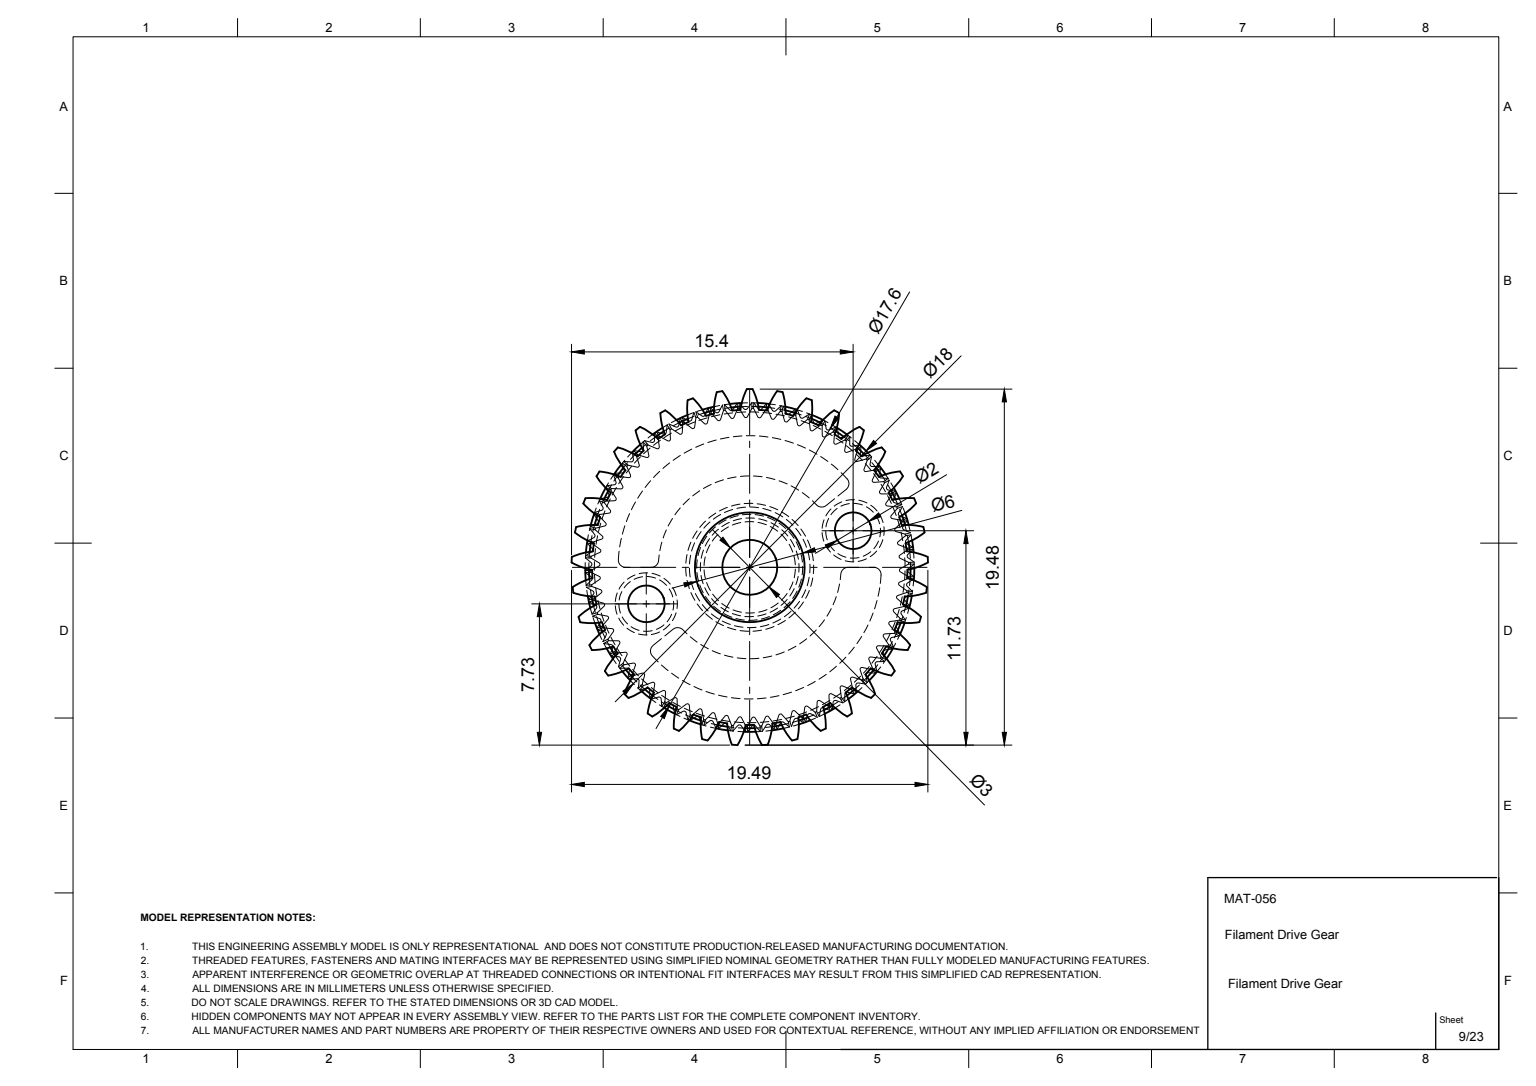
ISO-10303-21;
HEADER;
/* Generated by software containing ST-Developer
 * from STEP Tools, Inc. (www.steptools.com) 
 */

FILE_DESCRIPTION(
/* description */ (''),
/* implementation_level */ '2;1');

FILE_NAME(
/* name */ 'Filament Drive Gear.step',
/* time_stamp */ '2026-10-28T16:47:13+01:00',
/* author */ (''),
/* organization */ (''),
/* preprocessor_version */ 'ST-DEVELOPER v20.2',
/* originating_system */ 'Autodesk Translation Framework v15.17.0.0',
/* authorisation */ '');

FILE_SCHEMA (('AUTOMOTIVE_DESIGN { 1 0 10303 214 3 1 1 }'));
ENDSEC;

DATA;
#10=MECHANICAL_DESIGN_GEOMETRIC_PRESENTATION_REPRESENTATION('',(#4574,#4575),#459242);
#1698=TOROIDAL_SURFACE('',#97244,10.516666667,1.816666667);
#1699=TOROIDAL_SURFACE('',#97247,10.516666667,1.816666667);
#1700=TOROIDAL_SURFACE('',#97250,10.516666667,1.816666667);
#1701=TOROIDAL_SURFACE('',#97253,10.516666667,1.816666667);
#1702=TOROIDAL_SURFACE('',#97256,10.516666667,1.816666667);
#1703=TOROIDAL_SURFACE('',#97259,10.516666667,1.816666667);
#1704=TOROIDAL_SURFACE('',#97262,10.516666667,1.816666667);
#1705=TOROIDAL_SURFACE('',#97265,10.516666667,1.816666667);
#1706=TOROIDAL_SURFACE('',#97268,10.516666667,1.816666667);
#1707=TOROIDAL_SURFACE('',#97271,10.516666667,1.816666667);
#1708=TOROIDAL_SURFACE('',#97274,10.516666667,1.816666667);
#1709=TOROIDAL_SURFACE('',#97277,10.516666667,1.816666667);
#1710=TOROIDAL_SURFACE('',#97280,10.516666667,1.816666667);
#1711=TOROIDAL_SURFACE('',#97283,10.516666667,1.816666667);
#1712=TOROIDAL_SURFACE('',#97286,10.516666667,1.816666667);
#1713=TOROIDAL_SURFACE('',#97289,10.516666667,1.816666667);
#1714=TOROIDAL_SURFACE('',#97292,10.516666667,1.816666667);
#1715=TOROIDAL_SURFACE('',#97295,10.516666667,1.816666667);
#1716=TOROIDAL_SURFACE('',#97298,10.516666667,1.816666667);
#1717=TOROIDAL_SURFACE('',#97301,10.516666667,1.816666667);
#1718=TOROIDAL_SURFACE('',#97304,10.516666667,1.816666667);
#1719=TOROIDAL_SURFACE('',#97307,10.516666667,1.816666667);
#1720=TOROIDAL_SURFACE('',#97310,10.516666667,1.816666667);
#1721=TOROIDAL_SURFACE('',#97313,10.516666667,1.816666667);
#1722=TOROIDAL_SURFACE('',#97316,10.516666667,1.816666667);
#1723=TOROIDAL_SURFACE('',#97319,10.516666667,1.816666667);
#1724=TOROIDAL_SURFACE('',#97322,10.516666667,1.816666667);
#1725=TOROIDAL_SURFACE('',#97325,10.516666667,1.816666667);
#1726=TOROIDAL_SURFACE('',#97328,10.516666667,1.816666667);
#1727=TOROIDAL_SURFACE('',#97331,10.516666667,1.816666667);
#1728=TOROIDAL_SURFACE('',#97334,10.516666667,1.816666667);
#1729=TOROIDAL_SURFACE('',#97337,10.516666667,1.816666667);
#1730=TOROIDAL_SURFACE('',#97340,10.516666667,1.816666667);
#1731=TOROIDAL_SURFACE('',#97343,10.516666667,1.816666667);
#1732=TOROIDAL_SURFACE('',#97346,10.516666667,1.816666667);
#1733=TOROIDAL_SURFACE('',#97349,10.516666667,1.816666667);
#1734=TOROIDAL_SURFACE('',#97352,10.516666667,1.816666667);
#1735=TOROIDAL_SURFACE('',#97355,10.516666667,1.816666667);
#1736=TOROIDAL_SURFACE('',#97358,10.516666667,1.816666667);
#1737=TOROIDAL_SURFACE('',#97361,10.516666667,1.816666667);
#1738=TOROIDAL_SURFACE('',#97364,10.516666667,1.816666667);
#1739=TOROIDAL_SURFACE('',#97367,10.516666667,1.816666667);
#1740=TOROIDAL_SURFACE('',#97370,10.516666667,1.816666667);
#1741=TOROIDAL_SURFACE('',#97373,10.516666667,1.816666667);
#1742=TOROIDAL_SURFACE('',#97376,10.516666667,1.816666667);
#1743=TOROIDAL_SURFACE('',#97379,10.516666667,1.816666667);
#1744=TOROIDAL_SURFACE('',#97382,10.516666667,1.816666667);
#1745=TOROIDAL_SURFACE('',#97385,10.516666667,1.816666667);
#1746=TOROIDAL_SURFACE('',#97388,10.516666667,1.816666667);
#1747=TOROIDAL_SURFACE('',#97391,10.516666667,1.816666667);
#1748=TOROIDAL_SURFACE('',#97394,10.516666667,1.816666667);
#1749=TOROIDAL_SURFACE('',#97397,10.516666667,1.816666667);
#1750=TOROIDAL_SURFACE('',#97400,10.516666667,1.816666667);
#1751=TOROIDAL_SURFACE('',#97403,10.516666667,1.816666667);
#1752=TOROIDAL_SURFACE('',#97406,10.516666667,1.816666667);
#1753=TOROIDAL_SURFACE('',#97409,10.516666667,1.816666667);
#1754=TOROIDAL_SURFACE('',#97412,10.516666667,1.816666667);
#1755=TOROIDAL_SURFACE('',#97415,10.516666667,1.816666667);
#1756=TOROIDAL_SURFACE('',#97418,10.516666667,1.816666667);
#1757=TOROIDAL_SURFACE('',#97421,10.516666667,1.816666667);
#1758=TOROIDAL_SURFACE('',#97424,10.516666667,1.816666667);
#1759=TOROIDAL_SURFACE('',#97427,10.516666667,1.816666667);
#1760=TOROIDAL_SURFACE('',#97430,10.516666667,1.816666667);
#1761=TOROIDAL_SURFACE('',#97433,10.516666667,1.816666667);
#1762=TOROIDAL_SURFACE('',#97436,10.516666667,1.816666667);
#1763=TOROIDAL_SURFACE('',#97439,10.516666667,1.816666667);
#1764=TOROIDAL_SURFACE('',#97442,10.516666667,1.816666667);
#1765=TOROIDAL_SURFACE('',#97445,10.516666667,1.816666667);
#1766=TOROIDAL_SURFACE('',#97448,10.516666667,1.816666667);
#1767=TOROIDAL_SURFACE('',#97451,10.516666667,1.816666667);
#1768=TOROIDAL_SURFACE('',#97496,2.222884449,0.1);
#1769=TOROIDAL_SURFACE('',#97501,2.222884449,0.1);
#1770=TOROIDAL_SURFACE('',#97506,2.222884449,0.1);
#1771=TOROIDAL_SURFACE('',#97511,2.222884449,0.1);
#1772=TOROIDAL_SURFACE('',#97516,2.222884449,0.1);
#1773=TOROIDAL_SURFACE('',#97521,2.222884449,0.1);
#1774=TOROIDAL_SURFACE('',#97526,2.222884449,0.1);
#1775=TOROIDAL_SURFACE('',#97531,2.222884449,0.1);
#1776=TOROIDAL_SURFACE('',#97536,2.222884449,0.1);
#1777=TOROIDAL_SURFACE('',#97541,2.222884449,0.1);
#1778=TOROIDAL_SURFACE('',#97546,2.222884449,0.1);
#1779=TOROIDAL_SURFACE('',#97551,2.222884449,0.1);
#1780=TOROIDAL_SURFACE('',#97556,2.222884449,0.1);
#1781=TOROIDAL_SURFACE('',#97561,2.222884449,0.1);
#1782=TOROIDAL_SURFACE('',#97566,2.222884449,0.1);
#1783=TOROIDAL_SURFACE('',#97571,2.222884449,0.1);
#1784=TOROIDAL_SURFACE('',#97576,2.222884449,0.1);
#1785=TOROIDAL_SURFACE('',#97581,2.222884449,0.1);
#1786=TOROIDAL_SURFACE('',#97586,2.222884449,0.1);
#1787=TOROIDAL_SURFACE('',#97591,2.222884449,0.1);
#1788=TOROIDAL_SURFACE('',#97596,2.222884449,0.1);
#1789=TOROIDAL_SURFACE('',#97601,2.222884449,0.1);
#1790=TOROIDAL_SURFACE('',#97606,2.222884449,0.1);
#1791=TOROIDAL_SURFACE('',#97611,2.222884449,0.1);
#1792=TOROIDAL_SURFACE('',#97616,2.222884449,0.1);
#1793=TOROIDAL_SURFACE('',#97621,2.222884449,0.1);
#1794=TOROIDAL_SURFACE('',#97626,2.222884449,0.1);
#1795=TOROIDAL_SURFACE('',#97631,2.222884449,0.1);
#1796=TOROIDAL_SURFACE('',#97636,2.222884449,0.1);
#1797=TOROIDAL_SURFACE('',#97641,2.222884449,0.1);
#1798=TOROIDAL_SURFACE('',#97646,2.222884449,0.1);
#1799=TOROIDAL_SURFACE('',#97651,2.222884449,0.1);
#1800=TOROIDAL_SURFACE('',#97656,2.222884449,0.1);
#1801=TOROIDAL_SURFACE('',#97661,2.222884449,0.1);
#1802=TOROIDAL_SURFACE('',#97666,2.222884449,0.1);
#1803=TOROIDAL_SURFACE('',#97671,2.222884449,0.1);
#1804=TOROIDAL_SURFACE('',#97676,2.222884449,0.1);
#1805=TOROIDAL_SURFACE('',#97681,2.222884449,0.1);
#1806=TOROIDAL_SURFACE('',#97686,2.222884449,0.1);
#1807=TOROIDAL_SURFACE('',#97691,2.222884449,0.1);
#1808=TOROIDAL_SURFACE('',#97696,2.222884449,0.1);
#1809=TOROIDAL_SURFACE('',#97701,2.222884449,0.1);
#1810=TOROIDAL_SURFACE('',#97706,2.222884449,0.1);
#1811=TOROIDAL_SURFACE('',#97711,2.222884449,0.1);
#1812=TOROIDAL_SURFACE('',#97716,2.222884449,0.1);
#1813=TOROIDAL_SURFACE('',#97721,2.222884449,0.1);
#1814=TOROIDAL_SURFACE('',#97726,2.222884449,0.1);
#1815=TOROIDAL_SURFACE('',#97731,2.222884449,0.1);
#1816=TOROIDAL_SURFACE('',#97736,2.222884449,0.1);
#1817=TOROIDAL_SURFACE('',#97741,2.222884449,0.1);
#1818=TOROIDAL_SURFACE('',#97746,2.222884449,0.1);
#1819=TOROIDAL_SURFACE('',#97751,2.222884449,0.1);
#1820=TOROIDAL_SURFACE('',#97756,2.222884449,0.1);
#1821=TOROIDAL_SURFACE('',#97761,2.222884449,0.1);
#1822=TOROIDAL_SURFACE('',#97766,2.222884449,0.1);
#1823=TOROIDAL_SURFACE('',#97771,2.222884449,0.1);
#1824=TOROIDAL_SURFACE('',#97776,2.222884449,0.1);
#1825=TOROIDAL_SURFACE('',#97781,2.222884449,0.1);
#1826=TOROIDAL_SURFACE('',#97786,2.222884449,0.1);
#1827=TOROIDAL_SURFACE('',#97791,2.222884449,0.1);
#1828=TOROIDAL_SURFACE('',#97796,2.222884449,0.1);
#1829=TOROIDAL_SURFACE('',#97801,2.222884449,0.1);
#1830=TOROIDAL_SURFACE('',#97806,2.222884449,0.1);
#1831=TOROIDAL_SURFACE('',#97811,2.222884449,0.1);
#1832=TOROIDAL_SURFACE('',#97816,2.222884449,0.1);
#1833=TOROIDAL_SURFACE('',#97821,2.222884449,0.1);
#1834=TOROIDAL_SURFACE('',#97826,2.222884449,0.1);
#1835=TOROIDAL_SURFACE('',#97831,2.222884449,0.1);
#1836=TOROIDAL_SURFACE('',#97836,2.222884449,0.1);
#1837=TOROIDAL_SURFACE('',#97841,2.222884449,0.1);
#1838=TOROIDAL_SURFACE('',#97850,1.6,0.1);
#1839=TOROIDAL_SURFACE('',#97854,1.6,0.1);
#1840=TOROIDAL_SURFACE('',#97858,1.7,0.2);
#1841=TOROIDAL_SURFACE('',#97863,1.7,0.2);
#1842=TOROIDAL_SURFACE('',#97867,2.8,0.2);
#1843=TOROIDAL_SURFACE('',#97872,0.6,0.2);
#1844=TOROIDAL_SURFACE('',#97877,0.6,0.2);
#1845=TOROIDAL_SURFACE('',#97882,3.9,0.4);
#1846=TOROIDAL_SURFACE('',#97887,1.1,0.4);
#1847=TOROIDAL_SURFACE('',#97892,1.1,0.4);
#1848=TOROIDAL_SURFACE('',#98404,0.6,0.2);
#1849=TOROIDAL_SURFACE('',#98409,7.4,0.2);
#1850=TOROIDAL_SURFACE('',#98410,0.6,0.2);
#1851=TOROIDAL_SURFACE('',#98412,4.8,0.2);
#1852=TOROIDAL_SURFACE('',#98416,0.6,0.2);
#1853=TOROIDAL_SURFACE('',#98417,0.6,0.2);
#1854=TOROIDAL_SURFACE('',#98420,4.8,0.2);
#1855=TOROIDAL_SURFACE('',#98423,0.6,0.2);
#1856=TOROIDAL_SURFACE('',#98427,7.4,0.2);
#1857=TOROIDAL_SURFACE('',#98429,0.6,0.2);
#4411=SHAPE_REPRESENTATION_RELATIONSHIP('SRR','None',#459336,#4432);
#4432=ADVANCED_BREP_SHAPE_REPRESENTATION('',(#4454,#4455),#459225);
#4454=MANIFOLD_SOLID_BREP('Feed gear',#94632);
#4455=MANIFOLD_SOLID_BREP('Drive gear',#94633);
#4574=STYLED_ITEM('',(#459512),#4454);
#4575=STYLED_ITEM('',(#459512),#4455);
#4712=CONICAL_SURFACE('',#97454,2.9,0.78539816250733);
#4713=CONICAL_SURFACE('',#97458,1.5,0.78539816250733);
#4714=CONICAL_SURFACE('',#97462,1.5,0.78539816250733);
#4715=CONICAL_SURFACE('',#97466,8.8,0.78539816250733);
#4716=CONICAL_SURFACE('',#97470,1.7,0.78539816250733);
#4717=CONICAL_SURFACE('',#97473,1.7,0.78539816250733);
#4718=CONICAL_SURFACE('',#97476,3.3,0.78539816250733);
#4719=CONICAL_SURFACE('',#97480,2.5,0.78539816250733);
#4720=CONICAL_SURFACE('',#97485,9.,0.78539816250733);
#4721=CONICAL_SURFACE('',#97494,2.272884449,1.04719754999232);
#4722=CONICAL_SURFACE('',#97498,1.816666667,1.04719754999232);
#4723=CONICAL_SURFACE('',#97499,2.272884449,1.04719754999232);
#4724=CONICAL_SURFACE('',#97503,1.816666667,1.04719754999232);
#4725=CONICAL_SURFACE('',#97504,2.272884449,1.04719754999232);
#4726=CONICAL_SURFACE('',#97508,1.816666667,1.04719754999232);
#4727=CONICAL_SURFACE('',#97509,2.272884449,1.04719754999232);
#4728=CONICAL_SURFACE('',#97513,1.816666667,1.04719754999232);
#4729=CONICAL_SURFACE('',#97514,2.272884449,1.04719754999232);
#4730=CONICAL_SURFACE('',#97518,1.816666667,1.04719754999232);
#4731=CONICAL_SURFACE('',#97519,2.272884449,1.04719754999232);
#4732=CONICAL_SURFACE('',#97523,1.816666667,1.04719754999232);
#4733=CONICAL_SURFACE('',#97524,2.272884449,1.04719754999232);
#4734=CONICAL_SURFACE('',#97528,1.816666667,1.04719754999232);
#4735=CONICAL_SURFACE('',#97529,2.272884449,1.04719754999232);
#4736=CONICAL_SURFACE('',#97533,1.816666667,1.04719754999232);
#4737=CONICAL_SURFACE('',#97534,2.272884449,1.04719754999232);
#4738=CONICAL_SURFACE('',#97538,1.816666667,1.04719754999232);
#4739=CONICAL_SURFACE('',#97539,2.272884449,1.04719754999232);
#4740=CONICAL_SURFACE('',#97543,1.816666667,1.04719754999232);
#4741=CONICAL_SURFACE('',#97544,2.272884449,1.04719754999232);
#4742=CONICAL_SURFACE('',#97548,1.816666667,1.04719754999232);
#4743=CONICAL_SURFACE('',#97549,2.272884449,1.04719754999232);
#4744=CONICAL_SURFACE('',#97553,1.816666667,1.04719754999232);
#4745=CONICAL_SURFACE('',#97554,2.272884449,1.04719754999232);
#4746=CONICAL_SURFACE('',#97558,1.816666667,1.04719754999232);
#4747=CONICAL_SURFACE('',#97559,2.272884449,1.04719754999232);
#4748=CONICAL_SURFACE('',#97563,1.816666667,1.04719754999232);
#4749=CONICAL_SURFACE('',#97564,2.272884449,1.04719754999232);
#4750=CONICAL_SURFACE('',#97568,1.816666667,1.04719754999232);
#4751=CONICAL_SURFACE('',#97569,2.272884449,1.04719754999232);
#4752=CONICAL_SURFACE('',#97573,1.816666667,1.04719754999232);
#4753=CONICAL_SURFACE('',#97574,2.272884449,1.04719754999232);
#4754=CONICAL_SURFACE('',#97578,1.816666667,1.04719754999232);
#4755=CONICAL_SURFACE('',#97579,2.272884449,1.04719754999232);
#4756=CONICAL_SURFACE('',#97583,1.816666667,1.04719754999232);
#4757=CONICAL_SURFACE('',#97584,2.272884449,1.04719754999232);
#4758=CONICAL_SURFACE('',#97588,1.816666667,1.04719754999232);
#4759=CONICAL_SURFACE('',#97589,2.272884449,1.04719754999232);
#4760=CONICAL_SURFACE('',#97593,1.816666667,1.04719754999232);
#4761=CONICAL_SURFACE('',#97594,2.272884449,1.04719754999232);
#4762=CONICAL_SURFACE('',#97598,1.816666667,1.04719754999232);
#4763=CONICAL_SURFACE('',#97599,2.272884449,1.04719754999232);
#4764=CONICAL_SURFACE('',#97603,1.816666667,1.04719754999232);
#4765=CONICAL_SURFACE('',#97604,2.272884449,1.04719754999232);
#4766=CONICAL_SURFACE('',#97608,1.816666667,1.04719754999232);
#4767=CONICAL_SURFACE('',#97609,2.272884449,1.04719754999232);
#4768=CONICAL_SURFACE('',#97613,1.816666667,1.04719754999232);
#4769=CONICAL_SURFACE('',#97614,2.272884449,1.04719754999232);
#4770=CONICAL_SURFACE('',#97618,1.816666667,1.04719754999232);
#4771=CONICAL_SURFACE('',#97619,2.272884449,1.04719754999232);
#4772=CONICAL_SURFACE('',#97623,1.816666667,1.04719754999232);
#4773=CONICAL_SURFACE('',#97624,2.272884449,1.04719754999232);
#4774=CONICAL_SURFACE('',#97628,1.816666667,1.04719754999232);
#4775=CONICAL_SURFACE('',#97629,2.272884449,1.04719754999232);
#4776=CONICAL_SURFACE('',#97633,1.816666667,1.04719754999232);
#4777=CONICAL_SURFACE('',#97634,2.272884449,1.04719754999232);
#4778=CONICAL_SURFACE('',#97638,1.816666667,1.04719754999232);
#4779=CONICAL_SURFACE('',#97639,2.272884449,1.04719754999232);
#4780=CONICAL_SURFACE('',#97643,1.816666667,1.04719754999232);
#4781=CONICAL_SURFACE('',#97644,2.272884449,1.04719754999232);
#4782=CONICAL_SURFACE('',#97648,1.816666667,1.04719754999232);
#4783=CONICAL_SURFACE('',#97649,2.272884449,1.04719754999232);
#4784=CONICAL_SURFACE('',#97653,1.816666667,1.04719754999232);
#4785=CONICAL_SURFACE('',#97654,2.272884449,1.04719754999232);
#4786=CONICAL_SURFACE('',#97658,1.816666667,1.04719754999232);
#4787=CONICAL_SURFACE('',#97659,2.272884449,1.04719754999232);
#4788=CONICAL_SURFACE('',#97663,1.816666667,1.04719754999232);
#4789=CONICAL_SURFACE('',#97664,2.272884449,1.04719754999232);
#4790=CONICAL_SURFACE('',#97668,1.816666667,1.04719754999232);
#4791=CONICAL_SURFACE('',#97669,2.272884449,1.04719754999232);
#4792=CONICAL_SURFACE('',#97673,1.816666667,1.04719754999232);
#4793=CONICAL_SURFACE('',#97674,2.272884449,1.04719754999232);
#4794=CONICAL_SURFACE('',#97678,1.816666667,1.04719754999232);
#4795=CONICAL_SURFACE('',#97679,2.272884449,1.04719754999232);
#4796=CONICAL_SURFACE('',#97683,1.816666667,1.04719754999232);
#4797=CONICAL_SURFACE('',#97684,2.272884449,1.04719754999232);
#4798=CONICAL_SURFACE('',#97688,1.816666667,1.04719754999232);
#4799=CONICAL_SURFACE('',#97689,2.272884449,1.04719754999232);
#4800=CONICAL_SURFACE('',#97693,1.816666667,1.04719754999232);
#4801=CONICAL_SURFACE('',#97694,2.272884449,1.04719754999232);
#4802=CONICAL_SURFACE('',#97698,1.816666667,1.04719754999232);
#4803=CONICAL_SURFACE('',#97699,2.272884449,1.04719754999232);
#4804=CONICAL_SURFACE('',#97703,1.816666667,1.04719754999232);
#4805=CONICAL_SURFACE('',#97704,2.272884449,1.04719754999232);
#4806=CONICAL_SURFACE('',#97708,1.816666667,1.04719754999232);
#4807=CONICAL_SURFACE('',#97709,2.272884449,1.04719754999232);
#4808=CONICAL_SURFACE('',#97713,1.816666667,1.04719754999232);
#4809=CONICAL_SURFACE('',#97714,2.272884449,1.04719754999232);
#4810=CONICAL_SURFACE('',#97718,1.816666667,1.04719754999232);
#4811=CONICAL_SURFACE('',#97719,2.272884449,1.04719754999232);
#4812=CONICAL_SURFACE('',#97723,1.816666667,1.04719754999232);
#4813=CONICAL_SURFACE('',#97724,2.272884449,1.04719754999232);
#4814=CONICAL_SURFACE('',#97728,1.816666667,1.04719754999232);
#4815=CONICAL_SURFACE('',#97729,2.272884449,1.04719754999232);
#4816=CONICAL_SURFACE('',#97733,1.816666667,1.04719754999232);
#4817=CONICAL_SURFACE('',#97734,2.272884449,1.04719754999232);
#4818=CONICAL_SURFACE('',#97738,1.816666667,1.04719754999232);
#4819=CONICAL_SURFACE('',#97739,2.272884449,1.04719754999232);
#4820=CONICAL_SURFACE('',#97743,1.816666667,1.04719754999232);
#4821=CONICAL_SURFACE('',#97744,2.272884449,1.04719754999232);
#4822=CONICAL_SURFACE('',#97748,1.816666667,1.04719754999232);
#4823=CONICAL_SURFACE('',#97749,2.272884449,1.04719754999232);
#4824=CONICAL_SURFACE('',#97753,1.816666667,1.04719754999232);
#4825=CONICAL_SURFACE('',#97754,2.272884449,1.04719754999232);
#4826=CONICAL_SURFACE('',#97758,1.816666667,1.04719754999232);
#4827=CONICAL_SURFACE('',#97759,2.272884449,1.04719754999232);
#4828=CONICAL_SURFACE('',#97763,1.816666667,1.04719754999232);
#4829=CONICAL_SURFACE('',#97764,2.272884449,1.04719754999232);
#4830=CONICAL_SURFACE('',#97768,1.816666667,1.04719754999232);
#4831=CONICAL_SURFACE('',#97769,2.272884449,1.04719754999232);
#4832=CONICAL_SURFACE('',#97773,1.816666667,1.04719754999232);
#4833=CONICAL_SURFACE('',#97774,2.272884449,1.04719754999232);
#4834=CONICAL_SURFACE('',#97778,1.816666667,1.04719754999232);
#4835=CONICAL_SURFACE('',#97779,2.272884449,1.04719754999232);
#4836=CONICAL_SURFACE('',#97783,1.816666667,1.04719754999232);
#4837=CONICAL_SURFACE('',#97784,2.272884449,1.04719754999232);
#4838=CONICAL_SURFACE('',#97788,1.816666667,1.04719754999232);
#4839=CONICAL_SURFACE('',#97789,2.272884449,1.04719754999232);
#4840=CONICAL_SURFACE('',#97793,1.816666667,1.04719754999232);
#4841=CONICAL_SURFACE('',#97794,2.272884449,1.04719754999232);
#4842=CONICAL_SURFACE('',#97798,1.816666667,1.04719754999232);
#4843=CONICAL_SURFACE('',#97799,2.272884449,1.04719754999232);
#4844=CONICAL_SURFACE('',#97803,1.816666667,1.04719754999232);
#4845=CONICAL_SURFACE('',#97804,2.272884449,1.04719754999232);
#4846=CONICAL_SURFACE('',#97808,1.816666667,1.04719754999232);
#4847=CONICAL_SURFACE('',#97809,2.272884449,1.04719754999232);
#4848=CONICAL_SURFACE('',#97813,1.816666667,1.04719754999232);
#4849=CONICAL_SURFACE('',#97814,2.272884449,1.04719754999232);
#4850=CONICAL_SURFACE('',#97818,1.816666667,1.04719754999232);
#4851=CONICAL_SURFACE('',#97819,2.272884449,1.04719754999232);
#4852=CONICAL_SURFACE('',#97823,1.816666667,1.04719754999232);
#4853=CONICAL_SURFACE('',#97824,2.272884449,1.04719754999232);
#4854=CONICAL_SURFACE('',#97828,1.816666667,1.04719754999232);
#4855=CONICAL_SURFACE('',#97829,2.272884449,1.04719754999232);
#4856=CONICAL_SURFACE('',#97833,1.816666667,1.04719754999232);
#4857=CONICAL_SURFACE('',#97834,2.272884449,1.04719754999232);
#4858=CONICAL_SURFACE('',#97838,1.816666667,1.04719754999232);
#4859=CONICAL_SURFACE('',#97839,2.272884449,1.04719754999232);
#4860=CONICAL_SURFACE('',#97843,1.816666667,1.04719754999232);
#5170=FACE_BOUND('',#13390,.T.);
#5171=FACE_BOUND('',#13392,.T.);
#5172=FACE_BOUND('',#13393,.T.);
#5173=FACE_BOUND('',#13394,.T.);
#5174=FACE_BOUND('',#13396,.T.);
#5175=FACE_BOUND('',#13397,.T.);
#5176=FACE_BOUND('',#13398,.T.);
#5177=FACE_BOUND('',#13633,.T.);
#5178=FACE_BOUND('',#13634,.T.);
#5179=FACE_BOUND('',#13635,.T.);
#5180=FACE_BOUND('',#13636,.T.);
#5181=FACE_BOUND('',#13637,.T.);
#5182=FACE_BOUND('',#13675,.T.);
#5183=FACE_BOUND('',#13676,.T.);
#5184=FACE_BOUND('',#13677,.T.);
#5185=FACE_BOUND('',#13787,.T.);
#5186=FACE_BOUND('',#13791,.T.);
#5591=PLANE('',#97491);
#5592=PLANE('',#97492);
#5593=PLANE('',#97493);
#5594=PLANE('',#97922);
#5595=PLANE('',#98149);
#5596=PLANE('',#98366);
#5597=PLANE('',#98367);
#5598=PLANE('',#98368);
#5599=PLANE('',#98369);
#5600=PLANE('',#98370);
#5601=PLANE('',#98380);
#5602=PLANE('',#98386);
#5603=PLANE('',#98390);
#5604=PLANE('',#98396);
#5605=PLANE('',#98403);
#5606=PLANE('',#98430);
#5607=PLANE('',#98431);
#7440=FACE_OUTER_BOUND('',#13305,.T.);
#7441=FACE_OUTER_BOUND('',#13306,.T.);
#7442=FACE_OUTER_BOUND('',#13307,.T.);
#7443=FACE_OUTER_BOUND('',#13308,.T.);
#7444=FACE_OUTER_BOUND('',#13309,.T.);
#7445=FACE_OUTER_BOUND('',#13310,.T.);
#7446=FACE_OUTER_BOUND('',#13311,.T.);
#7447=FACE_OUTER_BOUND('',#13312,.T.);
#7448=FACE_OUTER_BOUND('',#13313,.T.);
#7449=FACE_OUTER_BOUND('',#13314,.T.);
#7450=FACE_OUTER_BOUND('',#13315,.T.);
#7451=FACE_OUTER_BOUND('',#13316,.T.);
#7452=FACE_OUTER_BOUND('',#13317,.T.);
#7453=FACE_OUTER_BOUND('',#13318,.T.);
#7454=FACE_OUTER_BOUND('',#13319,.T.);
#7455=FACE_OUTER_BOUND('',#13320,.T.);
#7456=FACE_OUTER_BOUND('',#13321,.T.);
#7457=FACE_OUTER_BOUND('',#13322,.T.);
#7458=FACE_OUTER_BOUND('',#13323,.T.);
#7459=FACE_OUTER_BOUND('',#13324,.T.);
#7460=FACE_OUTER_BOUND('',#13325,.T.);
#7461=FACE_OUTER_BOUND('',#13326,.T.);
#7462=FACE_OUTER_BOUND('',#13327,.T.);
#7463=FACE_OUTER_BOUND('',#13328,.T.);
#7464=FACE_OUTER_BOUND('',#13329,.T.);
#7465=FACE_OUTER_BOUND('',#13330,.T.);
#7466=FACE_OUTER_BOUND('',#13331,.T.);
#7467=FACE_OUTER_BOUND('',#13332,.T.);
#7468=FACE_OUTER_BOUND('',#13333,.T.);
#7469=FACE_OUTER_BOUND('',#13334,.T.);
#7470=FACE_OUTER_BOUND('',#13335,.T.);
#7471=FACE_OUTER_BOUND('',#13336,.T.);
#7472=FACE_OUTER_BOUND('',#13337,.T.);
#7473=FACE_OUTER_BOUND('',#13338,.T.);
#7474=FACE_OUTER_BOUND('',#13339,.T.);
#7475=FACE_OUTER_BOUND('',#13340,.T.);
#7476=FACE_OUTER_BOUND('',#13341,.T.);
#7477=FACE_OUTER_BOUND('',#13342,.T.);
#7478=FACE_OUTER_BOUND('',#13343,.T.);
#7479=FACE_OUTER_BOUND('',#13344,.T.);
#7480=FACE_OUTER_BOUND('',#13345,.T.);
#7481=FACE_OUTER_BOUND('',#13346,.T.);
#7482=FACE_OUTER_BOUND('',#13347,.T.);
#7483=FACE_OUTER_BOUND('',#13348,.T.);
#7484=FACE_OUTER_BOUND('',#13349,.T.);
#7485=FACE_OUTER_BOUND('',#13350,.T.);
#7486=FACE_OUTER_BOUND('',#13351,.T.);
#7487=FACE_OUTER_BOUND('',#13352,.T.);
#7488=FACE_OUTER_BOUND('',#13353,.T.);
#7489=FACE_OUTER_BOUND('',#13354,.T.);
#7490=FACE_OUTER_BOUND('',#13355,.T.);
#7491=FACE_OUTER_BOUND('',#13356,.T.);
#7492=FACE_OUTER_BOUND('',#13357,.T.);
#7493=FACE_OUTER_BOUND('',#13358,.T.);
#7494=FACE_OUTER_BOUND('',#13359,.T.);
#7495=FACE_OUTER_BOUND('',#13360,.T.);
#7496=FACE_OUTER_BOUND('',#13361,.T.);
#7497=FACE_OUTER_BOUND('',#13362,.T.);
#7498=FACE_OUTER_BOUND('',#13363,.T.);
#7499=FACE_OUTER_BOUND('',#13364,.T.);
#7500=FACE_OUTER_BOUND('',#13365,.T.);
#7501=FACE_OUTER_BOUND('',#13366,.T.);
#7502=FACE_OUTER_BOUND('',#13367,.T.);
#7503=FACE_OUTER_BOUND('',#13368,.T.);
#7504=FACE_OUTER_BOUND('',#13369,.T.);
#7505=FACE_OUTER_BOUND('',#13370,.T.);
#7506=FACE_OUTER_BOUND('',#13371,.T.);
#7507=FACE_OUTER_BOUND('',#13372,.T.);
#7508=FACE_OUTER_BOUND('',#13373,.T.);
#7509=FACE_OUTER_BOUND('',#13374,.T.);
#7510=FACE_OUTER_BOUND('',#13375,.T.);
#7511=FACE_OUTER_BOUND('',#13376,.T.);
#7512=FACE_OUTER_BOUND('',#13377,.T.);
#7513=FACE_OUTER_BOUND('',#13378,.T.);
#7514=FACE_OUTER_BOUND('',#13379,.T.);
#7515=FACE_OUTER_BOUND('',#13380,.T.);
#7516=FACE_OUTER_BOUND('',#13381,.T.);
#7517=FACE_OUTER_BOUND('',#13382,.T.);
#7518=FACE_OUTER_BOUND('',#13383,.T.);
#7519=FACE_OUTER_BOUND('',#13384,.T.);
#7520=FACE_OUTER_BOUND('',#13385,.T.);
#7521=FACE_OUTER_BOUND('',#13386,.T.);
#7522=FACE_OUTER_BOUND('',#13387,.T.);
#7523=FACE_OUTER_BOUND('',#13388,.T.);
#7524=FACE_OUTER_BOUND('',#13389,.T.);
#7525=FACE_OUTER_BOUND('',#13391,.T.);
#7526=FACE_OUTER_BOUND('',#13395,.T.);
#7527=FACE_OUTER_BOUND('',#13399,.T.);
#7528=FACE_OUTER_BOUND('',#13400,.T.);
#7529=FACE_OUTER_BOUND('',#13401,.T.);
#7530=FACE_OUTER_BOUND('',#13402,.T.);
#7531=FACE_OUTER_BOUND('',#13403,.T.);
#7532=FACE_OUTER_BOUND('',#13404,.T.);
#7533=FACE_OUTER_BOUND('',#13405,.T.);
#7534=FACE_OUTER_BOUND('',#13406,.T.);
#7535=FACE_OUTER_BOUND('',#13407,.T.);
#7536=FACE_OUTER_BOUND('',#13408,.T.);
#7537=FACE_OUTER_BOUND('',#13409,.T.);
#7538=FACE_OUTER_BOUND('',#13410,.T.);
#7539=FACE_OUTER_BOUND('',#13411,.T.);
#7540=FACE_OUTER_BOUND('',#13412,.T.);
#7541=FACE_OUTER_BOUND('',#13413,.T.);
#7542=FACE_OUTER_BOUND('',#13414,.T.);
#7543=FACE_OUTER_BOUND('',#13415,.T.);
#7544=FACE_OUTER_BOUND('',#13416,.T.);
#7545=FACE_OUTER_BOUND('',#13417,.T.);
#7546=FACE_OUTER_BOUND('',#13418,.T.);
#7547=FACE_OUTER_BOUND('',#13419,.T.);
#7548=FACE_OUTER_BOUND('',#13420,.T.);
#7549=FACE_OUTER_BOUND('',#13421,.T.);
#7550=FACE_OUTER_BOUND('',#13422,.T.);
#7551=FACE_OUTER_BOUND('',#13423,.T.);
#7552=FACE_OUTER_BOUND('',#13424,.T.);
#7553=FACE_OUTER_BOUND('',#13425,.T.);
#7554=FACE_OUTER_BOUND('',#13426,.T.);
#7555=FACE_OUTER_BOUND('',#13427,.T.);
#7556=FACE_OUTER_BOUND('',#13428,.T.);
#7557=FACE_OUTER_BOUND('',#13429,.T.);
#7558=FACE_OUTER_BOUND('',#13430,.T.);
#7559=FACE_OUTER_BOUND('',#13431,.T.);
#7560=FACE_OUTER_BOUND('',#13432,.T.);
#7561=FACE_OUTER_BOUND('',#13433,.T.);
#7562=FACE_OUTER_BOUND('',#13434,.T.);
#7563=FACE_OUTER_BOUND('',#13435,.T.);
#7564=FACE_OUTER_BOUND('',#13436,.T.);
#7565=FACE_OUTER_BOUND('',#13437,.T.);
#7566=FACE_OUTER_BOUND('',#13438,.T.);
#7567=FACE_OUTER_BOUND('',#13439,.T.);
#7568=FACE_OUTER_BOUND('',#13440,.T.);
#7569=FACE_OUTER_BOUND('',#13441,.T.);
#7570=FACE_OUTER_BOUND('',#13442,.T.);
#7571=FACE_OUTER_BOUND('',#13443,.T.);
#7572=FACE_OUTER_BOUND('',#13444,.T.);
#7573=FACE_OUTER_BOUND('',#13445,.T.);
#7574=FACE_OUTER_BOUND('',#13446,.T.);
#7575=FACE_OUTER_BOUND('',#13447,.T.);
#7576=FACE_OUTER_BOUND('',#13448,.T.);
#7577=FACE_OUTER_BOUND('',#13449,.T.);
#7578=FACE_OUTER_BOUND('',#13450,.T.);
#7579=FACE_OUTER_BOUND('',#13451,.T.);
#7580=FACE_OUTER_BOUND('',#13452,.T.);
#7581=FACE_OUTER_BOUND('',#13453,.T.);
#7582=FACE_OUTER_BOUND('',#13454,.T.);
#7583=FACE_OUTER_BOUND('',#13455,.T.);
#7584=FACE_OUTER_BOUND('',#13456,.T.);
#7585=FACE_OUTER_BOUND('',#13457,.T.);
#7586=FACE_OUTER_BOUND('',#13458,.T.);
#7587=FACE_OUTER_BOUND('',#13459,.T.);
#7588=FACE_OUTER_BOUND('',#13460,.T.);
#7589=FACE_OUTER_BOUND('',#13461,.T.);
#7590=FACE_OUTER_BOUND('',#13462,.T.);
#7591=FACE_OUTER_BOUND('',#13463,.T.);
#7592=FACE_OUTER_BOUND('',#13464,.T.);
#7593=FACE_OUTER_BOUND('',#13465,.T.);
#7594=FACE_OUTER_BOUND('',#13466,.T.);
#7595=FACE_OUTER_BOUND('',#13467,.T.);
#7596=FACE_OUTER_BOUND('',#13468,.T.);
#7597=FACE_OUTER_BOUND('',#13469,.T.);
#7598=FACE_OUTER_BOUND('',#13470,.T.);
#7599=FACE_OUTER_BOUND('',#13471,.T.);
#7600=FACE_OUTER_BOUND('',#13472,.T.);
#7601=FACE_OUTER_BOUND('',#13473,.T.);
#7602=FACE_OUTER_BOUND('',#13474,.T.);
#7603=FACE_OUTER_BOUND('',#13475,.T.);
#7604=FACE_OUTER_BOUND('',#13476,.T.);
#7605=FACE_OUTER_BOUND('',#13477,.T.);
#7606=FACE_OUTER_BOUND('',#13478,.T.);
#7607=FACE_OUTER_BOUND('',#13479,.T.);
#7608=FACE_OUTER_BOUND('',#13480,.T.);
#7609=FACE_OUTER_BOUND('',#13481,.T.);
#7610=FACE_OUTER_BOUND('',#13482,.T.);
#7611=FACE_OUTER_BOUND('',#13483,.T.);
#7612=FACE_OUTER_BOUND('',#13484,.T.);
#7613=FACE_OUTER_BOUND('',#13485,.T.);
#7614=FACE_OUTER_BOUND('',#13486,.T.);
#7615=FACE_OUTER_BOUND('',#13487,.T.);
#7616=FACE_OUTER_BOUND('',#13488,.T.);
#7617=FACE_OUTER_BOUND('',#13489,.T.);
#7618=FACE_OUTER_BOUND('',#13490,.T.);
#7619=FACE_OUTER_BOUND('',#13491,.T.);
#7620=FACE_OUTER_BOUND('',#13492,.T.);
#7621=FACE_OUTER_BOUND('',#13493,.T.);
#7622=FACE_OUTER_BOUND('',#13494,.T.);
#7623=FACE_OUTER_BOUND('',#13495,.T.);
#7624=FACE_OUTER_BOUND('',#13496,.T.);
#7625=FACE_OUTER_BOUND('',#13497,.T.);
#7626=FACE_OUTER_BOUND('',#13498,.T.);
#7627=FACE_OUTER_BOUND('',#13499,.T.);
#7628=FACE_OUTER_BOUND('',#13500,.T.);
#7629=FACE_OUTER_BOUND('',#13501,.T.);
#7630=FACE_OUTER_BOUND('',#13502,.T.);
#7631=FACE_OUTER_BOUND('',#13503,.T.);
#7632=FACE_OUTER_BOUND('',#13504,.T.);
#7633=FACE_OUTER_BOUND('',#13505,.T.);
#7634=FACE_OUTER_BOUND('',#13506,.T.);
#7635=FACE_OUTER_BOUND('',#13507,.T.);
#7636=FACE_OUTER_BOUND('',#13508,.T.);
#7637=FACE_OUTER_BOUND('',#13509,.T.);
#7638=FACE_OUTER_BOUND('',#13510,.T.);
#7639=FACE_OUTER_BOUND('',#13511,.T.);
#7640=FACE_OUTER_BOUND('',#13512,.T.);
#7641=FACE_OUTER_BOUND('',#13513,.T.);
#7642=FACE_OUTER_BOUND('',#13514,.T.);
#7643=FACE_OUTER_BOUND('',#13515,.T.);
#7644=FACE_OUTER_BOUND('',#13516,.T.);
#7645=FACE_OUTER_BOUND('',#13517,.T.);
#7646=FACE_OUTER_BOUND('',#13518,.T.);
#7647=FACE_OUTER_BOUND('',#13519,.T.);
#7648=FACE_OUTER_BOUND('',#13520,.T.);
#7649=FACE_OUTER_BOUND('',#13521,.T.);
#7650=FACE_OUTER_BOUND('',#13522,.T.);
#7651=FACE_OUTER_BOUND('',#13523,.T.);
#7652=FACE_OUTER_BOUND('',#13524,.T.);
#7653=FACE_OUTER_BOUND('',#13525,.T.);
#7654=FACE_OUTER_BOUND('',#13526,.T.);
#7655=FACE_OUTER_BOUND('',#13527,.T.);
#7656=FACE_OUTER_BOUND('',#13528,.T.);
#7657=FACE_OUTER_BOUND('',#13529,.T.);
#7658=FACE_OUTER_BOUND('',#13530,.T.);
#7659=FACE_OUTER_BOUND('',#13531,.T.);
#7660=FACE_OUTER_BOUND('',#13532,.T.);
#7661=FACE_OUTER_BOUND('',#13533,.T.);
#7662=FACE_OUTER_BOUND('',#13534,.T.);
#7663=FACE_OUTER_BOUND('',#13535,.T.);
#7664=FACE_OUTER_BOUND('',#13536,.T.);
#7665=FACE_OUTER_BOUND('',#13537,.T.);
#7666=FACE_OUTER_BOUND('',#13538,.T.);
#7667=FACE_OUTER_BOUND('',#13539,.T.);
#7668=FACE_OUTER_BOUND('',#13540,.T.);
#7669=FACE_OUTER_BOUND('',#13541,.T.);
#7670=FACE_OUTER_BOUND('',#13542,.T.);
#7671=FACE_OUTER_BOUND('',#13543,.T.);
#7672=FACE_OUTER_BOUND('',#13544,.T.);
#7673=FACE_OUTER_BOUND('',#13545,.T.);
#7674=FACE_OUTER_BOUND('',#13546,.T.);
#7675=FACE_OUTER_BOUND('',#13547,.T.);
#7676=FACE_OUTER_BOUND('',#13548,.T.);
#7677=FACE_OUTER_BOUND('',#13549,.T.);
#7678=FACE_OUTER_BOUND('',#13550,.T.);
#7679=FACE_OUTER_BOUND('',#13551,.T.);
#7680=FACE_OUTER_BOUND('',#13552,.T.);
#7681=FACE_OUTER_BOUND('',#13553,.T.);
#7682=FACE_OUTER_BOUND('',#13554,.T.);
#7683=FACE_OUTER_BOUND('',#13555,.T.);
#7684=FACE_OUTER_BOUND('',#13556,.T.);
#7685=FACE_OUTER_BOUND('',#13557,.T.);
#7686=FACE_OUTER_BOUND('',#13558,.T.);
#7687=FACE_OUTER_BOUND('',#13559,.T.);
#7688=FACE_OUTER_BOUND('',#13560,.T.);
#7689=FACE_OUTER_BOUND('',#13561,.T.);
#7690=FACE_OUTER_BOUND('',#13562,.T.);
#7691=FACE_OUTER_BOUND('',#13563,.T.);
#7692=FACE_OUTER_BOUND('',#13564,.T.);
#7693=FACE_OUTER_BOUND('',#13565,.T.);
#7694=FACE_OUTER_BOUND('',#13566,.T.);
#7695=FACE_OUTER_BOUND('',#13567,.T.);
#7696=FACE_OUTER_BOUND('',#13568,.T.);
#7697=FACE_OUTER_BOUND('',#13569,.T.);
#7698=FACE_OUTER_BOUND('',#13570,.T.);
#7699=FACE_OUTER_BOUND('',#13571,.T.);
#7700=FACE_OUTER_BOUND('',#13572,.T.);
#7701=FACE_OUTER_BOUND('',#13573,.T.);
#7702=FACE_OUTER_BOUND('',#13574,.T.);
#7703=FACE_OUTER_BOUND('',#13575,.T.);
#7704=FACE_OUTER_BOUND('',#13576,.T.);
#7705=FACE_OUTER_BOUND('',#13577,.T.);
#7706=FACE_OUTER_BOUND('',#13578,.T.);
#7707=FACE_OUTER_BOUND('',#13579,.T.);
#7708=FACE_OUTER_BOUND('',#13580,.T.);
#7709=FACE_OUTER_BOUND('',#13581,.T.);
#7710=FACE_OUTER_BOUND('',#13582,.T.);
#7711=FACE_OUTER_BOUND('',#13583,.T.);
#7712=FACE_OUTER_BOUND('',#13584,.T.);
#7713=FACE_OUTER_BOUND('',#13585,.T.);
#7714=FACE_OUTER_BOUND('',#13586,.T.);
#7715=FACE_OUTER_BOUND('',#13587,.T.);
#7716=FACE_OUTER_BOUND('',#13588,.T.);
#7717=FACE_OUTER_BOUND('',#13589,.T.);
#7718=FACE_OUTER_BOUND('',#13590,.T.);
#7719=FACE_OUTER_BOUND('',#13591,.T.);
#7720=FACE_OUTER_BOUND('',#13592,.T.);
#7721=FACE_OUTER_BOUND('',#13593,.T.);
#7722=FACE_OUTER_BOUND('',#13594,.T.);
#7723=FACE_OUTER_BOUND('',#13595,.T.);
#7724=FACE_OUTER_BOUND('',#13596,.T.);
#7725=FACE_OUTER_BOUND('',#13597,.T.);
#7726=FACE_OUTER_BOUND('',#13598,.T.);
#7727=FACE_OUTER_BOUND('',#13599,.T.);
#7728=FACE_OUTER_BOUND('',#13600,.T.);
#7729=FACE_OUTER_BOUND('',#13601,.T.);
#7730=FACE_OUTER_BOUND('',#13602,.T.);
#7731=FACE_OUTER_BOUND('',#13603,.T.);
#7732=FACE_OUTER_BOUND('',#13604,.T.);
#7733=FACE_OUTER_BOUND('',#13605,.T.);
#7734=FACE_OUTER_BOUND('',#13606,.T.);
#7735=FACE_OUTER_BOUND('',#13607,.T.);
#7736=FACE_OUTER_BOUND('',#13608,.T.);
#7737=FACE_OUTER_BOUND('',#13609,.T.);
#7738=FACE_OUTER_BOUND('',#13610,.T.);
#7739=FACE_OUTER_BOUND('',#13611,.T.);
#7740=FACE_OUTER_BOUND('',#13612,.T.);
#7741=FACE_OUTER_BOUND('',#13613,.T.);
#7742=FACE_OUTER_BOUND('',#13614,.T.);
#7743=FACE_OUTER_BOUND('',#13615,.T.);
#7744=FACE_OUTER_BOUND('',#13616,.T.);
#7745=FACE_OUTER_BOUND('',#13617,.T.);
#7746=FACE_OUTER_BOUND('',#13618,.T.);
#7747=FACE_OUTER_BOUND('',#13619,.T.);
#7748=FACE_OUTER_BOUND('',#13620,.T.);
#7749=FACE_OUTER_BOUND('',#13621,.T.);
#7750=FACE_OUTER_BOUND('',#13622,.T.);
#7751=FACE_OUTER_BOUND('',#13623,.T.);
#7752=FACE_OUTER_BOUND('',#13624,.T.);
#7753=FACE_OUTER_BOUND('',#13625,.T.);
#7754=FACE_OUTER_BOUND('',#13626,.T.);
#7755=FACE_OUTER_BOUND('',#13627,.T.);
#7756=FACE_OUTER_BOUND('',#13628,.T.);
#7757=FACE_OUTER_BOUND('',#13629,.T.);
#7758=FACE_OUTER_BOUND('',#13630,.T.);
#7759=FACE_OUTER_BOUND('',#13631,.T.);
#7760=FACE_OUTER_BOUND('',#13632,.T.);
#7761=FACE_OUTER_BOUND('',#13638,.T.);
#7762=FACE_OUTER_BOUND('',#13639,.T.);
#7763=FACE_OUTER_BOUND('',#13640,.T.);
#7764=FACE_OUTER_BOUND('',#13641,.T.);
#7765=FACE_OUTER_BOUND('',#13642,.T.);
#7766=FACE_OUTER_BOUND('',#13643,.T.);
#7767=FACE_OUTER_BOUND('',#13644,.T.);
#7768=FACE_OUTER_BOUND('',#13645,.T.);
#7769=FACE_OUTER_BOUND('',#13646,.T.);
#7770=FACE_OUTER_BOUND('',#13647,.T.);
#7771=FACE_OUTER_BOUND('',#13648,.T.);
#7772=FACE_OUTER_BOUND('',#13649,.T.);
#7773=FACE_OUTER_BOUND('',#13650,.T.);
#7774=FACE_OUTER_BOUND('',#13651,.T.);
#7775=FACE_OUTER_BOUND('',#13652,.T.);
#7776=FACE_OUTER_BOUND('',#13653,.T.);
#7777=FACE_OUTER_BOUND('',#13654,.T.);
#7778=FACE_OUTER_BOUND('',#13655,.T.);
#7779=FACE_OUTER_BOUND('',#13656,.T.);
#7780=FACE_OUTER_BOUND('',#13657,.T.);
#7781=FACE_OUTER_BOUND('',#13658,.T.);
#7782=FACE_OUTER_BOUND('',#13659,.T.);
#7783=FACE_OUTER_BOUND('',#13660,.T.);
#7784=FACE_OUTER_BOUND('',#13661,.T.);
#7785=FACE_OUTER_BOUND('',#13662,.T.);
#7786=FACE_OUTER_BOUND('',#13663,.T.);
#7787=FACE_OUTER_BOUND('',#13664,.T.);
#7788=FACE_OUTER_BOUND('',#13665,.T.);
#7789=FACE_OUTER_BOUND('',#13666,.T.);
#7790=FACE_OUTER_BOUND('',#13667,.T.);
#7791=FACE_OUTER_BOUND('',#13668,.T.);
#7792=FACE_OUTER_BOUND('',#13669,.T.);
#7793=FACE_OUTER_BOUND('',#13670,.T.);
#7794=FACE_OUTER_BOUND('',#13671,.T.);
#7795=FACE_OUTER_BOUND('',#13672,.T.);
#7796=FACE_OUTER_BOUND('',#13673,.T.);
#7797=FACE_OUTER_BOUND('',#13674,.T.);
#7798=FACE_OUTER_BOUND('',#13678,.T.);
#7799=FACE_OUTER_BOUND('',#13679,.T.);
#7800=FACE_OUTER_BOUND('',#13680,.T.);
#7801=FACE_OUTER_BOUND('',#13681,.T.);
#7802=FACE_OUTER_BOUND('',#13682,.T.);
#7803=FACE_OUTER_BOUND('',#13683,.T.);
#7804=FACE_OUTER_BOUND('',#13684,.T.);
#7805=FACE_OUTER_BOUND('',#13685,.T.);
#7806=FACE_OUTER_BOUND('',#13686,.T.);
#7807=FACE_OUTER_BOUND('',#13687,.T.);
#7808=FACE_OUTER_BOUND('',#13688,.T.);
#7809=FACE_OUTER_BOUND('',#13689,.T.);
#7810=FACE_OUTER_BOUND('',#13690,.T.);
#7811=FACE_OUTER_BOUND('',#13691,.T.);
#7812=FACE_OUTER_BOUND('',#13692,.T.);
#7813=FACE_OUTER_BOUND('',#13693,.T.);
#7814=FACE_OUTER_BOUND('',#13694,.T.);
#7815=FACE_OUTER_BOUND('',#13695,.T.);
#7816=FACE_OUTER_BOUND('',#13696,.T.);
#7817=FACE_OUTER_BOUND('',#13697,.T.);
#7818=FACE_OUTER_BOUND('',#13698,.T.);
#7819=FACE_OUTER_BOUND('',#13699,.T.);
#7820=FACE_OUTER_BOUND('',#13700,.T.);
#7821=FACE_OUTER_BOUND('',#13701,.T.);
#7822=FACE_OUTER_BOUND('',#13702,.T.);
#7823=FACE_OUTER_BOUND('',#13703,.T.);
#7824=FACE_OUTER_BOUND('',#13704,.T.);
#7825=FACE_OUTER_BOUND('',#13705,.T.);
#7826=FACE_OUTER_BOUND('',#13706,.T.);
#7827=FACE_OUTER_BOUND('',#13707,.T.);
#7828=FACE_OUTER_BOUND('',#13708,.T.);
#7829=FACE_OUTER_BOUND('',#13709,.T.);
#7830=FACE_OUTER_BOUND('',#13710,.T.);
#7831=FACE_OUTER_BOUND('',#13711,.T.);
#7832=FACE_OUTER_BOUND('',#13712,.T.);
#7833=FACE_OUTER_BOUND('',#13713,.T.);
#7834=FACE_OUTER_BOUND('',#13714,.T.);
#7835=FACE_OUTER_BOUND('',#13715,.T.);
#7836=FACE_OUTER_BOUND('',#13716,.T.);
#7837=FACE_OUTER_BOUND('',#13717,.T.);
#7838=FACE_OUTER_BOUND('',#13718,.T.);
#7839=FACE_OUTER_BOUND('',#13719,.T.);
#7840=FACE_OUTER_BOUND('',#13720,.T.);
#7841=FACE_OUTER_BOUND('',#13721,.T.);
#7842=FACE_OUTER_BOUND('',#13722,.T.);
#7843=FACE_OUTER_BOUND('',#13723,.T.);
#7844=FACE_OUTER_BOUND('',#13724,.T.);
#7845=FACE_OUTER_BOUND('',#13725,.T.);
#7846=FACE_OUTER_BOUND('',#13726,.T.);
#7847=FACE_OUTER_BOUND('',#13727,.T.);
#7848=FACE_OUTER_BOUND('',#13728,.T.);
#7849=FACE_OUTER_BOUND('',#13729,.T.);
#7850=FACE_OUTER_BOUND('',#13730,.T.);
#7851=FACE_OUTER_BOUND('',#13731,.T.);
#7852=FACE_OUTER_BOUND('',#13732,.T.);
#7853=FACE_OUTER_BOUND('',#13733,.T.);
#7854=FACE_OUTER_BOUND('',#13734,.T.);
#7855=FACE_OUTER_BOUND('',#13735,.T.);
#7856=FACE_OUTER_BOUND('',#13736,.T.);
#7857=FACE_OUTER_BOUND('',#13737,.T.);
#7858=FACE_OUTER_BOUND('',#13738,.T.);
#7859=FACE_OUTER_BOUND('',#13739,.T.);
#7860=FACE_OUTER_BOUND('',#13740,.T.);
#7861=FACE_OUTER_BOUND('',#13741,.T.);
#7862=FACE_OUTER_BOUND('',#13742,.T.);
#7863=FACE_OUTER_BOUND('',#13743,.T.);
#7864=FACE_OUTER_BOUND('',#13744,.T.);
#7865=FACE_OUTER_BOUND('',#13745,.T.);
#7866=FACE_OUTER_BOUND('',#13746,.T.);
#7867=FACE_OUTER_BOUND('',#13747,.T.);
#7868=FACE_OUTER_BOUND('',#13748,.T.);
#7869=FACE_OUTER_BOUND('',#13749,.T.);
#7870=FACE_OUTER_BOUND('',#13750,.T.);
#7871=FACE_OUTER_BOUND('',#13751,.T.);
#7872=FACE_OUTER_BOUND('',#13752,.T.);
#7873=FACE_OUTER_BOUND('',#13753,.T.);
#7874=FACE_OUTER_BOUND('',#13754,.T.);
#7875=FACE_OUTER_BOUND('',#13755,.T.);
#7876=FACE_OUTER_BOUND('',#13756,.T.);
#7877=FACE_OUTER_BOUND('',#13757,.T.);
#7878=FACE_OUTER_BOUND('',#13758,.T.);
#7879=FACE_OUTER_BOUND('',#13759,.T.);
#7880=FACE_OUTER_BOUND('',#13760,.T.);
#7881=FACE_OUTER_BOUND('',#13761,.T.);
#7882=FACE_OUTER_BOUND('',#13762,.T.);
#7883=FACE_OUTER_BOUND('',#13763,.T.);
#7884=FACE_OUTER_BOUND('',#13764,.T.);
#7885=FACE_OUTER_BOUND('',#13765,.T.);
#7886=FACE_OUTER_BOUND('',#13766,.T.);
#7887=FACE_OUTER_BOUND('',#13767,.T.);
#7888=FACE_OUTER_BOUND('',#13768,.T.);
#7889=FACE_OUTER_BOUND('',#13769,.T.);
#7890=FACE_OUTER_BOUND('',#13770,.T.);
#7891=FACE_OUTER_BOUND('',#13771,.T.);
#7892=FACE_OUTER_BOUND('',#13772,.T.);
#7893=FACE_OUTER_BOUND('',#13773,.T.);
#7894=FACE_OUTER_BOUND('',#13774,.T.);
#7895=FACE_OUTER_BOUND('',#13775,.T.);
#7896=FACE_OUTER_BOUND('',#13776,.T.);
#7897=FACE_OUTER_BOUND('',#13777,.T.);
#7898=FACE_OUTER_BOUND('',#13778,.T.);
#7899=FACE_OUTER_BOUND('',#13779,.T.);
#7900=FACE_OUTER_BOUND('',#13780,.T.);
#7901=FACE_OUTER_BOUND('',#13781,.T.);
#7902=FACE_OUTER_BOUND('',#13782,.T.);
#7903=FACE_OUTER_BOUND('',#13783,.T.);
#7904=FACE_OUTER_BOUND('',#13784,.T.);
#7905=FACE_OUTER_BOUND('',#13785,.T.);
#7906=FACE_OUTER_BOUND('',#13786,.T.);
#7907=FACE_OUTER_BOUND('',#13788,.T.);
#7908=FACE_OUTER_BOUND('',#13789,.T.);
#7909=FACE_OUTER_BOUND('',#13790,.T.);
#7910=FACE_OUTER_BOUND('',#13792,.T.);
#7911=FACE_OUTER_BOUND('',#13793,.T.);
#7912=FACE_OUTER_BOUND('',#13794,.T.);
#7913=FACE_OUTER_BOUND('',#13795,.T.);
#7914=FACE_OUTER_BOUND('',#13796,.T.);
#7915=FACE_OUTER_BOUND('',#13797,.T.);
#7916=FACE_OUTER_BOUND('',#13798,.T.);
#7917=FACE_OUTER_BOUND('',#13799,.T.);
#7918=FACE_OUTER_BOUND('',#13800,.T.);
#7919=FACE_OUTER_BOUND('',#13801,.T.);
#7920=FACE_OUTER_BOUND('',#13802,.T.);
#7921=FACE_OUTER_BOUND('',#13803,.T.);
#7922=FACE_OUTER_BOUND('',#13804,.T.);
#7923=FACE_OUTER_BOUND('',#13805,.T.);
#7924=FACE_OUTER_BOUND('',#13806,.T.);
#7925=FACE_OUTER_BOUND('',#13807,.T.);
#7926=FACE_OUTER_BOUND('',#13808,.T.);
#7927=FACE_OUTER_BOUND('',#13809,.T.);
#7928=FACE_OUTER_BOUND('',#13810,.T.);
#7929=FACE_OUTER_BOUND('',#13811,.T.);
#7930=FACE_OUTER_BOUND('',#13812,.T.);
#7931=FACE_OUTER_BOUND('',#13813,.T.);
#7932=FACE_OUTER_BOUND('',#13814,.T.);
#7933=FACE_OUTER_BOUND('',#13815,.T.);
#7934=FACE_OUTER_BOUND('',#13816,.T.);
#7935=FACE_OUTER_BOUND('',#13817,.T.);
#7936=FACE_OUTER_BOUND('',#13818,.T.);
#7937=FACE_OUTER_BOUND('',#13819,.T.);
#7938=FACE_OUTER_BOUND('',#13820,.T.);
#7939=FACE_OUTER_BOUND('',#13821,.T.);
#7940=FACE_OUTER_BOUND('',#13822,.T.);
#7941=FACE_OUTER_BOUND('',#13823,.T.);
#13305=EDGE_LOOP('',(#63834,#63835,#63836,#63837));
#13306=EDGE_LOOP('',(#63838,#63839,#63840,#63841));
#13307=EDGE_LOOP('',(#63842,#63843,#63844,#63845));
#13308=EDGE_LOOP('',(#63846,#63847,#63848,#63849));
#13309=EDGE_LOOP('',(#63850,#63851,#63852,#63853));
#13310=EDGE_LOOP('',(#63854,#63855,#63856,#63857));
#13311=EDGE_LOOP('',(#63858,#63859,#63860,#63861));
#13312=EDGE_LOOP('',(#63862,#63863,#63864,#63865));
#13313=EDGE_LOOP('',(#63866,#63867,#63868,#63869));
#13314=EDGE_LOOP('',(#63870,#63871,#63872,#63873));
#13315=EDGE_LOOP('',(#63874,#63875,#63876,#63877));
#13316=EDGE_LOOP('',(#63878,#63879,#63880,#63881));
#13317=EDGE_LOOP('',(#63882,#63883,#63884,#63885));
#13318=EDGE_LOOP('',(#63886,#63887,#63888,#63889));
#13319=EDGE_LOOP('',(#63890,#63891,#63892,#63893));
#13320=EDGE_LOOP('',(#63894,#63895,#63896,#63897));
#13321=EDGE_LOOP('',(#63898,#63899,#63900,#63901));
#13322=EDGE_LOOP('',(#63902,#63903,#63904,#63905));
#13323=EDGE_LOOP('',(#63906,#63907,#63908,#63909));
#13324=EDGE_LOOP('',(#63910,#63911,#63912,#63913));
#13325=EDGE_LOOP('',(#63914,#63915,#63916,#63917));
#13326=EDGE_LOOP('',(#63918,#63919,#63920,#63921));
#13327=EDGE_LOOP('',(#63922,#63923,#63924,#63925));
#13328=EDGE_LOOP('',(#63926,#63927,#63928,#63929));
#13329=EDGE_LOOP('',(#63930,#63931,#63932,#63933));
#13330=EDGE_LOOP('',(#63934,#63935,#63936,#63937));
#13331=EDGE_LOOP('',(#63938,#63939,#63940,#63941));
#13332=EDGE_LOOP('',(#63942,#63943,#63944,#63945));
#13333=EDGE_LOOP('',(#63946,#63947,#63948,#63949));
#13334=EDGE_LOOP('',(#63950,#63951,#63952,#63953));
#13335=EDGE_LOOP('',(#63954,#63955,#63956,#63957));
#13336=EDGE_LOOP('',(#63958,#63959,#63960,#63961));
#13337=EDGE_LOOP('',(#63962,#63963,#63964,#63965));
#13338=EDGE_LOOP('',(#63966,#63967,#63968,#63969));
#13339=EDGE_LOOP('',(#63970,#63971,#63972,#63973));
#13340=EDGE_LOOP('',(#63974,#63975,#63976,#63977));
#13341=EDGE_LOOP('',(#63978,#63979,#63980,#63981));
#13342=EDGE_LOOP('',(#63982,#63983,#63984,#63985));
#13343=EDGE_LOOP('',(#63986,#63987,#63988,#63989));
#13344=EDGE_LOOP('',(#63990,#63991,#63992,#63993));
#13345=EDGE_LOOP('',(#63994,#63995,#63996,#63997));
#13346=EDGE_LOOP('',(#63998,#63999,#64000,#64001));
#13347=EDGE_LOOP('',(#64002,#64003,#64004,#64005));
#13348=EDGE_LOOP('',(#64006,#64007,#64008,#64009));
#13349=EDGE_LOOP('',(#64010,#64011,#64012,#64013));
#13350=EDGE_LOOP('',(#64014,#64015,#64016,#64017));
#13351=EDGE_LOOP('',(#64018,#64019,#64020,#64021));
#13352=EDGE_LOOP('',(#64022,#64023,#64024,#64025));
#13353=EDGE_LOOP('',(#64026,#64027,#64028,#64029));
#13354=EDGE_LOOP('',(#64030,#64031,#64032,#64033));
#13355=EDGE_LOOP('',(#64034,#64035,#64036,#64037));
#13356=EDGE_LOOP('',(#64038,#64039,#64040,#64041));
#13357=EDGE_LOOP('',(#64042,#64043,#64044,#64045));
#13358=EDGE_LOOP('',(#64046,#64047,#64048,#64049));
#13359=EDGE_LOOP('',(#64050,#64051,#64052,#64053));
#13360=EDGE_LOOP('',(#64054,#64055,#64056,#64057));
#13361=EDGE_LOOP('',(#64058,#64059,#64060,#64061));
#13362=EDGE_LOOP('',(#64062,#64063,#64064,#64065));
#13363=EDGE_LOOP('',(#64066,#64067,#64068,#64069));
#13364=EDGE_LOOP('',(#64070,#64071,#64072,#64073));
#13365=EDGE_LOOP('',(#64074,#64075,#64076,#64077));
#13366=EDGE_LOOP('',(#64078,#64079,#64080,#64081));
#13367=EDGE_LOOP('',(#64082,#64083,#64084,#64085));
#13368=EDGE_LOOP('',(#64086,#64087,#64088,#64089));
#13369=EDGE_LOOP('',(#64090,#64091,#64092,#64093));
#13370=EDGE_LOOP('',(#64094,#64095,#64096,#64097));
#13371=EDGE_LOOP('',(#64098,#64099,#64100,#64101));
#13372=EDGE_LOOP('',(#64102,#64103,#64104,#64105));
#13373=EDGE_LOOP('',(#64106,#64107,#64108,#64109));
#13374=EDGE_LOOP('',(#64110,#64111,#64112,#64113));
#13375=EDGE_LOOP('',(#64114,#64115,#64116,#64117,#64118));
#13376=EDGE_LOOP('',(#64119,#64120,#64121,#64122,#64123));
#13377=EDGE_LOOP('',(#64124,#64125,#64126,#64127,#64128));
#13378=EDGE_LOOP('',(#64129,#64130,#64131,#64132,#64133));
#13379=EDGE_LOOP('',(#64134,#64135,#64136,#64137));
#13380=EDGE_LOOP('',(#64138,#64139,#64140,#64141));
#13381=EDGE_LOOP('',(#64142,#64143,#64144,#64145,#64146));
#13382=EDGE_LOOP('',(#64147,#64148,#64149,#64150));
#13383=EDGE_LOOP('',(#64151,#64152,#64153,#64154,#64155));
#13384=EDGE_LOOP('',(#64156,#64157,#64158,#64159,#64160));
#13385=EDGE_LOOP('',(#64161,#64162,#64163,#64164,#64165,#64166,#64167,#64168,
#64169,#64170,#64171,#64172,#64173,#64174,#64175,#64176,#64177,#64178,#64179,
#64180,#64181,#64182,#64183,#64184,#64185,#64186,#64187,#64188,#64189,#64190,
#64191,#64192,#64193,#64194,#64195,#64196,#64197,#64198,#64199,#64200,#64201,
#64202,#64203,#64204,#64205,#64206,#64207,#64208,#64209,#64210,#64211,#64212,
#64213,#64214,#64215,#64216,#64217,#64218,#64219,#64220,#64221,#64222,#64223,
#64224,#64225,#64226,#64227,#64228,#64229,#64230,#64231,#64232,#64233,#64234,
#64235,#64236,#64237,#64238,#64239,#64240,#64241,#64242,#64243,#64244,#64245,
#64246,#64247,#64248,#64249,#64250,#64251,#64252,#64253,#64254,#64255,#64256,
#64257,#64258,#64259,#64260,#64261,#64262,#64263,#64264,#64265,#64266,#64267,
#64268,#64269,#64270,#64271,#64272,#64273,#64274,#64275,#64276,#64277,#64278,
#64279,#64280,#64281,#64282,#64283,#64284,#64285,#64286,#64287,#64288,#64289,
#64290,#64291,#64292,#64293,#64294,#64295,#64296,#64297,#64298,#64299,#64300,
#64301,#64302,#64303,#64304,#64305,#64306,#64307,#64308,#64309,#64310,#64311,
#64312,#64313,#64314,#64315,#64316,#64317,#64318,#64319,#64320,#64321,#64322,
#64323,#64324,#64325,#64326,#64327,#64328,#64329,#64330,#64331,#64332,#64333,
#64334,#64335,#64336,#64337,#64338,#64339,#64340,#64341,#64342,#64343,#64344,
#64345,#64346,#64347,#64348,#64349,#64350,#64351,#64352,#64353,#64354,#64355,
#64356,#64357,#64358,#64359,#64360,#64361,#64362,#64363,#64364,#64365,#64366,
#64367,#64368,#64369,#64370,#64371,#64372,#64373,#64374,#64375,#64376,#64377,
#64378,#64379,#64380,#64381,#64382,#64383,#64384,#64385,#64386,#64387,#64388,
#64389,#64390,#64391,#64392,#64393,#64394,#64395,#64396,#64397,#64398,#64399,
#64400,#64401,#64402,#64403,#64404,#64405,#64406,#64407,#64408,#64409,#64410,
#64411,#64412,#64413,#64414,#64415,#64416,#64417,#64418,#64419,#64420,#64421,
#64422,#64423,#64424,#64425,#64426,#64427,#64428,#64429,#64430,#64431,#64432,
#64433,#64434,#64435,#64436,#64437,#64438,#64439,#64440,#64441,#64442,#64443,
#64444));
#13386=EDGE_LOOP('',(#64445,#64446,#64447,#64448,#64449,#64450,#64451,#64452,
#64453,#64454,#64455,#64456,#64457,#64458,#64459,#64460,#64461,#64462,#64463,
#64464,#64465,#64466,#64467,#64468,#64469,#64470,#64471,#64472,#64473,#64474,
#64475,#64476,#64477,#64478,#64479,#64480,#64481,#64482,#64483,#64484,#64485,
#64486,#64487,#64488,#64489,#64490,#64491,#64492,#64493,#64494,#64495,#64496,
#64497,#64498,#64499,#64500,#64501,#64502,#64503,#64504,#64505,#64506,#64507,
#64508,#64509,#64510,#64511,#64512,#64513,#64514,#64515,#64516,#64517,#64518,
#64519,#64520,#64521,#64522,#64523,#64524,#64525,#64526,#64527,#64528,#64529,
#64530,#64531,#64532,#64533,#64534,#64535,#64536,#64537,#64538,#64539,#64540,
#64541,#64542,#64543,#64544,#64545,#64546,#64547,#64548,#64549,#64550,#64551,
#64552,#64553,#64554,#64555,#64556,#64557,#64558,#64559,#64560,#64561,#64562,
#64563,#64564,#64565,#64566,#64567,#64568,#64569,#64570,#64571,#64572,#64573,
#64574,#64575,#64576,#64577,#64578,#64579,#64580,#64581,#64582,#64583,#64584,
#64585,#64586,#64587,#64588,#64589,#64590,#64591,#64592,#64593,#64594,#64595,
#64596,#64597,#64598,#64599,#64600,#64601,#64602,#64603,#64604,#64605,#64606,
#64607,#64608,#64609,#64610,#64611,#64612,#64613,#64614,#64615,#64616,#64617,
#64618,#64619,#64620,#64621,#64622,#64623,#64624,#64625,#64626,#64627,#64628,
#64629,#64630,#64631,#64632,#64633,#64634,#64635,#64636,#64637,#64638,#64639,
#64640,#64641,#64642,#64643,#64644,#64645,#64646,#64647,#64648,#64649,#64650,
#64651,#64652,#64653,#64654,#64655,#64656,#64657,#64658,#64659,#64660,#64661,
#64662,#64663,#64664,#64665,#64666,#64667,#64668,#64669,#64670,#64671,#64672,
#64673,#64674,#64675,#64676,#64677,#64678,#64679,#64680,#64681,#64682,#64683,
#64684,#64685,#64686,#64687,#64688,#64689,#64690,#64691,#64692,#64693,#64694,
#64695,#64696,#64697,#64698,#64699,#64700,#64701,#64702,#64703,#64704,#64705,
#64706,#64707,#64708,#64709,#64710,#64711,#64712,#64713,#64714,#64715,#64716,
#64717,#64718,#64719,#64720,#64721,#64722,#64723,#64724,#64725,#64726,#64727,
#64728,#64729));
#13387=EDGE_LOOP('',(#64730,#64731,#64732,#64733,#64734));
#13388=EDGE_LOOP('',(#64735,#64736,#64737,#64738,#64739));
#13389=EDGE_LOOP('',(#64740));
#13390=EDGE_LOOP('',(#64741));
#13391=EDGE_LOOP('',(#64742));
#13392=EDGE_LOOP('',(#64743));
#13393=EDGE_LOOP('',(#64744));
#13394=EDGE_LOOP('',(#64745));
#13395=EDGE_LOOP('',(#64746));
#13396=EDGE_LOOP('',(#64747));
#13397=EDGE_LOOP('',(#64748));
#13398=EDGE_LOOP('',(#64749));
#13399=EDGE_LOOP('',(#64750,#64751,#64752,#64753));
#13400=EDGE_LOOP('',(#64754,#64755,#64756,#64757));
#13401=EDGE_LOOP('',(#64758,#64759,#64760,#64761));
#13402=EDGE_LOOP('',(#64762,#64763,#64764,#64765));
#13403=EDGE_LOOP('',(#64766,#64767,#64768,#64769));
#13404=EDGE_LOOP('',(#64770,#64771,#64772,#64773));
#13405=EDGE_LOOP('',(#64774,#64775,#64776,#64777));
#13406=EDGE_LOOP('',(#64778,#64779,#64780,#64781));
#13407=EDGE_LOOP('',(#64782,#64783,#64784,#64785));
#13408=EDGE_LOOP('',(#64786,#64787,#64788,#64789));
#13409=EDGE_LOOP('',(#64790,#64791,#64792,#64793));
#13410=EDGE_LOOP('',(#64794,#64795,#64796,#64797));
#13411=EDGE_LOOP('',(#64798,#64799,#64800,#64801));
#13412=EDGE_LOOP('',(#64802,#64803,#64804,#64805));
#13413=EDGE_LOOP('',(#64806,#64807,#64808,#64809));
#13414=EDGE_LOOP('',(#64810,#64811,#64812,#64813));
#13415=EDGE_LOOP('',(#64814,#64815,#64816,#64817));
#13416=EDGE_LOOP('',(#64818,#64819,#64820,#64821));
#13417=EDGE_LOOP('',(#64822,#64823,#64824,#64825));
#13418=EDGE_LOOP('',(#64826,#64827,#64828,#64829));
#13419=EDGE_LOOP('',(#64830,#64831,#64832,#64833));
#13420=EDGE_LOOP('',(#64834,#64835,#64836,#64837));
#13421=EDGE_LOOP('',(#64838,#64839,#64840,#64841));
#13422=EDGE_LOOP('',(#64842,#64843,#64844,#64845));
#13423=EDGE_LOOP('',(#64846,#64847,#64848,#64849));
#13424=EDGE_LOOP('',(#64850,#64851,#64852,#64853));
#13425=EDGE_LOOP('',(#64854,#64855,#64856,#64857));
#13426=EDGE_LOOP('',(#64858,#64859,#64860,#64861));
#13427=EDGE_LOOP('',(#64862,#64863,#64864,#64865));
#13428=EDGE_LOOP('',(#64866,#64867,#64868,#64869));
#13429=EDGE_LOOP('',(#64870,#64871,#64872,#64873));
#13430=EDGE_LOOP('',(#64874,#64875,#64876,#64877));
#13431=EDGE_LOOP('',(#64878,#64879,#64880,#64881));
#13432=EDGE_LOOP('',(#64882,#64883,#64884,#64885));
#13433=EDGE_LOOP('',(#64886,#64887,#64888,#64889));
#13434=EDGE_LOOP('',(#64890,#64891,#64892,#64893));
#13435=EDGE_LOOP('',(#64894,#64895,#64896,#64897));
#13436=EDGE_LOOP('',(#64898,#64899,#64900,#64901));
#13437=EDGE_LOOP('',(#64902,#64903,#64904,#64905));
#13438=EDGE_LOOP('',(#64906,#64907,#64908,#64909));
#13439=EDGE_LOOP('',(#64910,#64911,#64912,#64913));
#13440=EDGE_LOOP('',(#64914,#64915,#64916,#64917));
#13441=EDGE_LOOP('',(#64918,#64919,#64920,#64921));
#13442=EDGE_LOOP('',(#64922,#64923,#64924,#64925));
#13443=EDGE_LOOP('',(#64926,#64927,#64928,#64929));
#13444=EDGE_LOOP('',(#64930,#64931,#64932,#64933));
#13445=EDGE_LOOP('',(#64934,#64935,#64936,#64937));
#13446=EDGE_LOOP('',(#64938,#64939,#64940,#64941));
#13447=EDGE_LOOP('',(#64942,#64943,#64944,#64945));
#13448=EDGE_LOOP('',(#64946,#64947,#64948,#64949));
#13449=EDGE_LOOP('',(#64950,#64951,#64952,#64953));
#13450=EDGE_LOOP('',(#64954,#64955,#64956,#64957));
#13451=EDGE_LOOP('',(#64958,#64959,#64960,#64961));
#13452=EDGE_LOOP('',(#64962,#64963,#64964,#64965));
#13453=EDGE_LOOP('',(#64966,#64967,#64968,#64969));
#13454=EDGE_LOOP('',(#64970,#64971,#64972,#64973));
#13455=EDGE_LOOP('',(#64974,#64975,#64976,#64977));
#13456=EDGE_LOOP('',(#64978,#64979,#64980,#64981));
#13457=EDGE_LOOP('',(#64982,#64983,#64984,#64985));
#13458=EDGE_LOOP('',(#64986,#64987,#64988,#64989));
#13459=EDGE_LOOP('',(#64990,#64991,#64992,#64993));
#13460=EDGE_LOOP('',(#64994,#64995,#64996,#64997));
#13461=EDGE_LOOP('',(#64998,#64999,#65000,#65001));
#13462=EDGE_LOOP('',(#65002,#65003,#65004,#65005));
#13463=EDGE_LOOP('',(#65006,#65007,#65008,#65009));
#13464=EDGE_LOOP('',(#65010,#65011,#65012,#65013));
#13465=EDGE_LOOP('',(#65014,#65015,#65016,#65017));
#13466=EDGE_LOOP('',(#65018,#65019,#65020,#65021));
#13467=EDGE_LOOP('',(#65022,#65023,#65024,#65025));
#13468=EDGE_LOOP('',(#65026,#65027,#65028,#65029));
#13469=EDGE_LOOP('',(#65030,#65031,#65032,#65033));
#13470=EDGE_LOOP('',(#65034,#65035,#65036,#65037));
#13471=EDGE_LOOP('',(#65038,#65039,#65040,#65041));
#13472=EDGE_LOOP('',(#65042,#65043,#65044,#65045));
#13473=EDGE_LOOP('',(#65046,#65047,#65048,#65049));
#13474=EDGE_LOOP('',(#65050,#65051,#65052,#65053));
#13475=EDGE_LOOP('',(#65054,#65055,#65056,#65057));
#13476=EDGE_LOOP('',(#65058,#65059,#65060,#65061));
#13477=EDGE_LOOP('',(#65062,#65063,#65064,#65065));
#13478=EDGE_LOOP('',(#65066,#65067,#65068,#65069));
#13479=EDGE_LOOP('',(#65070,#65071,#65072,#65073));
#13480=EDGE_LOOP('',(#65074,#65075,#65076,#65077));
#13481=EDGE_LOOP('',(#65078,#65079,#65080,#65081));
#13482=EDGE_LOOP('',(#65082,#65083,#65084,#65085));
#13483=EDGE_LOOP('',(#65086,#65087,#65088,#65089));
#13484=EDGE_LOOP('',(#65090,#65091,#65092,#65093));
#13485=EDGE_LOOP('',(#65094,#65095,#65096,#65097));
#13486=EDGE_LOOP('',(#65098,#65099,#65100,#65101));
#13487=EDGE_LOOP('',(#65102,#65103,#65104,#65105));
#13488=EDGE_LOOP('',(#65106,#65107,#65108,#65109));
#13489=EDGE_LOOP('',(#65110,#65111,#65112,#65113));
#13490=EDGE_LOOP('',(#65114,#65115,#65116,#65117));
#13491=EDGE_LOOP('',(#65118,#65119,#65120,#65121));
#13492=EDGE_LOOP('',(#65122,#65123,#65124,#65125));
#13493=EDGE_LOOP('',(#65126,#65127,#65128,#65129));
#13494=EDGE_LOOP('',(#65130,#65131,#65132,#65133));
#13495=EDGE_LOOP('',(#65134,#65135,#65136,#65137));
#13496=EDGE_LOOP('',(#65138,#65139,#65140,#65141));
#13497=EDGE_LOOP('',(#65142,#65143,#65144,#65145));
#13498=EDGE_LOOP('',(#65146,#65147,#65148,#65149));
#13499=EDGE_LOOP('',(#65150,#65151,#65152,#65153));
#13500=EDGE_LOOP('',(#65154,#65155,#65156,#65157));
#13501=EDGE_LOOP('',(#65158,#65159,#65160,#65161));
#13502=EDGE_LOOP('',(#65162,#65163,#65164,#65165));
#13503=EDGE_LOOP('',(#65166,#65167,#65168,#65169));
#13504=EDGE_LOOP('',(#65170,#65171,#65172,#65173));
#13505=EDGE_LOOP('',(#65174,#65175,#65176,#65177,#65178,#65179));
#13506=EDGE_LOOP('',(#65180,#65181,#65182,#65183));
#13507=EDGE_LOOP('',(#65184,#65185,#65186,#65187));
#13508=EDGE_LOOP('',(#65188,#65189,#65190,#65191));
#13509=EDGE_LOOP('',(#65192,#65193,#65194,#65195));
#13510=EDGE_LOOP('',(#65196,#65197,#65198,#65199));
#13511=EDGE_LOOP('',(#65200,#65201,#65202,#65203));
#13512=EDGE_LOOP('',(#65204,#65205,#65206,#65207));
#13513=EDGE_LOOP('',(#65208,#65209,#65210,#65211));
#13514=EDGE_LOOP('',(#65212,#65213,#65214,#65215));
#13515=EDGE_LOOP('',(#65216,#65217,#65218,#65219));
#13516=EDGE_LOOP('',(#65220,#65221,#65222,#65223));
#13517=EDGE_LOOP('',(#65224,#65225,#65226,#65227));
#13518=EDGE_LOOP('',(#65228,#65229,#65230,#65231));
#13519=EDGE_LOOP('',(#65232,#65233,#65234,#65235));
#13520=EDGE_LOOP('',(#65236,#65237,#65238,#65239));
#13521=EDGE_LOOP('',(#65240,#65241,#65242,#65243));
#13522=EDGE_LOOP('',(#65244,#65245,#65246,#65247));
#13523=EDGE_LOOP('',(#65248,#65249,#65250,#65251));
#13524=EDGE_LOOP('',(#65252,#65253,#65254,#65255));
#13525=EDGE_LOOP('',(#65256,#65257,#65258,#65259));
#13526=EDGE_LOOP('',(#65260,#65261,#65262,#65263));
#13527=EDGE_LOOP('',(#65264,#65265,#65266,#65267));
#13528=EDGE_LOOP('',(#65268,#65269,#65270,#65271));
#13529=EDGE_LOOP('',(#65272,#65273,#65274,#65275));
#13530=EDGE_LOOP('',(#65276,#65277,#65278,#65279));
#13531=EDGE_LOOP('',(#65280,#65281,#65282,#65283));
#13532=EDGE_LOOP('',(#65284,#65285,#65286,#65287));
#13533=EDGE_LOOP('',(#65288,#65289,#65290,#65291));
#13534=EDGE_LOOP('',(#65292,#65293,#65294,#65295));
#13535=EDGE_LOOP('',(#65296,#65297,#65298,#65299));
#13536=EDGE_LOOP('',(#65300,#65301,#65302,#65303));
#13537=EDGE_LOOP('',(#65304,#65305,#65306,#65307));
#13538=EDGE_LOOP('',(#65308,#65309,#65310,#65311));
#13539=EDGE_LOOP('',(#65312,#65313,#65314,#65315));
#13540=EDGE_LOOP('',(#65316,#65317,#65318,#65319));
#13541=EDGE_LOOP('',(#65320,#65321,#65322,#65323));
#13542=EDGE_LOOP('',(#65324,#65325,#65326,#65327));
#13543=EDGE_LOOP('',(#65328,#65329,#65330,#65331));
#13544=EDGE_LOOP('',(#65332,#65333,#65334,#65335));
#13545=EDGE_LOOP('',(#65336,#65337,#65338,#65339));
#13546=EDGE_LOOP('',(#65340,#65341,#65342,#65343));
#13547=EDGE_LOOP('',(#65344,#65345,#65346,#65347));
#13548=EDGE_LOOP('',(#65348,#65349,#65350,#65351));
#13549=EDGE_LOOP('',(#65352,#65353,#65354,#65355));
#13550=EDGE_LOOP('',(#65356,#65357,#65358,#65359));
#13551=EDGE_LOOP('',(#65360,#65361,#65362,#65363));
#13552=EDGE_LOOP('',(#65364,#65365,#65366,#65367));
#13553=EDGE_LOOP('',(#65368,#65369,#65370,#65371));
#13554=EDGE_LOOP('',(#65372,#65373,#65374,#65375));
#13555=EDGE_LOOP('',(#65376,#65377,#65378,#65379));
#13556=EDGE_LOOP('',(#65380,#65381,#65382,#65383));
#13557=EDGE_LOOP('',(#65384,#65385,#65386,#65387));
#13558=EDGE_LOOP('',(#65388,#65389,#65390,#65391));
#13559=EDGE_LOOP('',(#65392,#65393,#65394,#65395));
#13560=EDGE_LOOP('',(#65396,#65397,#65398,#65399));
#13561=EDGE_LOOP('',(#65400,#65401,#65402,#65403));
#13562=EDGE_LOOP('',(#65404,#65405,#65406,#65407));
#13563=EDGE_LOOP('',(#65408,#65409,#65410,#65411));
#13564=EDGE_LOOP('',(#65412,#65413,#65414,#65415));
#13565=EDGE_LOOP('',(#65416,#65417,#65418,#65419));
#13566=EDGE_LOOP('',(#65420,#65421,#65422,#65423));
#13567=EDGE_LOOP('',(#65424,#65425,#65426,#65427));
#13568=EDGE_LOOP('',(#65428,#65429,#65430,#65431));
#13569=EDGE_LOOP('',(#65432,#65433,#65434,#65435));
#13570=EDGE_LOOP('',(#65436,#65437,#65438,#65439));
#13571=EDGE_LOOP('',(#65440,#65441,#65442,#65443));
#13572=EDGE_LOOP('',(#65444,#65445,#65446,#65447));
#13573=EDGE_LOOP('',(#65448,#65449,#65450,#65451));
#13574=EDGE_LOOP('',(#65452,#65453,#65454,#65455));
#13575=EDGE_LOOP('',(#65456,#65457,#65458,#65459));
#13576=EDGE_LOOP('',(#65460,#65461,#65462,#65463));
#13577=EDGE_LOOP('',(#65464,#65465,#65466,#65467));
#13578=EDGE_LOOP('',(#65468,#65469,#65470,#65471));
#13579=EDGE_LOOP('',(#65472,#65473,#65474,#65475));
#13580=EDGE_LOOP('',(#65476,#65477,#65478,#65479));
#13581=EDGE_LOOP('',(#65480,#65481,#65482,#65483));
#13582=EDGE_LOOP('',(#65484,#65485,#65486,#65487));
#13583=EDGE_LOOP('',(#65488,#65489,#65490,#65491));
#13584=EDGE_LOOP('',(#65492,#65493,#65494,#65495));
#13585=EDGE_LOOP('',(#65496,#65497,#65498,#65499));
#13586=EDGE_LOOP('',(#65500,#65501,#65502,#65503));
#13587=EDGE_LOOP('',(#65504,#65505,#65506,#65507));
#13588=EDGE_LOOP('',(#65508,#65509,#65510,#65511));
#13589=EDGE_LOOP('',(#65512,#65513,#65514,#65515));
#13590=EDGE_LOOP('',(#65516,#65517,#65518,#65519));
#13591=EDGE_LOOP('',(#65520,#65521,#65522,#65523));
#13592=EDGE_LOOP('',(#65524,#65525,#65526,#65527));
#13593=EDGE_LOOP('',(#65528,#65529,#65530,#65531));
#13594=EDGE_LOOP('',(#65532,#65533,#65534,#65535));
#13595=EDGE_LOOP('',(#65536,#65537,#65538,#65539));
#13596=EDGE_LOOP('',(#65540,#65541,#65542,#65543));
#13597=EDGE_LOOP('',(#65544,#65545,#65546,#65547));
#13598=EDGE_LOOP('',(#65548,#65549,#65550,#65551));
#13599=EDGE_LOOP('',(#65552,#65553,#65554,#65555));
#13600=EDGE_LOOP('',(#65556,#65557,#65558,#65559));
#13601=EDGE_LOOP('',(#65560,#65561,#65562,#65563));
#13602=EDGE_LOOP('',(#65564,#65565,#65566,#65567));
#13603=EDGE_LOOP('',(#65568,#65569,#65570,#65571));
#13604=EDGE_LOOP('',(#65572,#65573,#65574,#65575));
#13605=EDGE_LOOP('',(#65576,#65577,#65578,#65579));
#13606=EDGE_LOOP('',(#65580,#65581,#65582,#65583));
#13607=EDGE_LOOP('',(#65584,#65585,#65586,#65587));
#13608=EDGE_LOOP('',(#65588,#65589,#65590,#65591));
#13609=EDGE_LOOP('',(#65592,#65593,#65594,#65595));
#13610=EDGE_LOOP('',(#65596,#65597,#65598,#65599));
#13611=EDGE_LOOP('',(#65600,#65601,#65602,#65603));
#13612=EDGE_LOOP('',(#65604,#65605,#65606,#65607));
#13613=EDGE_LOOP('',(#65608,#65609,#65610,#65611,#65612));
#13614=EDGE_LOOP('',(#65613,#65614,#65615,#65616));
#13615=EDGE_LOOP('',(#65617,#65618,#65619,#65620,#65621));
#13616=EDGE_LOOP('',(#65622,#65623,#65624,#65625));
#13617=EDGE_LOOP('',(#65626,#65627,#65628,#65629));
#13618=EDGE_LOOP('',(#65630,#65631,#65632,#65633,#65634));
#13619=EDGE_LOOP('',(#65635,#65636,#65637,#65638,#65639));
#13620=EDGE_LOOP('',(#65640,#65641,#65642,#65643,#65644));
#13621=EDGE_LOOP('',(#65645,#65646,#65647,#65648));
#13622=EDGE_LOOP('',(#65649,#65650,#65651,#65652));
#13623=EDGE_LOOP('',(#65653,#65654,#65655,#65656,#65657));
#13624=EDGE_LOOP('',(#65658,#65659,#65660,#65661,#65662));
#13625=EDGE_LOOP('',(#65663,#65664,#65665,#65666,#65667));
#13626=EDGE_LOOP('',(#65668,#65669,#65670,#65671,#65672));
#13627=EDGE_LOOP('',(#65673,#65674,#65675,#65676));
#13628=EDGE_LOOP('',(#65677,#65678,#65679,#65680));
#13629=EDGE_LOOP('',(#65681,#65682,#65683,#65684));
#13630=EDGE_LOOP('',(#65685,#65686,#65687,#65688));
#13631=EDGE_LOOP('',(#65689,#65690,#65691,#65692,#65693));
#13632=EDGE_LOOP('',(#65694,#65695,#65696,#65697,#65698,#65699,#65700,#65701,
#65702,#65703,#65704,#65705,#65706,#65707,#65708,#65709,#65710,#65711,#65712,
#65713,#65714,#65715,#65716,#65717,#65718,#65719,#65720,#65721,#65722,#65723,
#65724,#65725,#65726,#65727,#65728,#65729,#65730,#65731,#65732,#65733,#65734,
#65735,#65736,#65737,#65738,#65739,#65740,#65741,#65742,#65743,#65744,#65745,
#65746,#65747,#65748,#65749,#65750,#65751,#65752,#65753,#65754,#65755,#65756,
#65757,#65758,#65759,#65760,#65761,#65762,#65763,#65764,#65765,#65766,#65767,
#65768,#65769,#65770,#65771,#65772,#65773,#65774,#65775,#65776,#65777,#65778,
#65779,#65780,#65781,#65782,#65783,#65784,#65785,#65786,#65787,#65788,#65789,
#65790,#65791,#65792,#65793,#65794,#65795,#65796,#65797,#65798,#65799,#65800,
#65801,#65802,#65803,#65804,#65805,#65806,#65807,#65808,#65809,#65810,#65811,
#65812,#65813,#65814,#65815,#65816,#65817,#65818,#65819,#65820,#65821,#65822,
#65823,#65824,#65825,#65826,#65827,#65828,#65829,#65830,#65831,#65832,#65833,
#65834,#65835,#65836,#65837,#65838,#65839,#65840,#65841));
#13633=EDGE_LOOP('',(#65842));
#13634=EDGE_LOOP('',(#65843));
#13635=EDGE_LOOP('',(#65844,#65845,#65846,#65847,#65848,#65849,#65850,#65851));
#13636=EDGE_LOOP('',(#65852,#65853,#65854,#65855,#65856,#65857,#65858,#65859));
#13637=EDGE_LOOP('',(#65860));
#13638=EDGE_LOOP('',(#65861,#65862,#65863,#65864));
#13639=EDGE_LOOP('',(#65865,#65866,#65867,#65868));
#13640=EDGE_LOOP('',(#65869,#65870,#65871,#65872));
#13641=EDGE_LOOP('',(#65873,#65874,#65875,#65876));
#13642=EDGE_LOOP('',(#65877,#65878,#65879,#65880));
#13643=EDGE_LOOP('',(#65881,#65882,#65883,#65884));
#13644=EDGE_LOOP('',(#65885,#65886,#65887,#65888));
#13645=EDGE_LOOP('',(#65889,#65890,#65891,#65892));
#13646=EDGE_LOOP('',(#65893,#65894,#65895,#65896));
#13647=EDGE_LOOP('',(#65897,#65898,#65899,#65900));
#13648=EDGE_LOOP('',(#65901,#65902,#65903,#65904));
#13649=EDGE_LOOP('',(#65905,#65906,#65907,#65908));
#13650=EDGE_LOOP('',(#65909,#65910,#65911,#65912));
#13651=EDGE_LOOP('',(#65913,#65914,#65915,#65916));
#13652=EDGE_LOOP('',(#65917,#65918,#65919,#65920));
#13653=EDGE_LOOP('',(#65921,#65922,#65923,#65924));
#13654=EDGE_LOOP('',(#65925,#65926,#65927,#65928));
#13655=EDGE_LOOP('',(#65929,#65930,#65931,#65932));
#13656=EDGE_LOOP('',(#65933,#65934,#65935,#65936));
#13657=EDGE_LOOP('',(#65937,#65938,#65939,#65940));
#13658=EDGE_LOOP('',(#65941,#65942,#65943,#65944));
#13659=EDGE_LOOP('',(#65945,#65946,#65947,#65948));
#13660=EDGE_LOOP('',(#65949,#65950,#65951,#65952));
#13661=EDGE_LOOP('',(#65953,#65954,#65955,#65956));
#13662=EDGE_LOOP('',(#65957,#65958,#65959,#65960));
#13663=EDGE_LOOP('',(#65961,#65962,#65963,#65964));
#13664=EDGE_LOOP('',(#65965,#65966,#65967,#65968));
#13665=EDGE_LOOP('',(#65969,#65970,#65971,#65972));
#13666=EDGE_LOOP('',(#65973,#65974,#65975,#65976));
#13667=EDGE_LOOP('',(#65977,#65978,#65979,#65980));
#13668=EDGE_LOOP('',(#65981,#65982,#65983,#65984));
#13669=EDGE_LOOP('',(#65985,#65986,#65987,#65988));
#13670=EDGE_LOOP('',(#65989,#65990,#65991,#65992));
#13671=EDGE_LOOP('',(#65993,#65994,#65995,#65996));
#13672=EDGE_LOOP('',(#65997,#65998,#65999,#66000));
#13673=EDGE_LOOP('',(#66001,#66002,#66003,#66004));
#13674=EDGE_LOOP('',(#66005,#66006,#66007,#66008,#66009,#66010,#66011,#66012,
#66013,#66014,#66015,#66016,#66017,#66018,#66019,#66020,#66021,#66022,#66023,
#66024,#66025,#66026,#66027,#66028,#66029,#66030,#66031,#66032,#66033,#66034,
#66035,#66036,#66037,#66038,#66039,#66040,#66041,#66042,#66043,#66044,#66045,
#66046,#66047,#66048,#66049,#66050,#66051,#66052,#66053,#66054,#66055,#66056,
#66057,#66058,#66059,#66060,#66061,#66062,#66063,#66064,#66065,#66066,#66067,
#66068,#66069,#66070,#66071,#66072,#66073,#66074,#66075,#66076,#66077,#66078,
#66079,#66080,#66081,#66082,#66083,#66084,#66085,#66086,#66087,#66088,#66089,
#66090,#66091,#66092,#66093,#66094,#66095,#66096,#66097,#66098,#66099,#66100,
#66101,#66102,#66103,#66104,#66105,#66106,#66107,#66108,#66109,#66110,#66111,
#66112,#66113,#66114,#66115,#66116,#66117,#66118,#66119,#66120,#66121,#66122,
#66123,#66124,#66125,#66126,#66127,#66128,#66129,#66130,#66131,#66132,#66133,
#66134,#66135,#66136,#66137,#66138,#66139,#66140,#66141,#66142,#66143,#66144,
#66145,#66146,#66147,#66148,#66149,#66150,#66151,#66152));
#13675=EDGE_LOOP('',(#66153));
#13676=EDGE_LOOP('',(#66154));
#13677=EDGE_LOOP('',(#66155));
#13678=EDGE_LOOP('',(#66156,#66157,#66158,#66159));
#13679=EDGE_LOOP('',(#66160,#66161,#66162,#66163));
#13680=EDGE_LOOP('',(#66164,#66165,#66166,#66167));
#13681=EDGE_LOOP('',(#66168,#66169,#66170,#66171));
#13682=EDGE_LOOP('',(#66172,#66173,#66174,#66175));
#13683=EDGE_LOOP('',(#66176,#66177,#66178,#66179));
#13684=EDGE_LOOP('',(#66180,#66181,#66182,#66183));
#13685=EDGE_LOOP('',(#66184,#66185,#66186,#66187));
#13686=EDGE_LOOP('',(#66188,#66189,#66190,#66191));
#13687=EDGE_LOOP('',(#66192,#66193,#66194,#66195));
#13688=EDGE_LOOP('',(#66196,#66197,#66198,#66199));
#13689=EDGE_LOOP('',(#66200,#66201,#66202,#66203));
#13690=EDGE_LOOP('',(#66204,#66205,#66206,#66207));
#13691=EDGE_LOOP('',(#66208,#66209,#66210,#66211));
#13692=EDGE_LOOP('',(#66212,#66213,#66214,#66215));
#13693=EDGE_LOOP('',(#66216,#66217,#66218,#66219));
#13694=EDGE_LOOP('',(#66220,#66221,#66222,#66223));
#13695=EDGE_LOOP('',(#66224,#66225,#66226,#66227));
#13696=EDGE_LOOP('',(#66228,#66229,#66230,#66231));
#13697=EDGE_LOOP('',(#66232,#66233,#66234,#66235));
#13698=EDGE_LOOP('',(#66236,#66237,#66238,#66239));
#13699=EDGE_LOOP('',(#66240,#66241,#66242,#66243));
#13700=EDGE_LOOP('',(#66244,#66245,#66246,#66247));
#13701=EDGE_LOOP('',(#66248,#66249,#66250,#66251));
#13702=EDGE_LOOP('',(#66252,#66253,#66254,#66255));
#13703=EDGE_LOOP('',(#66256,#66257,#66258,#66259));
#13704=EDGE_LOOP('',(#66260,#66261,#66262,#66263));
#13705=EDGE_LOOP('',(#66264,#66265,#66266,#66267));
#13706=EDGE_LOOP('',(#66268,#66269,#66270,#66271));
#13707=EDGE_LOOP('',(#66272,#66273,#66274,#66275));
#13708=EDGE_LOOP('',(#66276,#66277,#66278,#66279));
#13709=EDGE_LOOP('',(#66280,#66281,#66282,#66283));
#13710=EDGE_LOOP('',(#66284,#66285,#66286,#66287));
#13711=EDGE_LOOP('',(#66288,#66289,#66290,#66291));
#13712=EDGE_LOOP('',(#66292,#66293,#66294,#66295));
#13713=EDGE_LOOP('',(#66296,#66297,#66298,#66299));
#13714=EDGE_LOOP('',(#66300,#66301,#66302,#66303));
#13715=EDGE_LOOP('',(#66304,#66305,#66306,#66307));
#13716=EDGE_LOOP('',(#66308,#66309,#66310,#66311));
#13717=EDGE_LOOP('',(#66312,#66313,#66314,#66315));
#13718=EDGE_LOOP('',(#66316,#66317,#66318,#66319));
#13719=EDGE_LOOP('',(#66320,#66321,#66322,#66323));
#13720=EDGE_LOOP('',(#66324,#66325,#66326,#66327));
#13721=EDGE_LOOP('',(#66328,#66329,#66330,#66331));
#13722=EDGE_LOOP('',(#66332,#66333,#66334,#66335));
#13723=EDGE_LOOP('',(#66336,#66337,#66338,#66339));
#13724=EDGE_LOOP('',(#66340,#66341,#66342,#66343));
#13725=EDGE_LOOP('',(#66344,#66345,#66346,#66347));
#13726=EDGE_LOOP('',(#66348,#66349,#66350,#66351));
#13727=EDGE_LOOP('',(#66352,#66353,#66354,#66355));
#13728=EDGE_LOOP('',(#66356,#66357,#66358,#66359));
#13729=EDGE_LOOP('',(#66360,#66361,#66362,#66363));
#13730=EDGE_LOOP('',(#66364,#66365,#66366,#66367));
#13731=EDGE_LOOP('',(#66368,#66369,#66370,#66371));
#13732=EDGE_LOOP('',(#66372,#66373,#66374,#66375));
#13733=EDGE_LOOP('',(#66376,#66377,#66378,#66379));
#13734=EDGE_LOOP('',(#66380,#66381,#66382,#66383));
#13735=EDGE_LOOP('',(#66384,#66385,#66386,#66387));
#13736=EDGE_LOOP('',(#66388,#66389,#66390,#66391));
#13737=EDGE_LOOP('',(#66392,#66393,#66394,#66395));
#13738=EDGE_LOOP('',(#66396,#66397,#66398,#66399));
#13739=EDGE_LOOP('',(#66400,#66401,#66402,#66403));
#13740=EDGE_LOOP('',(#66404,#66405,#66406,#66407));
#13741=EDGE_LOOP('',(#66408,#66409,#66410,#66411));
#13742=EDGE_LOOP('',(#66412,#66413,#66414,#66415));
#13743=EDGE_LOOP('',(#66416,#66417,#66418,#66419));
#13744=EDGE_LOOP('',(#66420,#66421,#66422,#66423));
#13745=EDGE_LOOP('',(#66424,#66425,#66426,#66427));
#13746=EDGE_LOOP('',(#66428,#66429,#66430,#66431));
#13747=EDGE_LOOP('',(#66432,#66433,#66434,#66435));
#13748=EDGE_LOOP('',(#66436,#66437,#66438,#66439));
#13749=EDGE_LOOP('',(#66440,#66441,#66442,#66443));
#13750=EDGE_LOOP('',(#66444,#66445,#66446,#66447));
#13751=EDGE_LOOP('',(#66448,#66449,#66450,#66451));
#13752=EDGE_LOOP('',(#66452,#66453,#66454,#66455));
#13753=EDGE_LOOP('',(#66456,#66457,#66458,#66459));
#13754=EDGE_LOOP('',(#66460,#66461,#66462,#66463));
#13755=EDGE_LOOP('',(#66464,#66465,#66466,#66467));
#13756=EDGE_LOOP('',(#66468,#66469,#66470,#66471));
#13757=EDGE_LOOP('',(#66472,#66473,#66474,#66475));
#13758=EDGE_LOOP('',(#66476,#66477,#66478,#66479));
#13759=EDGE_LOOP('',(#66480,#66481,#66482,#66483));
#13760=EDGE_LOOP('',(#66484,#66485,#66486,#66487));
#13761=EDGE_LOOP('',(#66488,#66489,#66490,#66491));
#13762=EDGE_LOOP('',(#66492,#66493,#66494,#66495));
#13763=EDGE_LOOP('',(#66496,#66497,#66498,#66499));
#13764=EDGE_LOOP('',(#66500,#66501,#66502,#66503));
#13765=EDGE_LOOP('',(#66504,#66505,#66506,#66507));
#13766=EDGE_LOOP('',(#66508,#66509,#66510,#66511));
#13767=EDGE_LOOP('',(#66512,#66513,#66514,#66515));
#13768=EDGE_LOOP('',(#66516,#66517,#66518,#66519));
#13769=EDGE_LOOP('',(#66520,#66521,#66522,#66523));
#13770=EDGE_LOOP('',(#66524,#66525,#66526,#66527));
#13771=EDGE_LOOP('',(#66528,#66529,#66530,#66531));
#13772=EDGE_LOOP('',(#66532,#66533,#66534,#66535));
#13773=EDGE_LOOP('',(#66536,#66537,#66538,#66539));
#13774=EDGE_LOOP('',(#66540,#66541,#66542,#66543));
#13775=EDGE_LOOP('',(#66544,#66545,#66546,#66547));
#13776=EDGE_LOOP('',(#66548,#66549,#66550,#66551));
#13777=EDGE_LOOP('',(#66552,#66553,#66554,#66555));
#13778=EDGE_LOOP('',(#66556,#66557,#66558,#66559));
#13779=EDGE_LOOP('',(#66560,#66561,#66562,#66563));
#13780=EDGE_LOOP('',(#66564,#66565,#66566,#66567));
#13781=EDGE_LOOP('',(#66568,#66569,#66570,#66571));
#13782=EDGE_LOOP('',(#66572,#66573,#66574,#66575));
#13783=EDGE_LOOP('',(#66576,#66577,#66578,#66579));
#13784=EDGE_LOOP('',(#66580,#66581,#66582,#66583));
#13785=EDGE_LOOP('',(#66584,#66585,#66586,#66587));
#13786=EDGE_LOOP('',(#66588));
#13787=EDGE_LOOP('',(#66589));
#13788=EDGE_LOOP('',(#66590));
#13789=EDGE_LOOP('',(#66591));
#13790=EDGE_LOOP('',(#66592));
#13791=EDGE_LOOP('',(#66593));
#13792=EDGE_LOOP('',(#66594,#66595,#66596,#66597));
#13793=EDGE_LOOP('',(#66598,#66599,#66600,#66601));
#13794=EDGE_LOOP('',(#66602,#66603,#66604,#66605));
#13795=EDGE_LOOP('',(#66606,#66607,#66608,#66609));
#13796=EDGE_LOOP('',(#66610,#66611,#66612,#66613));
#13797=EDGE_LOOP('',(#66614,#66615,#66616,#66617));
#13798=EDGE_LOOP('',(#66618,#66619,#66620,#66621));
#13799=EDGE_LOOP('',(#66622,#66623,#66624,#66625,#66626,#66627,#66628,#66629));
#13800=EDGE_LOOP('',(#66630,#66631,#66632,#66633));
#13801=EDGE_LOOP('',(#66634,#66635,#66636,#66637));
#13802=EDGE_LOOP('',(#66638,#66639,#66640,#66641));
#13803=EDGE_LOOP('',(#66642,#66643,#66644,#66645));
#13804=EDGE_LOOP('',(#66646,#66647,#66648,#66649));
#13805=EDGE_LOOP('',(#66650,#66651,#66652,#66653));
#13806=EDGE_LOOP('',(#66654,#66655,#66656,#66657));
#13807=EDGE_LOOP('',(#66658,#66659,#66660,#66661,#66662,#66663,#66664,#66665));
#13808=EDGE_LOOP('',(#66666,#66667,#66668,#66669));
#13809=EDGE_LOOP('',(#66670,#66671,#66672,#66673));
#13810=EDGE_LOOP('',(#66674,#66675,#66676,#66677));
#13811=EDGE_LOOP('',(#66678,#66679,#66680,#66681));
#13812=EDGE_LOOP('',(#66682,#66683,#66684,#66685));
#13813=EDGE_LOOP('',(#66686,#66687,#66688,#66689));
#13814=EDGE_LOOP('',(#66690,#66691,#66692,#66693));
#13815=EDGE_LOOP('',(#66694,#66695,#66696,#66697));
#13816=EDGE_LOOP('',(#66698,#66699,#66700,#66701));
#13817=EDGE_LOOP('',(#66702,#66703,#66704,#66705));
#13818=EDGE_LOOP('',(#66706,#66707,#66708,#66709));
#13819=EDGE_LOOP('',(#66710,#66711,#66712,#66713));
#13820=EDGE_LOOP('',(#66714,#66715,#66716,#66717));
#13821=EDGE_LOOP('',(#66718,#66719,#66720,#66721));
#13822=EDGE_LOOP('',(#66722));
#13823=EDGE_LOOP('',(#66723));
#19464=CIRCLE('',#97245,9.);
#19465=CIRCLE('',#97246,9.);
#19466=CIRCLE('',#97248,9.);
#19467=CIRCLE('',#97249,9.);
#19468=CIRCLE('',#97251,9.);
#19469=CIRCLE('',#97252,9.);
#19470=CIRCLE('',#97254,9.);
#19471=CIRCLE('',#97255,9.);
#19472=CIRCLE('',#97257,9.);
#19473=CIRCLE('',#97258,9.);
#19474=CIRCLE('',#97260,9.);
#19475=CIRCLE('',#97261,9.);
#19476=CIRCLE('',#97263,9.);
#19477=CIRCLE('',#97264,9.);
#19478=CIRCLE('',#97266,9.);
#19479=CIRCLE('',#97267,9.);
#19480=CIRCLE('',#97269,9.);
#19481=CIRCLE('',#97270,9.);
#19482=CIRCLE('',#97272,9.);
#19483=CIRCLE('',#97273,9.);
#19484=CIRCLE('',#97275,9.);
#19485=CIRCLE('',#97276,9.);
#19486=CIRCLE('',#97278,9.);
#19487=CIRCLE('',#97279,9.);
#19488=CIRCLE('',#97281,9.);
#19489=CIRCLE('',#97282,9.);
#19490=CIRCLE('',#97284,9.);
#19491=CIRCLE('',#97285,9.);
#19492=CIRCLE('',#97287,9.);
#19493=CIRCLE('',#97288,9.);
#19494=CIRCLE('',#97290,9.);
#19495=CIRCLE('',#97291,9.);
#19496=CIRCLE('',#97293,9.);
#19497=CIRCLE('',#97294,9.);
#19498=CIRCLE('',#97296,9.);
#19499=CIRCLE('',#97297,9.);
#19500=CIRCLE('',#97299,9.);
#19501=CIRCLE('',#97300,9.);
#19502=CIRCLE('',#97302,9.);
#19503=CIRCLE('',#97303,9.);
#19504=CIRCLE('',#97305,9.);
#19505=CIRCLE('',#97306,9.);
#19506=CIRCLE('',#97308,9.);
#19507=CIRCLE('',#97309,9.);
#19508=CIRCLE('',#97311,9.);
#19509=CIRCLE('',#97312,9.);
#19510=CIRCLE('',#97314,9.);
#19511=CIRCLE('',#97315,9.);
#19512=CIRCLE('',#97317,9.);
#19513=CIRCLE('',#97318,9.);
#19514=CIRCLE('',#97320,9.);
#19515=CIRCLE('',#97321,9.);
#19516=CIRCLE('',#97323,9.);
#19517=CIRCLE('',#97324,9.);
#19518=CIRCLE('',#97326,9.);
#19519=CIRCLE('',#97327,9.);
#19520=CIRCLE('',#97329,9.);
#19521=CIRCLE('',#97330,9.);
#19522=CIRCLE('',#97332,9.);
#19523=CIRCLE('',#97333,9.);
#19524=CIRCLE('',#97335,9.);
#19525=CIRCLE('',#97336,9.);
#19526=CIRCLE('',#97338,9.);
#19527=CIRCLE('',#97339,9.);
#19528=CIRCLE('',#97341,9.);
#19529=CIRCLE('',#97342,9.);
#19530=CIRCLE('',#97344,9.);
#19531=CIRCLE('',#97345,9.);
#19532=CIRCLE('',#97347,9.);
#19533=CIRCLE('',#97348,9.);
#19534=CIRCLE('',#97350,9.);
#19535=CIRCLE('',#97351,9.);
#19536=CIRCLE('',#97353,9.);
#19537=CIRCLE('',#97354,9.);
#19538=CIRCLE('',#97356,9.);
#19539=CIRCLE('',#97357,9.);
#19540=CIRCLE('',#97359,9.);
#19541=CIRCLE('',#97360,9.);
#19542=CIRCLE('',#97362,9.);
#19543=CIRCLE('',#97363,9.);
#19544=CIRCLE('',#97365,9.);
#19545=CIRCLE('',#97366,9.);
#19546=CIRCLE('',#97368,9.);
#19547=CIRCLE('',#97369,9.);
#19548=CIRCLE('',#97371,9.);
#19549=CIRCLE('',#97372,9.);
#19550=CIRCLE('',#97374,9.);
#19551=CIRCLE('',#97375,9.);
#19552=CIRCLE('',#97377,9.);
#19553=CIRCLE('',#97378,9.);
#19554=CIRCLE('',#97380,9.);
#19555=CIRCLE('',#97381,9.);
#19556=CIRCLE('',#97383,9.);
#19557=CIRCLE('',#97384,9.);
#19558=CIRCLE('',#97386,9.);
#19559=CIRCLE('',#97387,9.);
#19560=CIRCLE('',#97389,9.);
#19561=CIRCLE('',#97390,9.);
#19562=CIRCLE('',#97392,9.);
#19563=CIRCLE('',#97393,9.);
#19564=CIRCLE('',#97395,9.);
#19565=CIRCLE('',#97396,9.);
#19566=CIRCLE('',#97398,9.);
#19567=CIRCLE('',#97399,9.);
#19568=CIRCLE('',#97401,9.);
#19569=CIRCLE('',#97402,9.);
#19570=CIRCLE('',#97404,9.);
#19571=CIRCLE('',#97405,9.);
#19572=CIRCLE('',#97407,9.);
#19573=CIRCLE('',#97408,9.);
#19574=CIRCLE('',#97410,9.);
#19575=CIRCLE('',#97411,9.);
#19576=CIRCLE('',#97413,9.);
#19577=CIRCLE('',#97414,9.);
#19578=CIRCLE('',#97416,9.);
#19579=CIRCLE('',#97417,9.);
#19580=CIRCLE('',#97419,9.);
#19581=CIRCLE('',#97420,9.);
#19582=CIRCLE('',#97422,9.);
#19583=CIRCLE('',#97423,9.);
#19584=CIRCLE('',#97425,9.);
#19585=CIRCLE('',#97426,9.);
#19586=CIRCLE('',#97428,9.);
#19587=CIRCLE('',#97429,9.);
#19588=CIRCLE('',#97431,9.);
#19589=CIRCLE('',#97432,9.);
#19590=CIRCLE('',#97434,9.);
#19591=CIRCLE('',#97435,9.);
#19592=CIRCLE('',#97437,9.);
#19593=CIRCLE('',#97438,9.);
#19594=CIRCLE('',#97440,9.);
#19595=CIRCLE('',#97441,9.);
#19596=CIRCLE('',#97443,9.);
#19597=CIRCLE('',#97444,9.);
#19598=CIRCLE('',#97446,9.);
#19599=CIRCLE('',#97447,9.);
#19600=CIRCLE('',#97449,9.);
#19601=CIRCLE('',#97450,9.);
#19602=CIRCLE('',#97452,9.);
#19603=CIRCLE('',#97453,9.);
#19604=CIRCLE('',#97455,2.5);
#19605=CIRCLE('',#97456,2.9);
#19606=CIRCLE('',#97457,2.5);
#19607=CIRCLE('',#97459,1.5);
#19608=CIRCLE('',#97460,1.7);
#19609=CIRCLE('',#97461,1.5);
#19610=CIRCLE('',#97463,1.5);
#19611=CIRCLE('',#97464,1.7);
#19612=CIRCLE('',#97465,1.5);
#19613=CIRCLE('',#97467,9.);
#19614=CIRCLE('',#97468,8.8);
#19615=CIRCLE('',#97469,9.);
#19616=CIRCLE('',#97471,1.5);
#19617=CIRCLE('',#97472,1.7);
#19618=CIRCLE('',#97474,1.5);
#19619=CIRCLE('',#97475,1.7);
#19620=CIRCLE('',#97477,3.5);
#19621=CIRCLE('',#97478,3.3);
#19622=CIRCLE('',#97479,3.5);
#19623=CIRCLE('',#97481,2.5);
#19624=CIRCLE('',#97482,2.7);
#19625=CIRCLE('',#97486,8.5);
#19626=CIRCLE('',#97489,3.5);
#19627=CIRCLE('',#97495,2.272884449);
#19628=CIRCLE('',#97497,2.272884449);
#19629=CIRCLE('',#97500,2.272884449);
#19630=CIRCLE('',#97502,2.272884449);
#19631=CIRCLE('',#97505,2.272884449);
#19632=CIRCLE('',#97507,2.272884449);
#19633=CIRCLE('',#97510,2.272884449);
#19634=CIRCLE('',#97512,2.272884449);
#19635=CIRCLE('',#97515,2.272884449);
#19636=CIRCLE('',#97517,2.272884449);
#19637=CIRCLE('',#97520,2.272884449);
#19638=CIRCLE('',#97522,2.272884449);
#19639=CIRCLE('',#97525,2.272884449);
#19640=CIRCLE('',#97527,2.27288445);
#19641=CIRCLE('',#97530,2.272884449);
#19642=CIRCLE('',#97532,2.272884449);
#19643=CIRCLE('',#97535,2.272884449);
#19644=CIRCLE('',#97537,2.272884449);
#19645=CIRCLE('',#97540,2.272884449);
#19646=CIRCLE('',#97542,2.272884449);
#19647=CIRCLE('',#97545,2.272884449);
#19648=CIRCLE('',#97547,2.27288445);
#19649=CIRCLE('',#97550,2.27288445);
#19650=CIRCLE('',#97552,2.272884449);
#19651=CIRCLE('',#97555,2.272884449);
#19652=CIRCLE('',#97557,2.272884449);
#19653=CIRCLE('',#97560,2.272884449);
#19654=CIRCLE('',#97562,2.272884449);
#19655=CIRCLE('',#97565,2.272884449);
#19656=CIRCLE('',#97567,2.272884449);
#19657=CIRCLE('',#97570,2.272884449);
#19658=CIRCLE('',#97572,2.272884449);
#19659=CIRCLE('',#97575,2.272884449);
#19660=CIRCLE('',#97577,2.272884449);
#19661=CIRCLE('',#97580,2.272884449);
#19662=CIRCLE('',#97582,2.272884449);
#19663=CIRCLE('',#97585,2.272884449);
#19664=CIRCLE('',#97587,2.272884449);
#19665=CIRCLE('',#97590,2.27288445);
#19666=CIRCLE('',#97592,2.272884449);
#19667=CIRCLE('',#97595,2.272884449);
#19668=CIRCLE('',#97597,2.272884449);
#19669=CIRCLE('',#97600,2.272884449);
#19670=CIRCLE('',#97602,2.272884449);
#19671=CIRCLE('',#97605,2.272884449);
#19672=CIRCLE('',#97607,2.272884449);
#19673=CIRCLE('',#97610,2.272884449);
#19674=CIRCLE('',#97612,2.272884449);
#19675=CIRCLE('',#97615,2.272884449);
#19676=CIRCLE('',#97617,2.272884449);
#19677=CIRCLE('',#97620,2.272884449);
#19678=CIRCLE('',#97622,2.272884449);
#19679=CIRCLE('',#97625,2.272884449);
#19680=CIRCLE('',#97627,2.272884449);
#19681=CIRCLE('',#97630,2.272884449);
#19682=CIRCLE('',#97632,2.272884449);
#19683=CIRCLE('',#97635,2.272884449);
#19684=CIRCLE('',#97637,2.272884449);
#19685=CIRCLE('',#97640,2.272884449);
#19686=CIRCLE('',#97642,2.272884449);
#19687=CIRCLE('',#97645,2.272884449);
#19688=CIRCLE('',#97647,2.272884449);
#19689=CIRCLE('',#97650,2.272884449);
#19690=CIRCLE('',#97652,2.272884449);
#19691=CIRCLE('',#97655,2.272884449);
#19692=CIRCLE('',#97657,2.272884449);
#19693=CIRCLE('',#97660,2.272884449);
#19694=CIRCLE('',#97662,2.272884449);
#19695=CIRCLE('',#97665,2.272884449);
#19696=CIRCLE('',#97667,2.27288445);
#19697=CIRCLE('',#97670,2.272884449);
#19698=CIRCLE('',#97672,2.272884449);
#19699=CIRCLE('',#97675,2.272884449);
#19700=CIRCLE('',#97677,2.272884449);
#19701=CIRCLE('',#97680,2.272884449);
#19702=CIRCLE('',#97682,2.272884449);
#19703=CIRCLE('',#97685,2.272884449);
#19704=CIRCLE('',#97687,2.272884449);
#19705=CIRCLE('',#97690,2.272884449);
#19706=CIRCLE('',#97692,2.272884449);
#19707=CIRCLE('',#97695,2.272884449);
#19708=CIRCLE('',#97697,2.272884449);
#19709=CIRCLE('',#97700,2.272884449);
#19710=CIRCLE('',#97702,2.27288445);
#19711=CIRCLE('',#97705,2.272884449);
#19712=CIRCLE('',#97707,2.272884449);
#19713=CIRCLE('',#97710,2.272884449);
#19714=CIRCLE('',#97712,2.272884449);
#19715=CIRCLE('',#97715,2.272884449);
#19716=CIRCLE('',#97717,2.272884449);
#19717=CIRCLE('',#97720,2.272884449);
#19718=CIRCLE('',#97722,2.27288445);
#19719=CIRCLE('',#97725,2.27288445);
#19720=CIRCLE('',#97727,2.272884449);
#19721=CIRCLE('',#97730,2.272884449);
#19722=CIRCLE('',#97732,2.272884449);
#19723=CIRCLE('',#97735,2.272884449);
#19724=CIRCLE('',#97737,2.272884449);
#19725=CIRCLE('',#97740,2.272884449);
#19726=CIRCLE('',#97742,2.272884449);
#19727=CIRCLE('',#97745,2.272884449);
#19728=CIRCLE('',#97747,2.272884449);
#19729=CIRCLE('',#97750,2.272884449);
#19730=CIRCLE('',#97752,2.272884449);
#19731=CIRCLE('',#97755,2.272884449);
#19732=CIRCLE('',#97757,2.272884449);
#19733=CIRCLE('',#97760,2.272884449);
#19734=CIRCLE('',#97762,2.272884449);
#19735=CIRCLE('',#97765,2.27288445);
#19736=CIRCLE('',#97767,2.272884449);
#19737=CIRCLE('',#97770,2.272884449);
#19738=CIRCLE('',#97772,2.272884449);
#19739=CIRCLE('',#97775,2.272884449);
#19740=CIRCLE('',#97777,2.272884449);
#19741=CIRCLE('',#97780,2.272884449);
#19742=CIRCLE('',#97782,2.272884449);
#19743=CIRCLE('',#97785,2.272884449);
#19744=CIRCLE('',#97787,2.272884449);
#19745=CIRCLE('',#97790,2.272884449);
#19746=CIRCLE('',#97792,2.272884449);
#19747=CIRCLE('',#97795,2.272884449);
#19748=CIRCLE('',#97797,2.272884449);
#19749=CIRCLE('',#97800,2.272884449);
#19750=CIRCLE('',#97802,2.272884449);
#19751=CIRCLE('',#97805,2.272884449);
#19752=CIRCLE('',#97807,2.272884449);
#19753=CIRCLE('',#97810,2.272884449);
#19754=CIRCLE('',#97812,2.272884449);
#19755=CIRCLE('',#97815,2.272884449);
#19756=CIRCLE('',#97817,2.272884449);
#19757=CIRCLE('',#97820,2.272884449);
#19758=CIRCLE('',#97822,2.272884449);
#19759=CIRCLE('',#97825,2.272884449);
#19760=CIRCLE('',#97827,2.272884449);
#19761=CIRCLE('',#97830,2.272884449);
#19762=CIRCLE('',#97832,2.272884449);
#19763=CIRCLE('',#97835,2.272884449);
#19764=CIRCLE('',#97837,2.272884449);
#19765=CIRCLE('',#97840,2.272884449);
#19766=CIRCLE('',#97842,2.27288445);
#19767=CIRCLE('',#97845,1.);
#19768=CIRCLE('',#97846,1.);
#19769=CIRCLE('',#97848,1.);
#19770=CIRCLE('',#97849,1.);
#19771=CIRCLE('',#97851,1.6);
#19772=CIRCLE('',#97852,0.1);
#19773=CIRCLE('',#97853,1.5);
#19774=CIRCLE('',#97855,1.6);
#19775=CIRCLE('',#97856,0.1);
#19776=CIRCLE('',#97857,1.5);
#19777=CIRCLE('',#97859,1.5);
#19778=CIRCLE('',#97860,0.2);
#19779=CIRCLE('',#97861,1.7);
#19780=CIRCLE('',#97862,1.5);
#19781=CIRCLE('',#97864,1.5);
#19782=CIRCLE('',#97865,0.2);
#19783=CIRCLE('',#97866,1.7);
#19784=CIRCLE('',#97868,2.8);
#19785=CIRCLE('',#97869,0.2);
#19786=CIRCLE('',#97870,3.);
#19787=CIRCLE('',#97871,3.);
#19788=CIRCLE('',#97873,0.4);
#19789=CIRCLE('',#97874,0.2);
#19790=CIRCLE('',#97875,0.6);
#19791=CIRCLE('',#97876,0.2);
#19792=CIRCLE('',#97878,0.4);
#19793=CIRCLE('',#97879,0.2);
#19794=CIRCLE('',#97880,0.6);
#19795=CIRCLE('',#97881,0.2);
#19796=CIRCLE('',#97883,3.9);
#19797=CIRCLE('',#97884,0.4);
#19798=CIRCLE('',#97885,3.5);
#19799=CIRCLE('',#97886,3.5);
#19800=CIRCLE('',#97888,1.1);
#19801=CIRCLE('',#97889,0.4);
#19802=CIRCLE('',#97890,1.5);
#19803=CIRCLE('',#97891,1.5);
#19804=CIRCLE('',#97893,1.1);
#19805=CIRCLE('',#97894,0.4);
#19806=CIRCLE('',#97895,1.5);
#19807=CIRCLE('',#97896,1.5);
#19808=CIRCLE('',#97898,0.4);
#19809=CIRCLE('',#97899,0.4);
#19810=CIRCLE('',#97901,0.4);
#19811=CIRCLE('',#97902,0.4);
#19812=CIRCLE('',#97904,3.5);
#19813=CIRCLE('',#97908,3.);
#19814=CIRCLE('',#97910,3.7);
#19815=CIRCLE('',#97911,3.7);
#19816=CIRCLE('',#97913,3.7);
#19817=CIRCLE('',#97914,3.7);
#19818=CIRCLE('',#97916,3.7);
#19819=CIRCLE('',#97917,3.7);
#19820=CIRCLE('',#97919,3.7);
#19821=CIRCLE('',#97920,3.7);
#19822=CIRCLE('',#97923,3.7);
#19823=CIRCLE('',#97924,8.624);
#19824=CIRCLE('',#97925,3.7);
#19825=CIRCLE('',#97926,9.75);
#19826=CIRCLE('',#97927,3.7);
#19827=CIRCLE('',#97928,8.624);
#19828=CIRCLE('',#97929,3.7);
#19829=CIRCLE('',#97930,9.75);
#19830=CIRCLE('',#97931,3.7);
#19831=CIRCLE('',#97932,8.624);
#19832=CIRCLE('',#97933,3.7);
#19833=CIRCLE('',#97934,9.75);
#19834=CIRCLE('',#97935,3.7);
#19835=CIRCLE('',#97936,8.624);
#19836=CIRCLE('',#97937,3.7);
#19837=CIRCLE('',#97938,9.75);
#19838=CIRCLE('',#97939,3.7);
#19839=CIRCLE('',#97940,8.624);
#19840=CIRCLE('',#97941,3.7);
#19841=CIRCLE('',#97942,9.75);
#19842=CIRCLE('',#97943,3.7);
#19843=CIRCLE('',#97944,8.624);
#19844=CIRCLE('',#97945,3.7);
#19845=CIRCLE('',#97946,9.75);
#19846=CIRCLE('',#97947,3.7);
#19847=CIRCLE('',#97948,8.624);
#19848=CIRCLE('',#97949,3.7);
#19849=CIRCLE('',#97950,9.75);
#19850=CIRCLE('',#97951,3.7);
#19851=CIRCLE('',#97952,8.624);
#19852=CIRCLE('',#97953,9.75);
#19853=CIRCLE('',#97954,3.7);
#19854=CIRCLE('',#97955,8.624);
#19855=CIRCLE('',#97956,9.75);
#19856=CIRCLE('',#97957,3.7);
#19857=CIRCLE('',#97958,8.624);
#19858=CIRCLE('',#97959,3.7);
#19859=CIRCLE('',#97960,9.75);
#19860=CIRCLE('',#97961,3.7);
#19861=CIRCLE('',#97962,8.624);
#19862=CIRCLE('',#97963,3.7);
#19863=CIRCLE('',#97964,9.75);
#19864=CIRCLE('',#97965,3.7);
#19865=CIRCLE('',#97966,8.624);
#19866=CIRCLE('',#97967,3.7);
#19867=CIRCLE('',#97968,9.75);
#19868=CIRCLE('',#97969,3.7);
#19869=CIRCLE('',#97970,8.624);
#19870=CIRCLE('',#97971,3.7);
#19871=CIRCLE('',#97972,9.75);
#19872=CIRCLE('',#97973,3.7);
#19873=CIRCLE('',#97974,8.624);
#19874=CIRCLE('',#97975,3.7);
#19875=CIRCLE('',#97976,9.75);
#19876=CIRCLE('',#97977,3.7);
#19877=CIRCLE('',#97978,8.624);
#19878=CIRCLE('',#97979,3.7);
#19879=CIRCLE('',#97980,9.75);
#19880=CIRCLE('',#97981,3.7);
#19881=CIRCLE('',#97982,8.624);
#19882=CIRCLE('',#97983,3.7);
#19883=CIRCLE('',#97984,9.75);
#19884=CIRCLE('',#97985,3.7);
#19885=CIRCLE('',#97986,8.624);
#19886=CIRCLE('',#97987,3.7);
#19887=CIRCLE('',#97988,9.75);
#19888=CIRCLE('',#97989,3.7);
#19889=CIRCLE('',#97990,8.624);
#19890=CIRCLE('',#97991,3.7);
#19891=CIRCLE('',#97992,9.75);
#19892=CIRCLE('',#97993,3.7);
#19893=CIRCLE('',#97994,8.624);
#19894=CIRCLE('',#97995,3.7);
#19895=CIRCLE('',#97996,9.75);
#19896=CIRCLE('',#97997,3.7);
#19897=CIRCLE('',#97998,8.624);
#19898=CIRCLE('',#97999,3.7);
#19899=CIRCLE('',#98000,9.75);
#19900=CIRCLE('',#98001,3.7);
#19901=CIRCLE('',#98002,8.624);
#19902=CIRCLE('',#98003,3.7);
#19903=CIRCLE('',#98004,9.75);
#19904=CIRCLE('',#98005,3.7);
#19905=CIRCLE('',#98006,8.624);
#19906=CIRCLE('',#98007,3.7);
#19907=CIRCLE('',#98008,9.75);
#19908=CIRCLE('',#98009,3.7);
#19909=CIRCLE('',#98010,8.624);
#19910=CIRCLE('',#98011,3.7);
#19911=CIRCLE('',#98012,9.75);
#19912=CIRCLE('',#98013,3.7);
#19913=CIRCLE('',#98014,8.624);
#19914=CIRCLE('',#98015,3.7);
#19915=CIRCLE('',#98016,9.75);
#19916=CIRCLE('',#98017,3.7);
#19917=CIRCLE('',#98018,8.624);
#19918=CIRCLE('',#98019,3.7);
#19919=CIRCLE('',#98020,9.75);
#19920=CIRCLE('',#98021,3.7);
#19921=CIRCLE('',#98022,8.624);
#19922=CIRCLE('',#98023,3.7);
#19923=CIRCLE('',#98024,9.75);
#19924=CIRCLE('',#98025,3.7);
#19925=CIRCLE('',#98026,8.624);
#19926=CIRCLE('',#98027,3.7);
#19927=CIRCLE('',#98028,9.75);
#19928=CIRCLE('',#98029,3.7);
#19929=CIRCLE('',#98030,8.624);
#19930=CIRCLE('',#98031,3.7);
#19931=CIRCLE('',#98032,9.75);
#19932=CIRCLE('',#98033,3.7);
#19933=CIRCLE('',#98034,8.624);
#19934=CIRCLE('',#98035,3.7);
#19935=CIRCLE('',#98036,9.75);
#19936=CIRCLE('',#98037,3.7);
#19937=CIRCLE('',#98038,8.624);
#19938=CIRCLE('',#98039,3.7);
#19939=CIRCLE('',#98040,9.75);
#19940=CIRCLE('',#98041,8.624);
#19941=CIRCLE('',#98042,3.7);
#19942=CIRCLE('',#98043,9.75);
#19943=CIRCLE('',#98044,8.624);
#19944=CIRCLE('',#98045,3.7);
#19945=CIRCLE('',#98046,9.75);
#19946=CIRCLE('',#98047,3.7);
#19947=CIRCLE('',#98048,8.624);
#19948=CIRCLE('',#98049,3.7);
#19949=CIRCLE('',#98050,9.75);
#19950=CIRCLE('',#98051,3.7);
#19951=CIRCLE('',#98052,8.624);
#19952=CIRCLE('',#98053,3.7);
#19953=CIRCLE('',#98054,9.75);
#19954=CIRCLE('',#98055,3.7);
#19955=CIRCLE('',#98056,8.624);
#19956=CIRCLE('',#98057,3.7);
#19957=CIRCLE('',#98058,9.75);
#19958=CIRCLE('',#98059,3.7);
#19959=CIRCLE('',#98060,8.624);
#19960=CIRCLE('',#98061,3.7);
#19961=CIRCLE('',#98062,9.75);
#19962=CIRCLE('',#98063,3.7);
#19963=CIRCLE('',#98064,8.624);
#19964=CIRCLE('',#98065,3.7);
#19965=CIRCLE('',#98066,9.75);
#19966=CIRCLE('',#98067,4.8);
#19967=CIRCLE('',#98068,0.6);
#19968=CIRCLE('',#98069,7.4);
#19969=CIRCLE('',#98070,0.6);
#19970=CIRCLE('',#98071,0.6);
#19971=CIRCLE('',#98072,0.6);
#19972=CIRCLE('',#98073,7.4);
#19973=CIRCLE('',#98074,0.6);
#19974=CIRCLE('',#98075,4.8);
#19975=CIRCLE('',#98076,0.6);
#19976=CIRCLE('',#98078,9.75);
#19977=CIRCLE('',#98080,9.75);
#19978=CIRCLE('',#98082,9.75);
#19979=CIRCLE('',#98084,9.75);
#19980=CIRCLE('',#98086,9.75);
#19981=CIRCLE('',#98088,9.75);
#19982=CIRCLE('',#98090,9.75);
#19983=CIRCLE('',#98092,9.75);
#19984=CIRCLE('',#98094,9.75);
#19985=CIRCLE('',#98096,9.75);
#19986=CIRCLE('',#98098,9.75);
#19987=CIRCLE('',#98100,9.75);
#19988=CIRCLE('',#98102,9.75);
#19989=CIRCLE('',#98104,9.75);
#19990=CIRCLE('',#98106,9.75);
#19991=CIRCLE('',#98108,9.75);
#19992=CIRCLE('',#98110,9.75);
#19993=CIRCLE('',#98112,9.75);
#19994=CIRCLE('',#98114,9.75);
#19995=CIRCLE('',#98116,9.75);
#19996=CIRCLE('',#98118,9.75);
#19997=CIRCLE('',#98120,9.75);
#19998=CIRCLE('',#98122,9.75);
#19999=CIRCLE('',#98124,9.75);
#20000=CIRCLE('',#98126,9.75);
#20001=CIRCLE('',#98128,9.75);
#20002=CIRCLE('',#98130,9.75);
#20003=CIRCLE('',#98132,9.75);
#20004=CIRCLE('',#98134,9.75);
#20005=CIRCLE('',#98136,9.75);
#20006=CIRCLE('',#98138,9.75);
#20007=CIRCLE('',#98140,9.75);
#20008=CIRCLE('',#98142,9.75);
#20009=CIRCLE('',#98144,9.75);
#20010=CIRCLE('',#98146,9.75);
#20011=CIRCLE('',#98148,9.75);
#20012=CIRCLE('',#98150,3.7);
#20013=CIRCLE('',#98151,3.7);
#20014=CIRCLE('',#98152,8.624);
#20015=CIRCLE('',#98153,3.7);
#20016=CIRCLE('',#98154,3.7);
#20017=CIRCLE('',#98155,8.624);
#20018=CIRCLE('',#98156,3.7);
#20019=CIRCLE('',#98157,3.7);
#20020=CIRCLE('',#98158,8.624);
#20021=CIRCLE('',#98159,3.7);
#20022=CIRCLE('',#98160,3.7);
#20023=CIRCLE('',#98161,8.624);
#20024=CIRCLE('',#98162,3.7);
#20025=CIRCLE('',#98163,3.7);
#20026=CIRCLE('',#98164,8.624);
#20027=CIRCLE('',#98165,3.7);
#20028=CIRCLE('',#98166,3.7);
#20029=CIRCLE('',#98167,8.624);
#20030=CIRCLE('',#98168,3.7);
#20031=CIRCLE('',#98169,8.624);
#20032=CIRCLE('',#98170,3.7);
#20033=CIRCLE('',#98171,8.624);
#20034=CIRCLE('',#98172,3.7);
#20035=CIRCLE('',#98173,9.75);
#20036=CIRCLE('',#98174,3.7);
#20037=CIRCLE('',#98175,8.624);
#20038=CIRCLE('',#98176,3.7);
#20039=CIRCLE('',#98177,3.7);
#20040=CIRCLE('',#98178,8.624);
#20041=CIRCLE('',#98179,3.7);
#20042=CIRCLE('',#98180,3.7);
#20043=CIRCLE('',#98181,8.624);
#20044=CIRCLE('',#98182,3.7);
#20045=CIRCLE('',#98183,3.7);
#20046=CIRCLE('',#98184,8.624);
#20047=CIRCLE('',#98185,3.7);
#20048=CIRCLE('',#98186,3.7);
#20049=CIRCLE('',#98187,8.624);
#20050=CIRCLE('',#98188,3.7);
#20051=CIRCLE('',#98189,3.7);
#20052=CIRCLE('',#98190,8.624);
#20053=CIRCLE('',#98191,3.7);
#20054=CIRCLE('',#98192,3.7);
#20055=CIRCLE('',#98193,8.624);
#20056=CIRCLE('',#98194,3.7);
#20057=CIRCLE('',#98195,3.7);
#20058=CIRCLE('',#98196,8.624);
#20059=CIRCLE('',#98197,3.7);
#20060=CIRCLE('',#98198,3.7);
#20061=CIRCLE('',#98199,8.624);
#20062=CIRCLE('',#98200,3.7);
#20063=CIRCLE('',#98201,3.7);
#20064=CIRCLE('',#98202,8.624);
#20065=CIRCLE('',#98203,3.7);
#20066=CIRCLE('',#98204,3.7);
#20067=CIRCLE('',#98205,8.624);
#20068=CIRCLE('',#98206,3.7);
#20069=CIRCLE('',#98207,3.7);
#20070=CIRCLE('',#98208,8.624);
#20071=CIRCLE('',#98209,3.7);
#20072=CIRCLE('',#98210,3.7);
#20073=CIRCLE('',#98211,8.624);
#20074=CIRCLE('',#98212,3.7);
#20075=CIRCLE('',#98213,3.7);
#20076=CIRCLE('',#98214,8.624);
#20077=CIRCLE('',#98215,3.7);
#20078=CIRCLE('',#98216,3.7);
#20079=CIRCLE('',#98217,8.624);
#20080=CIRCLE('',#98218,3.7);
#20081=CIRCLE('',#98219,3.7);
#20082=CIRCLE('',#98220,8.624);
#20083=CIRCLE('',#98221,3.7);
#20084=CIRCLE('',#98222,3.7);
#20085=CIRCLE('',#98223,8.624);
#20086=CIRCLE('',#98224,3.7);
#20087=CIRCLE('',#98225,3.7);
#20088=CIRCLE('',#98226,8.624);
#20089=CIRCLE('',#98227,3.7);
#20090=CIRCLE('',#98228,3.7);
#20091=CIRCLE('',#98229,8.624);
#20092=CIRCLE('',#98230,3.7);
#20093=CIRCLE('',#98231,3.7);
#20094=CIRCLE('',#98232,8.624);
#20095=CIRCLE('',#98233,3.7);
#20096=CIRCLE('',#98234,8.624);
#20097=CIRCLE('',#98235,3.7);
#20098=CIRCLE('',#98236,8.624);
#20099=CIRCLE('',#98237,3.7);
#20100=CIRCLE('',#98238,3.7);
#20101=CIRCLE('',#98239,8.624);
#20102=CIRCLE('',#98240,3.7);
#20103=CIRCLE('',#98241,3.7);
#20104=CIRCLE('',#98242,8.624);
#20105=CIRCLE('',#98243,3.7);
#20106=CIRCLE('',#98244,3.7);
#20107=CIRCLE('',#98245,8.624);
#20108=CIRCLE('',#98246,3.7);
#20109=CIRCLE('',#98247,3.7);
#20110=CIRCLE('',#98248,8.624);
#20111=CIRCLE('',#98249,3.7);
#20112=CIRCLE('',#98250,3.7);
#20113=CIRCLE('',#98251,8.624);
#20114=CIRCLE('',#98252,3.7);
#20115=CIRCLE('',#98253,3.7);
#20116=CIRCLE('',#98254,8.624);
#20117=CIRCLE('',#98255,3.7);
#20118=CIRCLE('',#98256,3.7);
#20119=CIRCLE('',#98257,8.624);
#20120=CIRCLE('',#98372,0.4);
#20121=CIRCLE('',#98373,0.4);
#20122=CIRCLE('',#98375,5.);
#20123=CIRCLE('',#98376,5.);
#20124=CIRCLE('',#98378,0.4);
#20125=CIRCLE('',#98379,0.4);
#20126=CIRCLE('',#98382,0.4);
#20127=CIRCLE('',#98384,7.2);
#20128=CIRCLE('',#98385,7.2);
#20129=CIRCLE('',#98388,0.4);
#20130=CIRCLE('',#98389,0.4);
#20131=CIRCLE('',#98392,7.2);
#20132=CIRCLE('',#98393,7.2);
#20133=CIRCLE('',#98395,0.4);
#20134=CIRCLE('',#98398,0.4);
#20135=CIRCLE('',#98399,0.4);
#20136=CIRCLE('',#98401,5.);
#20137=CIRCLE('',#98402,5.);
#20138=CIRCLE('',#98405,0.2);
#20139=CIRCLE('',#98406,0.2);
#20140=CIRCLE('',#98408,0.2);
#20141=CIRCLE('',#98411,0.2);
#20142=CIRCLE('',#98413,0.2);
#20143=CIRCLE('',#98415,0.2);
#20144=CIRCLE('',#98418,0.2);
#20145=CIRCLE('',#98419,0.2);
#20146=CIRCLE('',#98421,0.2);
#20147=CIRCLE('',#98424,0.2);
#20148=CIRCLE('',#98426,0.2);
#20149=CIRCLE('',#98428,0.2);
#23757=B_SPLINE_CURVE_WITH_KNOTS('',3,(#145877,#145878,#145879,#145880,
#145881,#145882,#145883,#145884,#145885,#145886),.UNSPECIFIED.,.F.,.F.,
(4,2,2,2,4),(-0.67890407197508,-0.638811382079944,-0.567890404574991,-0.49694871747295,
-0.466428520808092),.UNSPECIFIED.);
#23758=B_SPLINE_CURVE_WITH_KNOTS('',3,(#145890,#145891,#145892,#145893,
#145894,#145895,#145896,#145897,#145898,#145899),.UNSPECIFIED.,.F.,.F.,
(4,2,2,2,4),(-0.678904071966558,-0.638811382082276,-0.567890404578285,-0.496948717476777,
-0.466428520822623),.UNSPECIFIED.);
#23759=B_SPLINE_CURVE_WITH_KNOTS('',3,(#145904,#145905,#145906,#145907,
#145908,#145909,#145910,#145911,#145912,#145913),.UNSPECIFIED.,.F.,.F.,
(4,2,2,2,4),(-0.678904071957372,-0.638811382080974,-0.567890404576434,-0.496948717474622,
-0.466428520828439),.UNSPECIFIED.);
#23760=B_SPLINE_CURVE_WITH_KNOTS('',3,(#145917,#145918,#145919,#145920,
#145921,#145922,#145923,#145924,#145925,#145926),.UNSPECIFIED.,.F.,.F.,
(4,2,2,2,4),(-0.678904071960599,-0.638811382082355,-0.567890404578383,-0.496948717476885,
-0.466428520828765),.UNSPECIFIED.);
#23761=B_SPLINE_CURVE_WITH_KNOTS('',3,(#145931,#145932,#145933,#145934,
#145935,#145936,#145937,#145938,#145939,#145940),.UNSPECIFIED.,.F.,.F.,
(4,2,2,2,4),(-0.678904071989196,-0.638811382078946,-0.567890404573567,-0.496948717471288,
-0.466428520791381),.UNSPECIFIED.);
#23762=B_SPLINE_CURVE_WITH_KNOTS('',3,(#145944,#145945,#145946,#145947,
#145948,#145949,#145950,#145951,#145952,#145953),.UNSPECIFIED.,.F.,.F.,
(4,2,2,2,4),(-0.67890407198423,-0.638811382082675,-0.567890404578853,-0.496948717477438,
-0.466428520805978),.UNSPECIFIED.);
#23763=B_SPLINE_CURVE_WITH_KNOTS('',3,(#145958,#145959,#145960,#145961,
#145962,#145963,#145964,#145965,#145966,#145967),.UNSPECIFIED.,.F.,.F.,
(4,2,2,2,4),(-0.67890407199097,-0.638811382078488,-0.567890404572896,-0.496948717470497,
-0.466428520788399),.UNSPECIFIED.);
#23764=B_SPLINE_CURVE_WITH_KNOTS('',3,(#145971,#145972,#145973,#145974,
#145975,#145976,#145977,#145978,#145979,#145980),.UNSPECIFIED.,.F.,.F.,
(4,2,2,2,4),(-0.678904071978841,-0.63881138207855,-0.567890404573014,-0.496948717470648,
-0.466428520800727),.UNSPECIFIED.);
#23765=B_SPLINE_CURVE_WITH_KNOTS('',3,(#145985,#145986,#145987,#145988,
#145989,#145990,#145991,#145992,#145993,#145994),.UNSPECIFIED.,.F.,.F.,
(4,2,2,2,4),(-0.678904071978394,-0.638811382081562,-0.567890404577268,-0.496948717475591,
-0.466428520789366),.UNSPECIFIED.);
#23766=B_SPLINE_CURVE_WITH_KNOTS('',3,(#145998,#145999,#146000,#146001,
#146002,#146003,#146004,#146005,#146006,#146007),.UNSPECIFIED.,.F.,.F.,
(4,2,2,2,4),(-0.67890407196277,-0.638811382079109,-0.567890404573782,-0.49694871747153,
-0.466428520818205),.UNSPECIFIED.);
#23767=B_SPLINE_CURVE_WITH_KNOTS('',3,(#146012,#146013,#146014,#146015,
#146016,#146017,#146018,#146019,#146020,#146021),.UNSPECIFIED.,.F.,.F.,
(4,2,2,2,4),(-0.678904071951945,-0.63881138208195,-0.567890404577823,-0.496948717476241,
-0.466428520836395),.UNSPECIFIED.);
#23768=B_SPLINE_CURVE_WITH_KNOTS('',3,(#146025,#146026,#146027,#146028,
#146029,#146030,#146031,#146032,#146033,#146034),.UNSPECIFIED.,.F.,.F.,
(4,2,2,2,4),(-0.678904071984223,-0.638811382077183,-0.567890404571043,-0.496948717468339,
-0.46642852079177),.UNSPECIFIED.);
#23769=B_SPLINE_CURVE_WITH_KNOTS('',3,(#146039,#146040,#146041,#146042,
#146043,#146044,#146045,#146046,#146047,#146048),.UNSPECIFIED.,.F.,.F.,
(4,2,2,2,4),(-0.678904071946678,-0.638811382083569,-0.567890404580107,-0.496948717478892,
-0.466428520817328),.UNSPECIFIED.);
#23770=B_SPLINE_CURVE_WITH_KNOTS('',3,(#146052,#146053,#146054,#146055,
#146056,#146057,#146058,#146059,#146060,#146061),.UNSPECIFIED.,.F.,.F.,
(4,2,2,2,4),(-0.678904071981315,-0.638811382080222,-0.567890404575361,-0.496948717473367,
-0.466428520802537),.UNSPECIFIED.);
#23771=B_SPLINE_CURVE_WITH_KNOTS('',3,(#146066,#146067,#146068,#146069,
#146070,#146071,#146072,#146073,#146074,#146075),.UNSPECIFIED.,.F.,.F.,
(4,2,2,2,4),(-0.678904071991326,-0.638811382081232,-0.567890404576792,-0.496948717475035,
-0.466428520807193),.UNSPECIFIED.);
#23772=B_SPLINE_CURVE_WITH_KNOTS('',3,(#146079,#146080,#146081,#146082,
#146083,#146084,#146085,#146086,#146087,#146088),.UNSPECIFIED.,.F.,.F.,
(4,2,2,2,4),(-0.678904071999347,-0.638811382081042,-0.567890404576521,-0.496948717474717,
-0.466428520786623),.UNSPECIFIED.);
#23773=B_SPLINE_CURVE_WITH_KNOTS('',3,(#146093,#146094,#146095,#146096,
#146097,#146098,#146099,#146100,#146101,#146102),.UNSPECIFIED.,.F.,.F.,
(4,2,2,2,4),(-0.678904071986479,-0.638811382080361,-0.56789040457558,-0.496948717473635,
-0.466428520797767),.UNSPECIFIED.);
#23774=B_SPLINE_CURVE_WITH_KNOTS('',3,(#146106,#146107,#146108,#146109,
#146110,#146111,#146112,#146113,#146114,#146115),.UNSPECIFIED.,.F.,.F.,
(4,2,2,2,4),(-0.678904071955915,-0.6388113820817,-0.567890404577456,-0.496948717475805,
-0.466428520793425),.UNSPECIFIED.);
#23775=B_SPLINE_CURVE_WITH_KNOTS('',3,(#146120,#146121,#146122,#146123,
#146124,#146125,#146126,#146127,#146128,#146129),.UNSPECIFIED.,.F.,.F.,
(4,2,2,2,4),(-0.67890407199572,-0.63881138208008,-0.567890404575174,-0.49694871747316,
-0.466428520827877),.UNSPECIFIED.);
#23776=B_SPLINE_CURVE_WITH_KNOTS('',3,(#146133,#146134,#146135,#146136,
#146137,#146138,#146139,#146140,#146141,#146142),.UNSPECIFIED.,.F.,.F.,
(4,2,2,2,4),(-0.678904071968026,-0.638811382077951,-0.567890404572114,-0.496948717469576,
-0.466428520809921),.UNSPECIFIED.);
#23777=B_SPLINE_CURVE_WITH_KNOTS('',3,(#146147,#146148,#146149,#146150,
#146151,#146152,#146153,#146154,#146155,#146156),.UNSPECIFIED.,.F.,.F.,
(4,2,2,2,4),(-0.678904071991079,-0.63881138208447,-0.567890404581382,-0.496948717480376,
-0.466428520838142),.UNSPECIFIED.);
#23778=B_SPLINE_CURVE_WITH_KNOTS('',3,(#146160,#146161,#146162,#146163,
#146164,#146165,#146166,#146167,#146168,#146169),.UNSPECIFIED.,.F.,.F.,
(4,2,2,2,4),(-0.678904072013284,-0.638811382084366,-0.567890404581246,-0.496948717480222,
-0.466428520827388),.UNSPECIFIED.);
#23779=B_SPLINE_CURVE_WITH_KNOTS('',3,(#146174,#146175,#146176,#146177,
#146178,#146179,#146180,#146181,#146182,#146183),.UNSPECIFIED.,.F.,.F.,
(4,2,2,2,4),(-0.678904071986053,-0.638811382076461,-0.567890404570022,-0.49694871746715,
-0.466428520788073),.UNSPECIFIED.);
#23780=B_SPLINE_CURVE_WITH_KNOTS('',3,(#146187,#146188,#146189,#146190,
#146191,#146192,#146193,#146194,#146195,#146196),.UNSPECIFIED.,.F.,.F.,
(4,2,2,2,4),(-0.67890407199352,-0.638811382083378,-0.567890404579852,-0.496948717478602,
-0.466428520817659),.UNSPECIFIED.);
#23781=B_SPLINE_CURVE_WITH_KNOTS('',3,(#146201,#146202,#146203,#146204,
#146205,#146206,#146207,#146208,#146209,#146210),.UNSPECIFIED.,.F.,.F.,
(4,2,2,2,4),(-0.678904071973262,-0.638811382076435,-0.567890404569995,-0.496948717467124,
-0.466428520774712),.UNSPECIFIED.);
#23782=B_SPLINE_CURVE_WITH_KNOTS('',3,(#146214,#146215,#146216,#146217,
#146218,#146219,#146220,#146221,#146222,#146223),.UNSPECIFIED.,.F.,.F.,
(4,2,2,2,4),(-0.678904071987068,-0.638811382078544,-0.567890404572966,-0.496948717470576,
-0.466428520843256),.UNSPECIFIED.);
#23783=B_SPLINE_CURVE_WITH_KNOTS('',3,(#146228,#146229,#146230,#146231,
#146232,#146233,#146234,#146235,#146236,#146237),.UNSPECIFIED.,.F.,.F.,
(4,2,2,2,4),(-0.678904071987881,-0.638811382084155,-0.567890404580941,-0.496948717479863,
-0.466428520806137),.UNSPECIFIED.);
#23784=B_SPLINE_CURVE_WITH_KNOTS('',3,(#146241,#146242,#146243,#146244,
#146245,#146246,#146247,#146248,#146249,#146250),.UNSPECIFIED.,.F.,.F.,
(4,2,2,2,4),(-0.678904072009282,-0.638811382083207,-0.567890404579597,-0.496948717478301,
-0.466428520834868),.UNSPECIFIED.);
#23785=B_SPLINE_CURVE_WITH_KNOTS('',3,(#146255,#146256,#146257,#146258,
#146259,#146260,#146261,#146262,#146263,#146264),.UNSPECIFIED.,.F.,.F.,
(4,2,2,2,4),(-0.678904071972205,-0.638811382079633,-0.567890404574503,-0.496948717472359,
-0.466428520810097),.UNSPECIFIED.);
#23786=B_SPLINE_CURVE_WITH_KNOTS('',3,(#146268,#146269,#146270,#146271,
#146272,#146273,#146274,#146275,#146276,#146277),.UNSPECIFIED.,.F.,.F.,
(4,2,2,2,4),(-0.678904071979395,-0.63881138208103,-0.567890404576514,-0.496948717474714,
-0.466428520794118),.UNSPECIFIED.);
#23787=B_SPLINE_CURVE_WITH_KNOTS('',3,(#146282,#146283,#146284,#146285,
#146286,#146287,#146288,#146289,#146290,#146291),.UNSPECIFIED.,.F.,.F.,
(4,2,2,2,4),(-0.678904071999173,-0.638811382081402,-0.567890404577046,-0.496948717475338,
-0.466428520787755),.UNSPECIFIED.);
#23788=B_SPLINE_CURVE_WITH_KNOTS('',3,(#146295,#146296,#146297,#146298,
#146299,#146300,#146301,#146302,#146303,#146304),.UNSPECIFIED.,.F.,.F.,
(4,2,2,2,4),(-0.678904071953474,-0.638811382080186,-0.567890404575329,-0.496948717473341,
-0.466428520830318),.UNSPECIFIED.);
#23789=B_SPLINE_CURVE_WITH_KNOTS('',3,(#146309,#146310,#146311,#146312,
#146313,#146314,#146315,#146316,#146317,#146318),.UNSPECIFIED.,.F.,.F.,
(4,2,2,2,4),(-0.678904072002962,-0.638811382083278,-0.567890404578545,-0.496948717476505,
-0.466428520787081),.UNSPECIFIED.);
#23790=B_SPLINE_CURVE_WITH_KNOTS('',3,(#146322,#146323,#146324,#146325,
#146326,#146327,#146328,#146329,#146330,#146331),.UNSPECIFIED.,.F.,.F.,
(4,2,2,2,4),(-0.678904071991591,-0.638811382082784,-0.567890404578999,-0.496948717477604,
-0.466428520798887),.UNSPECIFIED.);
#23791=B_SPLINE_CURVE_WITH_KNOTS('',3,(#146336,#146337,#146338,#146339,
#146340,#146341,#146342,#146343,#146344,#146345),.UNSPECIFIED.,.F.,.F.,
(4,2,2,2,4),(-0.678904071964557,-0.638811382077309,-0.567890404571244,-0.496948717468583,
-0.466428520811788),.UNSPECIFIED.);
#23792=B_SPLINE_CURVE_WITH_KNOTS('',3,(#146349,#146350,#146351,#146352,
#146353,#146354,#146355,#146356,#146357,#146358),.UNSPECIFIED.,.F.,.F.,
(4,2,2,2,4),(-0.678904071968788,-0.638811382079797,-0.567890404574743,-0.496948717472643,
-0.466428520813952),.UNSPECIFIED.);
#23793=B_SPLINE_CURVE_WITH_KNOTS('',3,(#146363,#146364,#146365,#146366,
#146367,#146368,#146369,#146370,#146371,#146372),.UNSPECIFIED.,.F.,.F.,
(4,2,2,2,4),(-0.678904071989876,-0.638811382082106,-0.567890404578026,-0.496948717476466,
-0.466428520798835),.UNSPECIFIED.);
#23794=B_SPLINE_CURVE_WITH_KNOTS('',3,(#146376,#146377,#146378,#146379,
#146380,#146381,#146382,#146383,#146384,#146385),.UNSPECIFIED.,.F.,.F.,
(4,2,2,2,4),(-0.678904072003597,-0.63881138208164,-0.567890404577412,-0.496948717475776,
-0.466428520791274),.UNSPECIFIED.);
#23795=B_SPLINE_CURVE_WITH_KNOTS('',3,(#146390,#146391,#146392,#146393,
#146394,#146395,#146396,#146397,#146398,#146399),.UNSPECIFIED.,.F.,.F.,
(4,2,2,2,4),(-0.678904071951742,-0.638811382079469,-0.567890404574304,-0.496948717472142,
-0.46642852083018),.UNSPECIFIED.);
#23796=B_SPLINE_CURVE_WITH_KNOTS('',3,(#146403,#146404,#146405,#146406,
#146407,#146408,#146409,#146410,#146411,#146412),.UNSPECIFIED.,.F.,.F.,
(4,2,2,2,4),(-0.678904071999128,-0.638811382080533,-0.567890404575816,-0.496948717473904,
-0.466428520785546),.UNSPECIFIED.);
#23797=B_SPLINE_CURVE_WITH_KNOTS('',3,(#146417,#146418,#146419,#146420,
#146421,#146422,#146423,#146424,#146425,#146426),.UNSPECIFIED.,.F.,.F.,
(4,2,2,2,4),(-0.678904071974422,-0.638811382079115,-0.567890404573812,-0.496948717471574,
-0.466428520806596),.UNSPECIFIED.);
#23798=B_SPLINE_CURVE_WITH_KNOTS('',3,(#146430,#146431,#146432,#146433,
#146434,#146435,#146436,#146437,#146438,#146439),.UNSPECIFIED.,.F.,.F.,
(4,2,2,2,4),(-0.678904071970067,-0.638811382078595,-0.567890404573052,-0.49694871747068,
-0.46642852080958),.UNSPECIFIED.);
#23799=B_SPLINE_CURVE_WITH_KNOTS('',3,(#146444,#146445,#146446,#146447,
#146448,#146449,#146450,#146451,#146452,#146453),.UNSPECIFIED.,.F.,.F.,
(4,2,2,2,4),(-0.678904071989481,-0.63881138208252,-0.567890404578625,-0.496948717477172,
-0.466428520800322),.UNSPECIFIED.);
#23800=B_SPLINE_CURVE_WITH_KNOTS('',3,(#146457,#146458,#146459,#146460,
#146461,#146462,#146463,#146464,#146465,#146466),.UNSPECIFIED.,.F.,.F.,
(4,2,2,2,4),(-0.678904071985814,-0.638811382083261,-0.567890404579705,-0.49694871747844,
-0.46642852080594),.UNSPECIFIED.);
#23801=B_SPLINE_CURVE_WITH_KNOTS('',3,(#146471,#146472,#146473,#146474,
#146475,#146476,#146477,#146478,#146479,#146480),.UNSPECIFIED.,.F.,.F.,
(4,2,2,2,4),(-0.678904071977239,-0.638811382076132,-0.567890404569544,-0.496948717466588,
-0.46642852081418),.UNSPECIFIED.);
#23802=B_SPLINE_CURVE_WITH_KNOTS('',3,(#146484,#146485,#146486,#146487,
#146488,#146489,#146490,#146491,#146492,#146493),.UNSPECIFIED.,.F.,.F.,
(4,2,2,2,4),(-0.678904071975199,-0.638811382077187,-0.567890404571049,-0.496948717468346,
-0.466428520800801),.UNSPECIFIED.);
#23803=B_SPLINE_CURVE_WITH_KNOTS('',3,(#146498,#146499,#146500,#146501,
#146502,#146503,#146504,#146505,#146506,#146507),.UNSPECIFIED.,.F.,.F.,
(4,2,2,2,4),(-0.678904071948059,-0.638811382083722,-0.567890404580332,-0.496948717479159,
-0.466428520818515),.UNSPECIFIED.);
#23804=B_SPLINE_CURVE_WITH_KNOTS('',3,(#146511,#146512,#146513,#146514,
#146515,#146516,#146517,#146518,#146519,#146520),.UNSPECIFIED.,.F.,.F.,
(4,2,2,2,4),(-0.678904071957727,-0.638811382077612,-0.567890404571677,-0.496948717469091,
-0.466428520789048),.UNSPECIFIED.);
#23805=B_SPLINE_CURVE_WITH_KNOTS('',3,(#146525,#146526,#146527,#146528,
#146529,#146530,#146531,#146532,#146533,#146534),.UNSPECIFIED.,.F.,.F.,
(4,2,2,2,4),(-0.678904071980107,-0.638811382084215,-0.567890404581017,-0.496948717479948,
-0.466428520814056),.UNSPECIFIED.);
#23806=B_SPLINE_CURVE_WITH_KNOTS('',3,(#146538,#146539,#146540,#146541,
#146542,#146543,#146544,#146545,#146546,#146547),.UNSPECIFIED.,.F.,.F.,
(4,2,2,2,4),(-0.678904071988661,-0.638811382083323,-0.567890404579782,-0.496948717478526,
-0.466428520803241),.UNSPECIFIED.);
#23807=B_SPLINE_CURVE_WITH_KNOTS('',3,(#146552,#146553,#146554,#146555,
#146556,#146557,#146558,#146559,#146560,#146561),.UNSPECIFIED.,.F.,.F.,
(4,2,2,2,4),(-0.678904071967123,-0.638811382077973,-0.567890404572164,-0.496948717469645,
-0.46642852080234),.UNSPECIFIED.);
#23808=B_SPLINE_CURVE_WITH_KNOTS('',3,(#146565,#146566,#146567,#146568,
#146569,#146570,#146571,#146572,#146573,#146574),.UNSPECIFIED.,.F.,.F.,
(4,2,2,2,4),(-0.678904071996527,-0.638811382080123,-0.567890404575202,-0.496948717473172,
-0.466428520787041),.UNSPECIFIED.);
#23809=B_SPLINE_CURVE_WITH_KNOTS('',3,(#146579,#146580,#146581,#146582,
#146583,#146584,#146585,#146586,#146587,#146588),.UNSPECIFIED.,.F.,.F.,
(4,2,2,2,4),(-0.678904071994029,-0.638811382081138,-0.567890404576668,-0.496948717474894,
-0.4664285208321),.UNSPECIFIED.);
#23810=B_SPLINE_CURVE_WITH_KNOTS('',3,(#146592,#146593,#146594,#146595,
#146596,#146597,#146598,#146599,#146600,#146601),.UNSPECIFIED.,.F.,.F.,
(4,2,2,2,4),(-0.678904071987538,-0.638811382080587,-0.567890404575871,-0.496948717473957,
-0.466428520797245),.UNSPECIFIED.);
#23811=B_SPLINE_CURVE_WITH_KNOTS('',3,(#146606,#146607,#146608,#146609,
#146610,#146611,#146612,#146613,#146614,#146615),.UNSPECIFIED.,.F.,.F.,
(4,2,2,2,4),(-0.678904071998108,-0.638811382080726,-0.567890404576086,-0.496948717474218,
-0.466428520787065),.UNSPECIFIED.);
#23812=B_SPLINE_CURVE_WITH_KNOTS('',3,(#146619,#146620,#146621,#146622,
#146623,#146624,#146625,#146626,#146627,#146628),.UNSPECIFIED.,.F.,.F.,
(4,2,2,2,4),(-0.678904071979078,-0.638811382081879,-0.567890404577713,-0.496948717476107,
-0.466428520806676),.UNSPECIFIED.);
#23813=B_SPLINE_CURVE_WITH_KNOTS('',3,(#146633,#146634,#146635,#146636,
#146637,#146638,#146639,#146640,#146641,#146642),.UNSPECIFIED.,.F.,.F.,
(4,2,2,2,4),(-0.678904072012607,-0.638811382080162,-0.567890404575286,-0.496948717473285,
-0.466428520771103),.UNSPECIFIED.);
#23814=B_SPLINE_CURVE_WITH_KNOTS('',3,(#146646,#146647,#146648,#146649,
#146650,#146651,#146652,#146653,#146654,#146655),.UNSPECIFIED.,.F.,.F.,
(4,2,2,2,4),(-0.678904071978783,-0.638811382085326,-0.5678904045826,-0.496948717481796,
-0.466428520818266),.UNSPECIFIED.);
#23815=B_SPLINE_CURVE_WITH_KNOTS('',3,(#146660,#146661,#146662,#146663,
#146664,#146665,#146666,#146667,#146668,#146669),.UNSPECIFIED.,.F.,.F.,
(4,2,2,2,4),(-0.678904071984418,-0.638811382077011,-0.567890404570846,-0.496948717468133,
-0.466428520791198),.UNSPECIFIED.);
#23816=B_SPLINE_CURVE_WITH_KNOTS('',3,(#146673,#146674,#146675,#146676,
#146677,#146678,#146679,#146680,#146681,#146682),.UNSPECIFIED.,.F.,.F.,
(4,2,2,2,4),(-0.678904072001018,-0.638811382081384,-0.567890404576977,-0.496948717475233,
-0.466428520835578),.UNSPECIFIED.);
#23817=B_SPLINE_CURVE_WITH_KNOTS('',3,(#146687,#146688,#146689,#146690,
#146691,#146692,#146693,#146694,#146695,#146696),.UNSPECIFIED.,.F.,.F.,
(4,2,2,2,4),(-0.678904071963263,-0.638811382080034,-0.567890404575033,-0.496948717472957,
-0.466428520820018),.UNSPECIFIED.);
#23818=B_SPLINE_CURVE_WITH_KNOTS('',3,(#146700,#146701,#146702,#146703,
#146704,#146705,#146706,#146707,#146708,#146709),.UNSPECIFIED.,.F.,.F.,
(4,2,2,2,4),(-0.678904071978785,-0.63881138208184,-0.567890404577665,-0.496948717476054,
-0.466428520809261),.UNSPECIFIED.);
#23819=B_SPLINE_CURVE_WITH_KNOTS('',3,(#146714,#146715,#146716,#146717,
#146718,#146719,#146720,#146721,#146722,#146723),.UNSPECIFIED.,.F.,.F.,
(4,2,2,2,4),(-0.678904071979651,-0.638811382078958,-0.567890404573559,-0.496948717471267,
-0.466428520800927),.UNSPECIFIED.);
#23820=B_SPLINE_CURVE_WITH_KNOTS('',3,(#146727,#146728,#146729,#146730,
#146731,#146732,#146733,#146734,#146735,#146736),.UNSPECIFIED.,.F.,.F.,
(4,2,2,2,4),(-0.678904071992989,-0.638811382079457,-0.567890404574321,-0.496948717472181,
-0.46642852078896),.UNSPECIFIED.);
#23821=B_SPLINE_CURVE_WITH_KNOTS('',3,(#146741,#146742,#146743,#146744,
#146745,#146746,#146747,#146748,#146749,#146750),.UNSPECIFIED.,.F.,.F.,
(4,2,2,2,4),(-0.67890407199661,-0.638811382082501,-0.567890404578577,-0.496948717477103,
-0.466428520807697),.UNSPECIFIED.);
#23822=B_SPLINE_CURVE_WITH_KNOTS('',3,(#146754,#146755,#146756,#146757,
#146758,#146759,#146760,#146761,#146762,#146763),.UNSPECIFIED.,.F.,.F.,
(4,2,2,2,4),(-0.678904071992571,-0.638811382080303,-0.567890404575509,-0.496948717473556,
-0.466428520781529),.UNSPECIFIED.);
#23823=B_SPLINE_CURVE_WITH_KNOTS('',3,(#146768,#146769,#146770,#146771,
#146772,#146773,#146774,#146775,#146776,#146777),.UNSPECIFIED.,.F.,.F.,
(4,2,2,2,4),(-0.678904071957711,-0.63881138208108,-0.567890404576584,-0.496948717474795,
-0.466428520828368),.UNSPECIFIED.);
#23824=B_SPLINE_CURVE_WITH_KNOTS('',3,(#146781,#146782,#146783,#146784,
#146785,#146786,#146787,#146788,#146789,#146790),.UNSPECIFIED.,.F.,.F.,
(4,2,2,2,4),(-0.678904071955128,-0.638811382079591,-0.567890404574442,-0.496948717472286,
-0.466428520827057),.UNSPECIFIED.);
#23825=B_SPLINE_CURVE_WITH_KNOTS('',3,(#146795,#146796,#146797,#146798,
#146799,#146800,#146801,#146802,#146803,#146804),.UNSPECIFIED.,.F.,.F.,
(4,2,2,2,4),(-0.67890407196334,-0.638811382080692,-0.567890404576,-0.496948717474097,
-0.466428520821681),.UNSPECIFIED.);
#23826=B_SPLINE_CURVE_WITH_KNOTS('',3,(#146808,#146809,#146810,#146811,
#146812,#146813,#146814,#146815,#146816,#146817),.UNSPECIFIED.,.F.,.F.,
(4,2,2,2,4),(-0.678904071975058,-0.638811382079965,-0.567890404575,-0.49694871747295,
-0.466428520808137),.UNSPECIFIED.);
#23827=B_SPLINE_CURVE_WITH_KNOTS('',3,(#146822,#146823,#146824,#146825,
#146826,#146827,#146828,#146829,#146830,#146831),.UNSPECIFIED.,.F.,.F.,
(4,2,2,2,4),(-0.678904071975006,-0.638811382079877,-0.567890404574935,-0.496948717472904,
-0.46642852080805),.UNSPECIFIED.);
#23828=B_SPLINE_CURVE_WITH_KNOTS('',3,(#146835,#146836,#146837,#146838,
#146839,#146840,#146841,#146842,#146843,#146844),.UNSPECIFIED.,.F.,.F.,
(4,2,2,2,4),(-0.678904071966622,-0.638811382082333,-0.567890404578333,-0.496948717476817,
-0.46642852082266),.UNSPECIFIED.);
#23829=B_SPLINE_CURVE_WITH_KNOTS('',3,(#146849,#146850,#146851,#146852,
#146853,#146854,#146855,#146856,#146857,#146858),.UNSPECIFIED.,.F.,.F.,
(4,2,2,2,4),(-0.678904071957464,-0.638811382081058,-0.567890404576504,-0.496948717474678,
-0.46642852082849),.UNSPECIFIED.);
#23830=B_SPLINE_CURVE_WITH_KNOTS('',3,(#146862,#146863,#146864,#146865,
#146866,#146867,#146868,#146869,#146870,#146871),.UNSPECIFIED.,.F.,.F.,
(4,2,2,2,4),(-0.678904071960602,-0.63881138208236,-0.567890404578389,-0.496948717476892,
-0.466428520828773),.UNSPECIFIED.);
#23831=B_SPLINE_CURVE_WITH_KNOTS('',3,(#146876,#146877,#146878,#146879,
#146880,#146881,#146882,#146883,#146884,#146885),.UNSPECIFIED.,.F.,.F.,
(4,2,2,2,4),(-0.678904071989264,-0.638811382079008,-0.567890404573618,-0.496948717471328,
-0.466428520791417),.UNSPECIFIED.);
#23832=B_SPLINE_CURVE_WITH_KNOTS('',3,(#146889,#146890,#146891,#146892,
#146893,#146894,#146895,#146896,#146897,#146898),.UNSPECIFIED.,.F.,.F.,
(4,2,2,2,4),(-0.678904071984124,-0.638811382082578,-0.567890404578774,-0.496948717477375,
-0.46642852080592),.UNSPECIFIED.);
#23833=B_SPLINE_CURVE_WITH_KNOTS('',3,(#146903,#146904,#146905,#146906,
#146907,#146908,#146909,#146910,#146911,#146912),.UNSPECIFIED.,.F.,.F.,
(4,2,2,2,4),(-0.678904071990912,-0.638811382078438,-0.567890404572854,-0.496948717470463,
-0.466428520788367),.UNSPECIFIED.);
#23834=B_SPLINE_CURVE_WITH_KNOTS('',3,(#146916,#146917,#146918,#146919,
#146920,#146921,#146922,#146923,#146924,#146925),.UNSPECIFIED.,.F.,.F.,
(4,2,2,2,4),(-0.67890407197895,-0.63881138207865,-0.567890404573101,-0.496948717470721,
-0.466428520800793),.UNSPECIFIED.);
#23835=B_SPLINE_CURVE_WITH_KNOTS('',3,(#146930,#146931,#146932,#146933,
#146934,#146935,#146936,#146937,#146938,#146939),.UNSPECIFIED.,.F.,.F.,
(4,2,2,2,4),(-0.67890407197844,-0.638811382081603,-0.567890404577301,-0.496948717475618,
-0.46642852078939),.UNSPECIFIED.);
#23836=B_SPLINE_CURVE_WITH_KNOTS('',3,(#146943,#146944,#146945,#146946,
#146947,#146948,#146949,#146950,#146951,#146952),.UNSPECIFIED.,.F.,.F.,
(4,2,2,2,4),(-0.678904071962693,-0.638811382079039,-0.567890404573721,-0.496948717471478,
-0.466428520818159),.UNSPECIFIED.);
#23837=B_SPLINE_CURVE_WITH_KNOTS('',3,(#146957,#146958,#146959,#146960,
#146961,#146962,#146963,#146964,#146965,#146966),.UNSPECIFIED.,.F.,.F.,
(4,2,2,2,4),(-0.678904071951875,-0.638811382081886,-0.56789040457777,-0.496948717476197,
-0.466428520836353),.UNSPECIFIED.);
#23838=B_SPLINE_CURVE_WITH_KNOTS('',3,(#146970,#146971,#146972,#146973,
#146974,#146975,#146976,#146977,#146978,#146979),.UNSPECIFIED.,.F.,.F.,
(4,2,2,2,4),(-0.678904071984224,-0.638811382077184,-0.567890404571044,-0.496948717468341,
-0.466428520791771),.UNSPECIFIED.);
#23839=B_SPLINE_CURVE_WITH_KNOTS('',3,(#146984,#146985,#146986,#146987,
#146988,#146989,#146990,#146991,#146992,#146993),.UNSPECIFIED.,.F.,.F.,
(4,2,2,2,4),(-0.678904071946679,-0.638811382083566,-0.567890404580102,-0.496948717478886,
-0.466428520817321),.UNSPECIFIED.);
#23840=B_SPLINE_CURVE_WITH_KNOTS('',3,(#146997,#146998,#146999,#147000,
#147001,#147002,#147003,#147004,#147005,#147006),.UNSPECIFIED.,.F.,.F.,
(4,2,2,2,4),(-0.678904071981425,-0.638811382080321,-0.567890404575443,-0.496948717473436,
-0.4664285208026),.UNSPECIFIED.);
#23841=B_SPLINE_CURVE_WITH_KNOTS('',3,(#147011,#147012,#147013,#147014,
#147015,#147016,#147017,#147018,#147019,#147020),.UNSPECIFIED.,.F.,.F.,
(4,2,2,2,4),(-0.678904071991316,-0.638811382081223,-0.567890404576789,-0.496948717475035,
-0.466428520807192),.UNSPECIFIED.);
#23842=B_SPLINE_CURVE_WITH_KNOTS('',3,(#147024,#147025,#147026,#147027,
#147028,#147029,#147030,#147031,#147032,#147033),.UNSPECIFIED.,.F.,.F.,
(4,2,2,2,4),(-0.678904071999418,-0.638811382081107,-0.567890404576574,-0.496948717474759,
-0.466428520786662),.UNSPECIFIED.);
#23843=B_SPLINE_CURVE_WITH_KNOTS('',3,(#147038,#147039,#147040,#147041,
#147042,#147043,#147044,#147045,#147046,#147047),.UNSPECIFIED.,.F.,.F.,
(4,2,2,2,4),(-0.678904071986371,-0.63881138208026,-0.567890404575494,-0.496948717473567,
-0.466428520797708),.UNSPECIFIED.);
#23844=B_SPLINE_CURVE_WITH_KNOTS('',3,(#147051,#147052,#147053,#147054,
#147055,#147056,#147057,#147058,#147059,#147060),.UNSPECIFIED.,.F.,.F.,
(4,2,2,2,4),(-0.678904071955908,-0.638811382081694,-0.56789040457745,-0.496948717475802,
-0.466428520793422),.UNSPECIFIED.);
#23845=B_SPLINE_CURVE_WITH_KNOTS('',3,(#147065,#147066,#147067,#147068,
#147069,#147070,#147071,#147072,#147073,#147074),.UNSPECIFIED.,.F.,.F.,
(4,2,2,2,4),(-0.678904071995711,-0.638811382080074,-0.567890404575169,-0.496948717473153,
-0.466428520827868),.UNSPECIFIED.);
#23846=B_SPLINE_CURVE_WITH_KNOTS('',3,(#147078,#147079,#147080,#147081,
#147082,#147083,#147084,#147085,#147086,#147087),.UNSPECIFIED.,.F.,.F.,
(4,2,2,2,4),(-0.6789040719681,-0.638811382078021,-0.567890404572175,-0.496948717469627,
-0.466428520809968),.UNSPECIFIED.);
#23847=B_SPLINE_CURVE_WITH_KNOTS('',3,(#147092,#147093,#147094,#147095,
#147096,#147097,#147098,#147099,#147100,#147101),.UNSPECIFIED.,.F.,.F.,
(4,2,2,2,4),(-0.678904071991019,-0.638811382084413,-0.567890404581332,-0.496948717480334,
-0.466428520838104),.UNSPECIFIED.);
#23848=B_SPLINE_CURVE_WITH_KNOTS('',3,(#147105,#147106,#147107,#147108,
#147109,#147110,#147111,#147112,#147113,#147114),.UNSPECIFIED.,.F.,.F.,
(4,2,2,2,4),(-0.678904072013258,-0.638811382084341,-0.567890404581218,-0.496948717480194,
-0.466428520827364),.UNSPECIFIED.);
#23849=B_SPLINE_CURVE_WITH_KNOTS('',3,(#147119,#147120,#147121,#147122,
#147123,#147124,#147125,#147126,#147127,#147128),.UNSPECIFIED.,.F.,.F.,
(4,2,2,2,4),(-0.678904071985943,-0.638811382076362,-0.567890404569934,-0.496948717467075,
-0.466428520788006),.UNSPECIFIED.);
#23850=B_SPLINE_CURVE_WITH_KNOTS('',3,(#147132,#147133,#147134,#147135,
#147136,#147137,#147138,#147139,#147140,#147141),.UNSPECIFIED.,.F.,.F.,
(4,2,2,2,4),(-0.678904071993597,-0.63881138208345,-0.567890404579917,-0.49694871747866,
-0.466428520817712),.UNSPECIFIED.);
#23851=B_SPLINE_CURVE_WITH_KNOTS('',3,(#147146,#147147,#147148,#147149,
#147150,#147151,#147152,#147153,#147154,#147155),.UNSPECIFIED.,.F.,.F.,
(4,2,2,2,4),(-0.678904071973235,-0.638811382076413,-0.567890404569979,-0.496948717467112,
-0.466428520774701),.UNSPECIFIED.);
#23852=B_SPLINE_CURVE_WITH_KNOTS('',3,(#147159,#147160,#147161,#147162,
#147163,#147164,#147165,#147166,#147167,#147168),.UNSPECIFIED.,.F.,.F.,
(4,2,2,2,4),(-0.67890407198703,-0.638811382078511,-0.567890404572937,-0.496948717470548,
-0.46642852084323),.UNSPECIFIED.);
#23853=B_SPLINE_CURVE_WITH_KNOTS('',3,(#147173,#147174,#147175,#147176,
#147177,#147178,#147179,#147180,#147181,#147182),.UNSPECIFIED.,.F.,.F.,
(4,2,2,2,4),(-0.678904071987918,-0.63881138208419,-0.567890404580971,-0.496948717479887,
-0.466428520806156),.UNSPECIFIED.);
#23854=B_SPLINE_CURVE_WITH_KNOTS('',3,(#147186,#147187,#147188,#147189,
#147190,#147191,#147192,#147193,#147194,#147195),.UNSPECIFIED.,.F.,.F.,
(4,2,2,2,4),(-0.678904072009243,-0.638811382083172,-0.567890404579565,-0.496948717478273,
-0.466428520834842),.UNSPECIFIED.);
#23855=B_SPLINE_CURVE_WITH_KNOTS('',3,(#147200,#147201,#147202,#147203,
#147204,#147205,#147206,#147207,#147208,#147209),.UNSPECIFIED.,.F.,.F.,
(4,2,2,2,4),(-0.678904071972171,-0.638811382079603,-0.567890404574478,-0.496948717472339,
-0.466428520810079),.UNSPECIFIED.);
#23856=B_SPLINE_CURVE_WITH_KNOTS('',3,(#147213,#147214,#147215,#147216,
#147217,#147218,#147219,#147220,#147221,#147222),.UNSPECIFIED.,.F.,.F.,
(4,2,2,2,4),(-0.67890407197948,-0.63881138208111,-0.567890404576586,-0.496948717474778,
-0.466428520794178),.UNSPECIFIED.);
#23857=B_SPLINE_CURVE_WITH_KNOTS('',3,(#147227,#147228,#147229,#147230,
#147231,#147232,#147233,#147234,#147235,#147236),.UNSPECIFIED.,.F.,.F.,
(4,2,2,2,4),(-0.67890407199919,-0.638811382081417,-0.567890404577054,-0.496948717475335,
-0.466428520787747),.UNSPECIFIED.);
#23858=B_SPLINE_CURVE_WITH_KNOTS('',3,(#147240,#147241,#147242,#147243,
#147244,#147245,#147246,#147247,#147248,#147249),.UNSPECIFIED.,.F.,.F.,
(4,2,2,2,4),(-0.678904071953487,-0.638811382080193,-0.567890404575326,-0.496948717473333,
-0.466428520830309),.UNSPECIFIED.);
#23859=B_SPLINE_CURVE_WITH_KNOTS('',3,(#147254,#147255,#147256,#147257,
#147258,#147259,#147260,#147261,#147262,#147263),.UNSPECIFIED.,.F.,.F.,
(4,2,2,2,4),(-0.678904072000796,-0.638811382081297,-0.567890404576874,-0.496948717475125,
-0.466428520785821),.UNSPECIFIED.);
#23860=B_SPLINE_CURVE_WITH_KNOTS('',3,(#147267,#147268,#147269,#147270,
#147271,#147272,#147273,#147274,#147275,#147276),.UNSPECIFIED.,.F.,.F.,
(4,2,2,2,4),(-0.678904071991668,-0.638811382082854,-0.567890404579058,-0.496948717477653,
-0.466428520798932),.UNSPECIFIED.);
#23861=B_SPLINE_CURVE_WITH_KNOTS('',3,(#147281,#147282,#147283,#147284,
#147285,#147286,#147287,#147288,#147289,#147290),.UNSPECIFIED.,.F.,.F.,
(4,2,2,2,4),(-0.678904071964471,-0.638811382077228,-0.567890404571169,-0.496948717468516,
-0.466428520811726),.UNSPECIFIED.);
#23862=B_SPLINE_CURVE_WITH_KNOTS('',3,(#147294,#147295,#147296,#147297,
#147298,#147299,#147300,#147301,#147302,#147303),.UNSPECIFIED.,.F.,.F.,
(4,2,2,2,4),(-0.678904071968841,-0.638811382079846,-0.567890404574781,-0.496948717472671,
-0.466428520813977),.UNSPECIFIED.);
#23863=B_SPLINE_CURVE_WITH_KNOTS('',3,(#147308,#147309,#147310,#147311,
#147312,#147313,#147314,#147315,#147316,#147317),.UNSPECIFIED.,.F.,.F.,
(4,2,2,2,4),(-0.678904071990042,-0.638811382082262,-0.567890404578158,-0.496948717476576,
-0.466428520798937),.UNSPECIFIED.);
#23864=B_SPLINE_CURVE_WITH_KNOTS('',3,(#147321,#147322,#147323,#147324,
#147325,#147326,#147327,#147328,#147329,#147330),.UNSPECIFIED.,.F.,.F.,
(4,2,2,2,4),(-0.678904072003725,-0.638811382081756,-0.567890404577507,-0.496948717475853,
-0.466428520791346),.UNSPECIFIED.);
#23865=B_SPLINE_CURVE_WITH_KNOTS('',3,(#147335,#147336,#147337,#147338,
#147339,#147340,#147341,#147342,#147343,#147344),.UNSPECIFIED.,.F.,.F.,
(4,2,2,2,4),(-0.678904071951667,-0.638811382079402,-0.567890404574249,-0.4969487174721,
-0.466428520830143),.UNSPECIFIED.);
#23866=B_SPLINE_CURVE_WITH_KNOTS('',3,(#147348,#147349,#147350,#147351,
#147352,#147353,#147354,#147355,#147356,#147357),.UNSPECIFIED.,.F.,.F.,
(4,2,2,2,4),(-0.678904071999203,-0.638811382080604,-0.567890404575878,-0.496948717473956,
-0.466428520785595),.UNSPECIFIED.);
#23867=B_SPLINE_CURVE_WITH_KNOTS('',3,(#147362,#147363,#147364,#147365,
#147366,#147367,#147368,#147369,#147370,#147371),.UNSPECIFIED.,.F.,.F.,
(4,2,2,2,4),(-0.678904071974462,-0.638811382079151,-0.567890404573839,-0.496948717471593,
-0.466428520806612),.UNSPECIFIED.);
#23868=B_SPLINE_CURVE_WITH_KNOTS('',3,(#147375,#147376,#147377,#147378,
#147379,#147380,#147381,#147382,#147383,#147384),.UNSPECIFIED.,.F.,.F.,
(4,2,2,2,4),(-0.678904071970275,-0.638811382078786,-0.567890404573214,-0.496948717470815,
-0.466428520809705),.UNSPECIFIED.);
#23869=B_SPLINE_CURVE_WITH_KNOTS('',3,(#147389,#147390,#147391,#147392,
#147393,#147394,#147395,#147396,#147397,#147398),.UNSPECIFIED.,.F.,.F.,
(4,2,2,2,4),(-0.678904071989522,-0.638811382082555,-0.567890404578647,-0.496948717477185,
-0.466428520800335),.UNSPECIFIED.);
#23870=B_SPLINE_CURVE_WITH_KNOTS('',3,(#147402,#147403,#147404,#147405,
#147406,#147407,#147408,#147409,#147410,#147411),.UNSPECIFIED.,.F.,.F.,
(4,2,2,2,4),(-0.678904071985921,-0.638811382083359,-0.56789040457979,-0.496948717478515,
-0.466428520806011),.UNSPECIFIED.);
#23871=B_SPLINE_CURVE_WITH_KNOTS('',3,(#147416,#147417,#147418,#147419,
#147420,#147421,#147422,#147423,#147424,#147425),.UNSPECIFIED.,.F.,.F.,
(4,2,2,2,4),(-0.678904071977173,-0.63881138207607,-0.567890404569492,-0.496948717466546,
-0.466428520814141),.UNSPECIFIED.);
#23872=B_SPLINE_CURVE_WITH_KNOTS('',3,(#147429,#147430,#147431,#147432,
#147433,#147434,#147435,#147436,#147437,#147438),.UNSPECIFIED.,.F.,.F.,
(4,2,2,2,4),(-0.678904071975169,-0.63881138207716,-0.567890404571027,-0.496948717468329,
-0.466428520800785),.UNSPECIFIED.);
#23873=B_SPLINE_CURVE_WITH_KNOTS('',3,(#147443,#147444,#147445,#147446,
#147447,#147448,#147449,#147450,#147451,#147452),.UNSPECIFIED.,.F.,.F.,
(4,2,2,2,4),(-0.67890407194793,-0.638811382083603,-0.567890404580231,-0.496948717479076,
-0.466428520818441),.UNSPECIFIED.);
#23874=B_SPLINE_CURVE_WITH_KNOTS('',3,(#147456,#147457,#147458,#147459,
#147460,#147461,#147462,#147463,#147464,#147465),.UNSPECIFIED.,.F.,.F.,
(4,2,2,2,4),(-0.678904071957711,-0.638811382077597,-0.567890404571664,-0.496948717469078,
-0.466428520789034),.UNSPECIFIED.);
#23875=B_SPLINE_CURVE_WITH_KNOTS('',3,(#147470,#147471,#147472,#147473,
#147474,#147475,#147476,#147477,#147478,#147479),.UNSPECIFIED.,.F.,.F.,
(4,2,2,2,4),(-0.678904071980114,-0.638811382084221,-0.567890404581019,-0.496948717479949,
-0.46642852081406),.UNSPECIFIED.);
#23876=B_SPLINE_CURVE_WITH_KNOTS('',3,(#147483,#147484,#147485,#147486,
#147487,#147488,#147489,#147490,#147491,#147492),.UNSPECIFIED.,.F.,.F.,
(4,2,2,2,4),(-0.678904071988688,-0.638811382083351,-0.567890404579804,-0.496948717478542,
-0.466428520803256),.UNSPECIFIED.);
#23877=B_SPLINE_CURVE_WITH_KNOTS('',3,(#147497,#147498,#147499,#147500,
#147501,#147502,#147503,#147504,#147505,#147506),.UNSPECIFIED.,.F.,.F.,
(4,2,2,2,4),(-0.678904071967103,-0.638811382077954,-0.567890404572145,-0.496948717469628,
-0.466428520802325),.UNSPECIFIED.);
#23878=B_SPLINE_CURVE_WITH_KNOTS('',3,(#147510,#147511,#147512,#147513,
#147514,#147515,#147516,#147517,#147518,#147519),.UNSPECIFIED.,.F.,.F.,
(4,2,2,2,4),(-0.678904071996367,-0.638811382079977,-0.567890404575077,-0.496948717473068,
-0.466428520786947),.UNSPECIFIED.);
#23879=B_SPLINE_CURVE_WITH_KNOTS('',3,(#147524,#147525,#147526,#147527,
#147528,#147529,#147530,#147531,#147532,#147533),.UNSPECIFIED.,.F.,.F.,
(4,2,2,2,4),(-0.678904071994096,-0.6388113820812,-0.567890404576721,-0.496948717474939,
-0.466428520832143),.UNSPECIFIED.);
#23880=B_SPLINE_CURVE_WITH_KNOTS('',3,(#147537,#147538,#147539,#147540,
#147541,#147542,#147543,#147544,#147545,#147546),.UNSPECIFIED.,.F.,.F.,
(4,2,2,2,4),(-0.678904071987513,-0.638811382080565,-0.567890404575855,-0.496948717473948,
-0.46642852079724),.UNSPECIFIED.);
#23881=B_SPLINE_CURVE_WITH_KNOTS('',3,(#147551,#147552,#147553,#147554,
#147555,#147556,#147557,#147558,#147559,#147560),.UNSPECIFIED.,.F.,.F.,
(4,2,2,2,4),(-0.678904071998105,-0.638811382080726,-0.567890404576089,-0.496948717474222,
-0.466428520787071),.UNSPECIFIED.);
#23882=B_SPLINE_CURVE_WITH_KNOTS('',3,(#147564,#147565,#147566,#147567,
#147568,#147569,#147570,#147571,#147572,#147573),.UNSPECIFIED.,.F.,.F.,
(4,2,2,2,4),(-0.678904071978989,-0.6388113820818,-0.567890404577646,-0.496948717476053,
-0.466428520806628),.UNSPECIFIED.);
#23883=B_SPLINE_CURVE_WITH_KNOTS('',3,(#147578,#147579,#147580,#147581,
#147582,#147583,#147584,#147585,#147586,#147587),.UNSPECIFIED.,.F.,.F.,
(4,2,2,2,4),(-0.678904072012599,-0.638811382080154,-0.56789040457528,-0.496948717473282,
-0.466428520771101),.UNSPECIFIED.);
#23884=B_SPLINE_CURVE_WITH_KNOTS('',3,(#147591,#147592,#147593,#147594,
#147595,#147596,#147597,#147598,#147599,#147600),.UNSPECIFIED.,.F.,.F.,
(4,2,2,2,4),(-0.678904071978745,-0.638811382085293,-0.567890404582573,-0.496948717481774,
-0.466428520818246),.UNSPECIFIED.);
#23885=B_SPLINE_CURVE_WITH_KNOTS('',3,(#147605,#147606,#147607,#147608,
#147609,#147610,#147611,#147612,#147613,#147614),.UNSPECIFIED.,.F.,.F.,
(4,2,2,2,4),(-0.678904071984472,-0.638811382077059,-0.567890404570888,-0.496948717468167,
-0.466428520791229),.UNSPECIFIED.);
#23886=B_SPLINE_CURVE_WITH_KNOTS('',3,(#147618,#147619,#147620,#147621,
#147622,#147623,#147624,#147625,#147626,#147627),.UNSPECIFIED.,.F.,.F.,
(4,2,2,2,4),(-0.678904072000963,-0.638811382081332,-0.567890404576933,-0.496948717475197,
-0.466428520835545),.UNSPECIFIED.);
#23887=B_SPLINE_CURVE_WITH_KNOTS('',3,(#147632,#147633,#147634,#147635,
#147636,#147637,#147638,#147639,#147640,#147641),.UNSPECIFIED.,.F.,.F.,
(4,2,2,2,4),(-0.678904071963139,-0.63881138207992,-0.567890404574934,-0.496948717472875,
-0.466428520819943),.UNSPECIFIED.);
#23888=B_SPLINE_CURVE_WITH_KNOTS('',3,(#147645,#147646,#147647,#147648,
#147649,#147650,#147651,#147652,#147653,#147654),.UNSPECIFIED.,.F.,.F.,
(4,2,2,2,4),(-0.678904071978786,-0.638811382081839,-0.567890404577663,-0.496948717476051,
-0.466428520809257),.UNSPECIFIED.);
#23889=B_SPLINE_CURVE_WITH_KNOTS('',3,(#147659,#147660,#147661,#147662,
#147663,#147664,#147665,#147666,#147667,#147668),.UNSPECIFIED.,.F.,.F.,
(4,2,2,2,4),(-0.678904071979581,-0.638811382078899,-0.567890404573514,-0.496948717471234,
-0.466428520800896),.UNSPECIFIED.);
#23890=B_SPLINE_CURVE_WITH_KNOTS('',3,(#147672,#147673,#147674,#147675,
#147676,#147677,#147678,#147679,#147680,#147681),.UNSPECIFIED.,.F.,.F.,
(4,2,2,2,4),(-0.6789040719931,-0.638811382079555,-0.567890404574399,-0.496948717472244,
-0.466428520789016),.UNSPECIFIED.);
#23891=B_SPLINE_CURVE_WITH_KNOTS('',3,(#147686,#147687,#147688,#147689,
#147690,#147691,#147692,#147693,#147694,#147695),.UNSPECIFIED.,.F.,.F.,
(4,2,2,2,4),(-0.678904071996576,-0.63881138208247,-0.567890404578552,-0.496948717477086,
-0.466428520807683),.UNSPECIFIED.);
#23892=B_SPLINE_CURVE_WITH_KNOTS('',3,(#147699,#147700,#147701,#147702,
#147703,#147704,#147705,#147706,#147707,#147708),.UNSPECIFIED.,.F.,.F.,
(4,2,2,2,4),(-0.678904071992612,-0.638811382080339,-0.567890404575539,-0.496948717473582,
-0.466428520781553),.UNSPECIFIED.);
#23893=B_SPLINE_CURVE_WITH_KNOTS('',3,(#147713,#147714,#147715,#147716,
#147717,#147718,#147719,#147720,#147721,#147722),.UNSPECIFIED.,.F.,.F.,
(4,2,2,2,4),(-0.678904071957699,-0.638811382081068,-0.567890404576578,-0.496948717474793,
-0.466428520828367),.UNSPECIFIED.);
#23894=B_SPLINE_CURVE_WITH_KNOTS('',3,(#147726,#147727,#147728,#147729,
#147730,#147731,#147732,#147733,#147734,#147735),.UNSPECIFIED.,.F.,.F.,
(4,2,2,2,4),(-0.678904071955071,-0.638811382079537,-0.567890404574392,-0.496948717472241,
-0.466428520827014),.UNSPECIFIED.);
#23895=B_SPLINE_CURVE_WITH_KNOTS('',3,(#147740,#147741,#147742,#147743,
#147744,#147745,#147746,#147747,#147748,#147749),.UNSPECIFIED.,.F.,.F.,
(4,2,2,2,4),(-0.678904071963275,-0.638811382080631,-0.567890404575947,-0.496948717474053,
-0.466428520821643),.UNSPECIFIED.);
#23896=B_SPLINE_CURVE_WITH_KNOTS('',3,(#147753,#147754,#147755,#147756,
#147757,#147758,#147759,#147760,#147761,#147762),.UNSPECIFIED.,.F.,.F.,
(4,2,2,2,4),(-0.678904071975039,-0.638811382079947,-0.567890404574985,-0.496948717472938,
-0.466428520808125),.UNSPECIFIED.);
#23897=B_SPLINE_CURVE_WITH_KNOTS('',3,(#147829,#147830,#147831,#147832,
#147833,#147834,#147835,#147836,#147837,#147838,#147839,#147840,#147841,
#147842,#147843,#147844,#147845),.UNSPECIFIED.,.F.,.F.,(4,2,2,3,2,2,2,4),
(-0.0105482508477054,-0.00774017959540533,-0.00385609988520743,0.,0.00219233319325163,
0.00438738203112965,0.0083182289718649,0.0105383937687012),
 .UNSPECIFIED.);
#23898=B_SPLINE_CURVE_WITH_KNOTS('',3,(#147846,#147847,#147848,#147849),
 .UNSPECIFIED.,.F.,.F.,(4,4),(2.06733813101515,2.11814920351283),
 .UNSPECIFIED.);
#23899=B_SPLINE_CURVE_WITH_KNOTS('',3,(#147851,#147852,#147853,#147854),
 .UNSPECIFIED.,.F.,.F.,(4,4),(3.73816266103403,3.78897373354396),
 .UNSPECIFIED.);
#23900=B_SPLINE_CURVE_WITH_KNOTS('',3,(#147856,#147857,#147858,#147859,
#147860,#147861,#147862,#147863,#147864,#147865,#147866,#147867,#147868,
#147869,#147870,#147871,#147872),.UNSPECIFIED.,.F.,.F.,(4,2,2,2,3,2,2,4),
(0.0529024353036734,0.0551226000958153,0.0590534470366397,0.0612484958745396,
0.0634408290678051,0.0672969289529751,0.0711810086631009,0.0739890798907039),
 .UNSPECIFIED.);
#23901=B_SPLINE_CURVE_WITH_KNOTS('',3,(#147873,#147874,#147875,#147876),
 .UNSPECIFIED.,.F.,.F.,(4,4),(2.06733813100459,2.11814920352257),
 .UNSPECIFIED.);
#23902=B_SPLINE_CURVE_WITH_KNOTS('',3,(#147878,#147879,#147880,#147881),
 .UNSPECIFIED.,.F.,.F.,(4,4),(3.73816266106249,3.78897373354877),
 .UNSPECIFIED.);
#23903=B_SPLINE_CURVE_WITH_KNOTS('',3,(#147883,#147884,#147885,#147886,
#147887,#147888,#147889,#147890,#147891,#147892,#147893,#147894,#147895,
#147896,#147897,#147898,#147899),.UNSPECIFIED.,.F.,.F.,(4,2,2,2,3,2,2,4),
(0.0529024352792957,0.0551226000955082,0.0590534470363172,0.0612484958742291,
0.0634408290675084,0.067296928952713,0.0711810086628562,0.0739890798962668),
 .UNSPECIFIED.);
#23904=B_SPLINE_CURVE_WITH_KNOTS('',3,(#147900,#147901,#147902,#147903),
 .UNSPECIFIED.,.F.,.F.,(4,4),(2.06733813090294,2.11814920352042),
 .UNSPECIFIED.);
#23905=B_SPLINE_CURVE_WITH_KNOTS('',3,(#147905,#147906,#147907,#147908),
 .UNSPECIFIED.,.F.,.F.,(4,4),(3.73816266145575,3.78897373392225),
 .UNSPECIFIED.);
#23906=B_SPLINE_CURVE_WITH_KNOTS('',3,(#147910,#147911,#147912,#147913,
#147914,#147915,#147916,#147917,#147918,#147919,#147920,#147921,#147922,
#147923,#147924,#147925,#147926),.UNSPECIFIED.,.F.,.F.,(4,2,2,2,3,2,2,4),
(0.0529024352448051,0.0551226000948243,0.0590534470358053,0.0612484958738077,
0.0634408290671648,0.067296928952395,0.0711810086624211,0.0739890799479556),
 .UNSPECIFIED.);
#23907=B_SPLINE_CURVE_WITH_KNOTS('',3,(#147927,#147928,#147929,#147930),
 .UNSPECIFIED.,.F.,.F.,(4,4),(2.06733813079829,2.11814920332747),
 .UNSPECIFIED.);
#23908=B_SPLINE_CURVE_WITH_KNOTS('',3,(#147932,#147933,#147934,#147935),
 .UNSPECIFIED.,.F.,.F.,(4,4),(3.7381626605244,3.78897373310771),
 .UNSPECIFIED.);
#23909=B_SPLINE_CURVE_WITH_KNOTS('',3,(#147937,#147938,#147939,#147940,
#147941,#147942,#147943,#147944,#147945,#147946,#147947,#147948,#147949,
#147950,#147951,#147952,#147953),.UNSPECIFIED.,.F.,.F.,(4,2,2,2,3,2,2,4),
(0.0529024352696854,0.0551226000951222,0.0590534470356417,0.0612484958734864,
0.063440829066722,0.0672969289520468,0.0711810086624219,0.0739890799428532),
 .UNSPECIFIED.);
#23910=B_SPLINE_CURVE_WITH_KNOTS('',3,(#147954,#147955,#147956,#147957),
 .UNSPECIFIED.,.F.,.F.,(4,4),(2.06733813108993,2.11814920359329),
 .UNSPECIFIED.);
#23911=B_SPLINE_CURVE_WITH_KNOTS('',3,(#147959,#147960,#147961,#147962),
 .UNSPECIFIED.,.F.,.F.,(4,4),(3.73816266065588,3.7889737331094),
 .UNSPECIFIED.);
#23912=B_SPLINE_CURVE_WITH_KNOTS('',3,(#147964,#147965,#147966,#147967,
#147968,#147969,#147970,#147971,#147972,#147973,#147974,#147975,#147976,
#147977,#147978,#147979,#147980),.UNSPECIFIED.,.F.,.F.,(4,2,2,2,3,2,2,4),
(0.0529024352500414,0.0551226000953574,0.0590534470359871,0.0612484958738545,
0.0634408290671024,0.0672969289523756,0.0711810086626638,0.073989079946815),
 .UNSPECIFIED.);
#23913=B_SPLINE_CURVE_WITH_KNOTS('',3,(#147981,#147982,#147983,#147984),
 .UNSPECIFIED.,.F.,.F.,(4,4),(2.06733813108585,2.1181492035795),
 .UNSPECIFIED.);
#23914=B_SPLINE_CURVE_WITH_KNOTS('',3,(#147986,#147987,#147988,#147989),
 .UNSPECIFIED.,.F.,.F.,(4,4),(3.73816265997327,3.78897373253894),
 .UNSPECIFIED.);
#23915=B_SPLINE_CURVE_WITH_KNOTS('',3,(#147991,#147992,#147993,#147994,
#147995,#147996,#147997,#147998,#147999,#148000,#148001,#148002,#148003,
#148004,#148005,#148006,#148007),.UNSPECIFIED.,.F.,.F.,(4,2,2,2,3,2,2,4),
(0.0529024352877033,0.055122600096207,0.0590534470365002,0.061248495874216,
0.063440829067339,0.0672969289526178,0.0711810086631494,0.0739890799430888),
 .UNSPECIFIED.);
#23916=B_SPLINE_CURVE_WITH_KNOTS('',3,(#148008,#148009,#148010,#148011),
 .UNSPECIFIED.,.F.,.F.,(4,4),(2.06733813118465,2.11814920367701),
 .UNSPECIFIED.);
#23917=B_SPLINE_CURVE_WITH_KNOTS('',3,(#148013,#148014,#148015,#148016),
 .UNSPECIFIED.,.F.,.F.,(4,4),(3.73816266083586,3.78897373340649),
 .UNSPECIFIED.);
#23918=B_SPLINE_CURVE_WITH_KNOTS('',3,(#148018,#148019,#148020,#148021,
#148022,#148023,#148024,#148025,#148026,#148027,#148028,#148029,#148030,
#148031,#148032,#148033,#148034),.UNSPECIFIED.,.F.,.F.,(4,2,2,2,3,2,2,4),
(0.0529024353274146,0.0551226000958684,0.0590534470366202,0.0612484958744934,
0.063440829067739,0.0672969289529286,0.071181008663116,0.0739890799286134),
 .UNSPECIFIED.);
#23919=B_SPLINE_CURVE_WITH_KNOTS('',3,(#148035,#148036,#148037,#148038),
 .UNSPECIFIED.,.F.,.F.,(4,4),(2.06733813097796,2.11814920353602),
 .UNSPECIFIED.);
#23920=B_SPLINE_CURVE_WITH_KNOTS('',3,(#148040,#148041,#148042,#148043),
 .UNSPECIFIED.,.F.,.F.,(4,4),(3.73816266096225,3.78897373348547),
 .UNSPECIFIED.);
#23921=B_SPLINE_CURVE_WITH_KNOTS('',3,(#148045,#148046,#148047,#148048,
#148049,#148050,#148051,#148052,#148053,#148054,#148055,#148056,#148057,
#148058,#148059,#148060,#148061),.UNSPECIFIED.,.F.,.F.,(4,2,2,2,3,2,2,4),
(0.0529024352352074,0.0551226000951276,0.0590534470358563,0.0612484958737609,
0.0634408290670414,0.067296928952303,0.0711810086625111,0.073989079927302),
 .UNSPECIFIED.);
#23922=B_SPLINE_CURVE_WITH_KNOTS('',3,(#148062,#148063,#148064,#148065),
 .UNSPECIFIED.,.F.,.F.,(4,4),(2.06733813095919,2.11814920352003),
 .UNSPECIFIED.);
#23923=B_SPLINE_CURVE_WITH_KNOTS('',3,(#148067,#148068,#148069,#148070),
 .UNSPECIFIED.,.F.,.F.,(4,4),(3.73816266110557,3.78897373362394),
 .UNSPECIFIED.);
#23924=B_SPLINE_CURVE_WITH_KNOTS('',3,(#148072,#148073,#148074,#148075,
#148076,#148077,#148078,#148079,#148080,#148081,#148082,#148083,#148084,
#148085,#148086,#148087,#148088),.UNSPECIFIED.,.F.,.F.,(4,2,2,2,3,2,2,4),
(0.0529024352526763,0.0551226000943946,0.0590534470351668,0.0612484958731182,
0.0634408290664451,0.0672969289517592,0.0711810086619386,0.0739890799932635),
 .UNSPECIFIED.);
#23925=B_SPLINE_CURVE_WITH_KNOTS('',3,(#148089,#148090,#148091,#148092),
 .UNSPECIFIED.,.F.,.F.,(4,4),(2.06733813088428,2.11814920342807),
 .UNSPECIFIED.);
#23926=B_SPLINE_CURVE_WITH_KNOTS('',3,(#148094,#148095,#148096,#148097),
 .UNSPECIFIED.,.F.,.F.,(4,4),(3.73816266018992,3.78897373275654),
 .UNSPECIFIED.);
#23927=B_SPLINE_CURVE_WITH_KNOTS('',3,(#148099,#148100,#148101,#148102,
#148103,#148104,#148105,#148106,#148107,#148108,#148109,#148110,#148111,
#148112,#148113,#148114,#148115),.UNSPECIFIED.,.F.,.F.,(4,2,2,2,3,2,2,4),
(0.0529024352594984,0.0551226000959426,0.0590534470363031,0.0612484958740503,
0.0634408290672013,0.0672969289524806,0.0711810086629572,0.0739890799144632),
 .UNSPECIFIED.);
#23928=B_SPLINE_CURVE_WITH_KNOTS('',3,(#148116,#148117,#148118,#148119),
 .UNSPECIFIED.,.F.,.F.,(4,4),(2.06733813112861,2.11814920361968),
 .UNSPECIFIED.);
#23929=B_SPLINE_CURVE_WITH_KNOTS('',3,(#148121,#148122,#148123,#148124),
 .UNSPECIFIED.,.F.,.F.,(4,4),(3.7381626617959,3.78897373426471),
 .UNSPECIFIED.);
#23930=B_SPLINE_CURVE_WITH_KNOTS('',3,(#148126,#148127,#148128,#148129,
#148130,#148131,#148132,#148133,#148134,#148135,#148136,#148137,#148138,
#148139,#148140,#148141,#148142),.UNSPECIFIED.,.F.,.F.,(4,2,2,2,3,2,2,4),
(0.0529024352876146,0.055122600094267,0.0590534470354298,0.0612484958735101,
0.0634408290669359,0.067296928952156,0.0711810086620328,0.0739890800128771),
 .UNSPECIFIED.);
#23931=B_SPLINE_CURVE_WITH_KNOTS('',3,(#148143,#148144,#148145,#148146),
 .UNSPECIFIED.,.F.,.F.,(4,4),(2.06733813072275,2.11814920323567),
 .UNSPECIFIED.);
#23932=B_SPLINE_CURVE_WITH_KNOTS('',3,(#148148,#148149,#148150,#148151),
 .UNSPECIFIED.,.F.,.F.,(4,4),(3.73816266167531,3.78897373415517),
 .UNSPECIFIED.);
#23933=B_SPLINE_CURVE_WITH_KNOTS('',3,(#148153,#148154,#148155,#148156,
#148157,#148158,#148159,#148160,#148161,#148162,#148163,#148164,#148165,
#148166,#148167,#148168,#148169),.UNSPECIFIED.,.F.,.F.,(4,2,2,2,3,2,2,4),
(0.0529024353277011,0.0551226000949243,0.0590534470360282,0.0612484958740575,
0.0634408290674342,0.0672969289526096,0.0711810086625277,0.0739890799254628),
 .UNSPECIFIED.);
#23934=B_SPLINE_CURVE_WITH_KNOTS('',3,(#148170,#148171,#148172,#148173),
 .UNSPECIFIED.,.F.,.F.,(4,4),(2.06733813079588,2.11814920335918),
 .UNSPECIFIED.);
#23935=B_SPLINE_CURVE_WITH_KNOTS('',3,(#148175,#148176,#148177,#148178),
 .UNSPECIFIED.,.F.,.F.,(4,4),(3.73816265995722,3.78897373248134),
 .UNSPECIFIED.);
#23936=B_SPLINE_CURVE_WITH_KNOTS('',3,(#148180,#148181,#148182,#148183,
#148184,#148185,#148186,#148187,#148188,#148189,#148190,#148191,#148192,
#148193,#148194,#148195,#148196),.UNSPECIFIED.,.F.,.F.,(4,2,2,2,3,2,2,4),
(0.0529024352480456,0.0551226000967675,0.0590534470371181,0.0612484958748231,
0.0634408290679309,0.0672969289531626,0.0711810086636647,0.0739890798763888),
 .UNSPECIFIED.);
#23937=B_SPLINE_CURVE_WITH_KNOTS('',3,(#148197,#148198,#148199,#148200),
 .UNSPECIFIED.,.F.,.F.,(4,4),(2.0673381312259,2.11814920375009),
 .UNSPECIFIED.);
#23938=B_SPLINE_CURVE_WITH_KNOTS('',3,(#148202,#148203,#148204,#148205),
 .UNSPECIFIED.,.F.,.F.,(4,4),(3.73816266135447,3.78897373388667),
 .UNSPECIFIED.);
#23939=B_SPLINE_CURVE_WITH_KNOTS('',3,(#148207,#148208,#148209,#148210,
#148211,#148212,#148213,#148214,#148215,#148216,#148217,#148218,#148219,
#148220,#148221,#148222,#148223),.UNSPECIFIED.,.F.,.F.,(4,2,2,2,3,2,2,4),
(0.0529024352811202,0.055122600094669,0.0590534470355693,0.0612484958735547,
0.0634408290669023,0.0672969289521659,0.0711810086622503,0.0739890799314381),
 .UNSPECIFIED.);
#23940=B_SPLINE_CURVE_WITH_KNOTS('',3,(#148224,#148225,#148226,#148227),
 .UNSPECIFIED.,.F.,.F.,(4,4),(2.06733813088284,2.11814920343982),
 .UNSPECIFIED.);
#23941=B_SPLINE_CURVE_WITH_KNOTS('',3,(#148229,#148230,#148231,#148232),
 .UNSPECIFIED.,.F.,.F.,(4,4),(3.73816266067428,3.78897373321881),
 .UNSPECIFIED.);
#23942=B_SPLINE_CURVE_WITH_KNOTS('',3,(#148234,#148235,#148236,#148237,
#148238,#148239,#148240,#148241,#148242,#148243,#148244,#148245,#148246,
#148247,#148248,#148249,#148250),.UNSPECIFIED.,.F.,.F.,(4,2,2,2,3,2,2,4),
(0.052902435264904,0.0551226000944819,0.0590534470351052,0.0612484958730058,
0.0634408290662948,0.0672969289516403,0.0711810086619305,0.0739890800019837),
 .UNSPECIFIED.);
#23943=B_SPLINE_CURVE_WITH_KNOTS('',3,(#148251,#148252,#148253,#148254),
 .UNSPECIFIED.,.F.,.F.,(4,4),(2.06733813102832,2.11814920355794),
 .UNSPECIFIED.);
#23944=B_SPLINE_CURVE_WITH_KNOTS('',3,(#148256,#148257,#148258,#148259),
 .UNSPECIFIED.,.F.,.F.,(4,4),(3.73816266066757,3.78897373314875),
 .UNSPECIFIED.);
#23945=B_SPLINE_CURVE_WITH_KNOTS('',3,(#148261,#148262,#148263,#148264,
#148265,#148266,#148267,#148268,#148269,#148270,#148271,#148272,#148273,
#148274,#148275,#148276,#148277),.UNSPECIFIED.,.F.,.F.,(4,2,2,2,3,2,2,4),
(0.052902435234979,0.0551226000954227,0.0590534470359989,0.0612484958738436,
0.063440829067074,0.067296928952351,0.0711810086626759,0.0739890799320362),
 .UNSPECIFIED.);
#23946=B_SPLINE_CURVE_WITH_KNOTS('',3,(#148278,#148279,#148280,#148281),
 .UNSPECIFIED.,.F.,.F.,(4,4),(2.06733813103431,2.11814920362238),
 .UNSPECIFIED.);
#23947=B_SPLINE_CURVE_WITH_KNOTS('',3,(#148283,#148284,#148285,#148286),
 .UNSPECIFIED.,.F.,.F.,(4,4),(3.73816266144136,3.7889737339741),
 .UNSPECIFIED.);
#23948=B_SPLINE_CURVE_WITH_KNOTS('',3,(#148288,#148289,#148290,#148291,
#148292,#148293,#148294,#148295,#148296,#148297,#148298,#148299,#148300,
#148301,#148302,#148303,#148304),.UNSPECIFIED.,.F.,.F.,(4,2,2,2,3,2,2,4),
(0.0529024352960807,0.0551226000944865,0.0590534470355066,0.0612484958735405,
0.0634408290669255,0.0672969289521807,0.0711810086621846,0.0739890800026948),
 .UNSPECIFIED.);
#23949=B_SPLINE_CURVE_WITH_KNOTS('',3,(#148305,#148306,#148307,#148308),
 .UNSPECIFIED.,.F.,.F.,(4,4),(2.06733813083286,2.11814920335294),
 .UNSPECIFIED.);
#23950=B_SPLINE_CURVE_WITH_KNOTS('',3,(#148310,#148311,#148312,#148313),
 .UNSPECIFIED.,.F.,.F.,(4,4),(3.73816266015891,3.78897373268002),
 .UNSPECIFIED.);
#23951=B_SPLINE_CURVE_WITH_KNOTS('',3,(#148315,#148316,#148317,#148318,
#148319,#148320,#148321,#148322,#148323,#148324,#148325,#148326,#148327,
#148328,#148329,#148330,#148331),.UNSPECIFIED.,.F.,.F.,(4,2,2,2,3,2,2,4),
(0.0529024352569361,0.0551226000955349,0.0590534470359355,0.0612484958737216,
0.0634408290669069,0.0672969289522366,0.0711810086627126,0.0739890799167341),
 .UNSPECIFIED.);
#23952=B_SPLINE_CURVE_WITH_KNOTS('',3,(#148332,#148333,#148334,#148335),
 .UNSPECIFIED.,.F.,.F.,(4,4),(2.06733813113835,2.11814920367071),
 .UNSPECIFIED.);
#23953=B_SPLINE_CURVE_WITH_KNOTS('',3,(#148337,#148338,#148339,#148340),
 .UNSPECIFIED.,.F.,.F.,(4,4),(3.7381626611044,3.78897373365368),
 .UNSPECIFIED.);
#23954=B_SPLINE_CURVE_WITH_KNOTS('',3,(#148342,#148343,#148344,#148345,
#148346,#148347,#148348,#148349,#148350,#148351,#148352,#148353,#148354,
#148355,#148356,#148357,#148358),.UNSPECIFIED.,.F.,.F.,(4,2,2,2,3,2,2,4),
(0.0529024352810775,0.0551226000949388,0.059053447035779,0.061248495873723,
0.0634408290670364,0.0672969289522796,0.071181008662396,0.0739890799780723),
 .UNSPECIFIED.);
#23955=B_SPLINE_CURVE_WITH_KNOTS('',3,(#148359,#148360,#148361,#148362),
 .UNSPECIFIED.,.F.,.F.,(4,4),(2.06733813095668,2.11814920343747),
 .UNSPECIFIED.);
#23956=B_SPLINE_CURVE_WITH_KNOTS('',3,(#148364,#148365,#148366,#148367),
 .UNSPECIFIED.,.F.,.F.,(4,4),(3.73816266102959,3.78897373355911),
 .UNSPECIFIED.);
#23957=B_SPLINE_CURVE_WITH_KNOTS('',3,(#148369,#148370,#148371,#148372,
#148373,#148374,#148375,#148376,#148377,#148378,#148379,#148380,#148381,
#148382,#148383,#148384,#148385),.UNSPECIFIED.,.F.,.F.,(4,2,2,2,3,2,2,4),
(0.0529024352095704,0.0551226000943593,0.0590534470350723,0.0612484958730129,
0.0634408290663316,0.0672969289516666,0.0711810086618903,0.0739890799467104),
 .UNSPECIFIED.);
#23958=B_SPLINE_CURVE_WITH_KNOTS('',3,(#148386,#148387,#148388,#148389),
 .UNSPECIFIED.,.F.,.F.,(4,4),(2.06733813091365,2.11814920351671),
 .UNSPECIFIED.);
#23959=B_SPLINE_CURVE_WITH_KNOTS('',3,(#148391,#148392,#148393,#148394),
 .UNSPECIFIED.,.F.,.F.,(4,4),(3.73816266050385,3.78897373306035),
 .UNSPECIFIED.);
#23960=B_SPLINE_CURVE_WITH_KNOTS('',3,(#148396,#148397,#148398,#148399,
#148400,#148401,#148402,#148403,#148404,#148405,#148406,#148407,#148408,
#148409,#148410,#148411,#148412),.UNSPECIFIED.,.F.,.F.,(4,2,2,2,3,2,2,4),
(0.0529024352813181,0.055122600095314,0.0590534470358095,0.061248495873635,
0.0634408290668542,0.0672969289521644,0.0711810086625508,0.073989079997811),
 .UNSPECIFIED.);
#23961=B_SPLINE_CURVE_WITH_KNOTS('',3,(#148413,#148414,#148415,#148416),
 .UNSPECIFIED.,.F.,.F.,(4,4),(2.06733813112279,2.11814920361366),
 .UNSPECIFIED.);
#23962=B_SPLINE_CURVE_WITH_KNOTS('',3,(#148418,#148419,#148420,#148421),
 .UNSPECIFIED.,.F.,.F.,(4,4),(3.73816266180585,3.78897373432959),
 .UNSPECIFIED.);
#23963=B_SPLINE_CURVE_WITH_KNOTS('',3,(#148423,#148424,#148425,#148426,
#148427,#148428,#148429,#148430,#148431,#148432,#148433,#148434,#148435,
#148436,#148437,#148438,#148439),.UNSPECIFIED.,.F.,.F.,(4,2,2,2,3,2,2,4),
(0.0529024353383817,0.0551226000952313,0.0590534470363804,0.0612484958744086,
0.0634408290677798,0.0672969289529119,0.0711810086627874,0.0739890799666121),
 .UNSPECIFIED.);
#23964=B_SPLINE_CURVE_WITH_KNOTS('',3,(#148440,#148441,#148442,#148443),
 .UNSPECIFIED.,.F.,.F.,(4,4),(2.06733813079015,2.11814920328276),
 .UNSPECIFIED.);
#23965=B_SPLINE_CURVE_WITH_KNOTS('',3,(#148445,#148446,#148447,#148448),
 .UNSPECIFIED.,.F.,.F.,(4,4),(3.73816266000277,3.78897373256649),
 .UNSPECIFIED.);
#23966=B_SPLINE_CURVE_WITH_KNOTS('',3,(#148450,#148451,#148452,#148453,
#148454,#148455,#148456,#148457,#148458,#148459,#148460,#148461,#148462,
#148463,#148464,#148465,#148466),.UNSPECIFIED.,.F.,.F.,(4,2,2,2,3,2,2,4),
(0.0529024352886305,0.0551226000964549,0.0590534470368377,0.0612484958745884,
0.06344082906773,0.0672969289529962,0.0711810086634918,0.0739890798865082),
 .UNSPECIFIED.);
#23967=B_SPLINE_CURVE_WITH_KNOTS('',3,(#148467,#148468,#148469,#148470),
 .UNSPECIFIED.,.F.,.F.,(4,4),(2.0673381311841,2.11814920373392),
 .UNSPECIFIED.);
#23968=B_SPLINE_CURVE_WITH_KNOTS('',3,(#148472,#148473,#148474,#148475),
 .UNSPECIFIED.,.F.,.F.,(4,4),(3.7381626598156,3.78897373232901),
 .UNSPECIFIED.);
#23969=B_SPLINE_CURVE_WITH_KNOTS('',3,(#148477,#148478,#148479,#148480,
#148481,#148482,#148483,#148484,#148485,#148486,#148487,#148488,#148489,
#148490,#148491,#148492,#148493),.UNSPECIFIED.,.F.,.F.,(4,2,2,2,3,2,2,4),
(0.0529024351998522,0.0551226000957807,0.0590534470360129,0.0612484958737305,
0.063440829066862,0.0672969289521915,0.0711810086627707,0.0739890799251832),
 .UNSPECIFIED.);
#23970=B_SPLINE_CURVE_WITH_KNOTS('',3,(#148494,#148495,#148496,#148497),
 .UNSPECIFIED.,.F.,.F.,(4,4),(2.06733813124236,2.11814920376004),
 .UNSPECIFIED.);
#23971=B_SPLINE_CURVE_WITH_KNOTS('',3,(#148499,#148500,#148501,#148502),
 .UNSPECIFIED.,.F.,.F.,(4,4),(3.73816266168604,3.78897373417607),
 .UNSPECIFIED.);
#23972=B_SPLINE_CURVE_WITH_KNOTS('',3,(#148504,#148505,#148506,#148507,
#148508,#148509,#148510,#148511,#148512,#148513,#148514,#148515,#148516,
#148517,#148518,#148519,#148520),.UNSPECIFIED.,.F.,.F.,(4,2,2,2,3,2,2,4),
(0.0529024352984763,0.0551226000947986,0.0590534470358693,0.0612484958738993,
0.0634408290672777,0.0672969289524761,0.0711810086624219,0.0739890800310639),
 .UNSPECIFIED.);
#23973=B_SPLINE_CURVE_WITH_KNOTS('',3,(#148521,#148522,#148523,#148524),
 .UNSPECIFIED.,.F.,.F.,(4,4),(2.06733813082859,2.11814920332163),
 .UNSPECIFIED.);
#23974=B_SPLINE_CURVE_WITH_KNOTS('',3,(#148526,#148527,#148528,#148529),
 .UNSPECIFIED.,.F.,.F.,(4,4),(3.73816266070724,3.78897373325739),
 .UNSPECIFIED.);
#23975=B_SPLINE_CURVE_WITH_KNOTS('',3,(#148531,#148532,#148533,#148534,
#148535,#148536,#148537,#148538,#148539,#148540,#148541,#148542,#148543,
#148544,#148545,#148546,#148547),.UNSPECIFIED.,.F.,.F.,(4,2,2,2,3,2,2,4),
(0.0529024352251564,0.0551226000947543,0.059053447035343,0.0612484958732276,
0.0634408290664983,0.0672969289518344,0.0711810086621559,0.0739890799592365),
 .UNSPECIFIED.);
#23976=B_SPLINE_CURVE_WITH_KNOTS('',3,(#148548,#148549,#148550,#148551),
 .UNSPECIFIED.,.F.,.F.,(4,4),(2.06733813102794,2.1181492036115),
 .UNSPECIFIED.);
#23977=B_SPLINE_CURVE_WITH_KNOTS('',3,(#148553,#148554,#148555,#148556),
 .UNSPECIFIED.,.F.,.F.,(4,4),(3.73816266082592,3.78897373338695),
 .UNSPECIFIED.);
#23978=B_SPLINE_CURVE_WITH_KNOTS('',3,(#148558,#148559,#148560,#148561,
#148562,#148563,#148564,#148565,#148566,#148567,#148568,#148569,#148570,
#148571,#148572,#148573,#148574),.UNSPECIFIED.,.F.,.F.,(4,2,2,2,3,2,2,4),
(0.052902435285732,0.0551226000951503,0.0590534470358304,0.0612484958737189,
0.0634408290669877,0.0672969289522547,0.0711810086624951,0.0739890799777724),
 .UNSPECIFIED.);
#23979=B_SPLINE_CURVE_WITH_KNOTS('',3,(#148575,#148576,#148577,#148578),
 .UNSPECIFIED.,.F.,.F.,(4,4),(2.06733813096253,2.11814920348551),
 .UNSPECIFIED.);
#23980=B_SPLINE_CURVE_WITH_KNOTS('',3,(#148580,#148581,#148582,#148583),
 .UNSPECIFIED.,.F.,.F.,(4,4),(3.73816266099154,3.78897373347697),
 .UNSPECIFIED.);
#23981=B_SPLINE_CURVE_WITH_KNOTS('',3,(#148585,#148586,#148587,#148588,
#148589,#148590,#148591,#148592,#148593,#148594,#148595,#148596,#148597,
#148598,#148599,#148600,#148601),.UNSPECIFIED.,.F.,.F.,(4,2,2,2,3,2,2,4),
(0.0529024352653158,0.0551226000958512,0.0590534470365838,0.0612484958744501,
0.0634408290676912,0.0672969289528806,0.0711810086630735,0.0739890798870407),
 .UNSPECIFIED.);
#23982=B_SPLINE_CURVE_WITH_KNOTS('',3,(#148602,#148603,#148604,#148605),
 .UNSPECIFIED.,.F.,.F.,(4,4),(2.06733813099677,2.11814920357114),
 .UNSPECIFIED.);
#23983=B_SPLINE_CURVE_WITH_KNOTS('',3,(#148607,#148608,#148609,#148610),
 .UNSPECIFIED.,.F.,.F.,(4,4),(3.73816266177325,3.78897373423991),
 .UNSPECIFIED.);
#23984=B_SPLINE_CURVE_WITH_KNOTS('',3,(#148612,#148613,#148614,#148615,
#148616,#148617,#148618,#148619,#148620,#148621,#148622,#148623,#148624,
#148625,#148626,#148627,#148628),.UNSPECIFIED.,.F.,.F.,(4,2,2,2,3,2,2,4),
(0.0529024353174922,0.0551226000947562,0.0590534470359121,0.0612484958739641,
0.0634408290673591,0.0672969289525375,0.0711810086624227,0.0739890799148762),
 .UNSPECIFIED.);
#23985=B_SPLINE_CURVE_WITH_KNOTS('',3,(#148629,#148630,#148631,#148632),
 .UNSPECIFIED.,.F.,.F.,(4,4),(2.06733813072299,2.11814920329931),
 .UNSPECIFIED.);
#23986=B_SPLINE_CURVE_WITH_KNOTS('',3,(#148634,#148635,#148636,#148637),
 .UNSPECIFIED.,.F.,.F.,(4,4),(3.73816266115613,3.78897373364958),
 .UNSPECIFIED.);
#23987=B_SPLINE_CURVE_WITH_KNOTS('',3,(#148639,#148640,#148641,#148642,
#148643,#148644,#148645,#148646,#148647,#148648,#148649,#148650,#148651,
#148652,#148653,#148654,#148655),.UNSPECIFIED.,.F.,.F.,(4,2,2,2,3,2,2,4),
(0.0529024352663877,0.0551226000951005,0.0590534470359006,0.061248495873833,
0.0634408290671345,0.0672969289523877,0.071181008662549,0.0739890799450588),
 .UNSPECIFIED.);
#23988=B_SPLINE_CURVE_WITH_KNOTS('',3,(#148656,#148657,#148658,#148659),
 .UNSPECIFIED.,.F.,.F.,(4,4),(2.06733813096761,2.11814920343851),
 .UNSPECIFIED.);
#23989=B_SPLINE_CURVE_WITH_KNOTS('',3,(#148661,#148662,#148663,#148664),
 .UNSPECIFIED.,.F.,.F.,(4,4),(3.73816266123958,3.78897373374303),
 .UNSPECIFIED.);
#23990=B_SPLINE_CURVE_WITH_KNOTS('',3,(#148666,#148667,#148668,#148669,
#148670,#148671,#148672,#148673,#148674,#148675,#148676,#148677,#148678,
#148679,#148680,#148681,#148682),.UNSPECIFIED.,.F.,.F.,(4,2,2,2,3,2,2,4),
(0.0529024352695806,0.0551226000945445,0.0590534470354143,0.0612484958733957,
0.0634408290667422,0.0672969289520255,0.0711810086621362,0.0739890799729577),
 .UNSPECIFIED.);
#23991=B_SPLINE_CURVE_WITH_KNOTS('',3,(#148683,#148684,#148685,#148686),
 .UNSPECIFIED.,.F.,.F.,(4,4),(2.06733813089893,2.11814920345364),
 .UNSPECIFIED.);
#23992=B_SPLINE_CURVE_WITH_KNOTS('',3,(#148688,#148689,#148690,#148691),
 .UNSPECIFIED.,.F.,.F.,(4,4),(3.73816266031907,3.78897373284873),
 .UNSPECIFIED.);
#23993=B_SPLINE_CURVE_WITH_KNOTS('',3,(#148693,#148694,#148695,#148696,
#148697,#148698,#148699,#148700,#148701,#148702,#148703,#148704,#148705,
#148706,#148707,#148708,#148709),.UNSPECIFIED.,.F.,.F.,(4,2,2,2,3,2,2,4),
(0.052902435265286,0.0551226000956631,0.0590534470361102,0.0612484958739062,
0.0634408290670971,0.0672969289523889,0.0711810086628101,0.0739890799683972),
 .UNSPECIFIED.);
#23994=B_SPLINE_CURVE_WITH_KNOTS('',3,(#148710,#148711,#148712,#148713),
 .UNSPECIFIED.,.F.,.F.,(4,4),(2.06733813117357,2.11814920366994),
 .UNSPECIFIED.);
#23995=B_SPLINE_CURVE_WITH_KNOTS('',3,(#148715,#148716,#148717,#148718),
 .UNSPECIFIED.,.F.,.F.,(4,4),(3.73816266063489,3.78897373319568),
 .UNSPECIFIED.);
#23996=B_SPLINE_CURVE_WITH_KNOTS('',3,(#148720,#148721,#148722,#148723,
#148724,#148725,#148726,#148727,#148728,#148729,#148730,#148731,#148732,
#148733,#148734,#148735,#148736),.UNSPECIFIED.,.F.,.F.,(4,2,2,2,3,2,2,4),
(0.0529024353177154,0.0551226000957153,0.0590534470363672,0.0612484958742148,
0.0634408290674435,0.067296928952665,0.07118100866292,0.0739890799725188),
 .UNSPECIFIED.);
#23997=B_SPLINE_CURVE_WITH_KNOTS('',3,(#148737,#148738,#148739,#148740),
 .UNSPECIFIED.,.F.,.F.,(4,4),(2.06733813102884,2.1181492034784),
 .UNSPECIFIED.);
#23998=B_SPLINE_CURVE_WITH_KNOTS('',3,(#148742,#148743,#148744,#148745),
 .UNSPECIFIED.,.F.,.F.,(4,4),(3.73816266078816,3.78897373330558),
 .UNSPECIFIED.);
#23999=B_SPLINE_CURVE_WITH_KNOTS('',3,(#148747,#148748,#148749,#148750,
#148751,#148752,#148753,#148754,#148755,#148756,#148757,#148758,#148759,
#148760,#148761,#148762,#148763),.UNSPECIFIED.,.F.,.F.,(4,2,2,2,3,2,2,4),
(0.0529024353240009,0.0551226000961563,0.0590534470368356,0.0612484958746766,
0.0634408290678929,0.0672969289530824,0.0711810086633302,0.0739890799110409),
 .UNSPECIFIED.);
#24000=B_SPLINE_CURVE_WITH_KNOTS('',3,(#148764,#148765,#148766,#148767),
 .UNSPECIFIED.,.F.,.F.,(4,4),(2.0673381310135,2.11814920352267),
 .UNSPECIFIED.);
#24001=B_SPLINE_CURVE_WITH_KNOTS('',3,(#148769,#148770,#148771,#148772),
 .UNSPECIFIED.,.F.,.F.,(4,4),(3.73816266085092,3.78897373334858),
 .UNSPECIFIED.);
#24002=B_SPLINE_CURVE_WITH_KNOTS('',3,(#148774,#148775,#148776,#148777,
#148778,#148779,#148780,#148781,#148782,#148783),.UNSPECIFIED.,.F.,.F.,
(4,2,2,2,4),(0.0529024352988807,0.0551226000957205,0.0590534470364613,0.0612484958743386,
0.0634408290675894),.UNSPECIFIED.);
#24003=B_SPLINE_CURVE_WITH_KNOTS('',3,(#148788,#148789,#148790,#148791,
#148792,#148793,#148794,#148795),.UNSPECIFIED.,.F.,.F.,(4,2,2,4),(0.0634408290675894,
0.0672969289527968,0.0711810086629958,0.073989079915298),.UNSPECIFIED.);
#24004=B_SPLINE_CURVE_WITH_KNOTS('',3,(#148796,#148797,#148798,#148799),
 .UNSPECIFIED.,.F.,.F.,(4,4),(2.06733813101515,2.11814920351282),
 .UNSPECIFIED.);
#24005=B_SPLINE_CURVE_WITH_KNOTS('',3,(#148801,#148802,#148803,#148804),
 .UNSPECIFIED.,.F.,.F.,(4,4),(3.73816266103402,3.78897373354396),
 .UNSPECIFIED.);
#24006=B_SPLINE_CURVE_WITH_KNOTS('',3,(#148806,#148807,#148808,#148809,
#148810,#148811,#148812,#148813,#148814,#148815,#148816,#148817,#148818,
#148819,#148820,#148821,#148822),.UNSPECIFIED.,.F.,.F.,(4,2,2,2,3,2,2,4),
(0.0529024353036826,0.0551226000958266,0.0590534470366519,0.0612484958745524,
0.0634408290678181,0.0672969289529889,0.0711810086631166,0.07398907989072),
 .UNSPECIFIED.);
#24007=B_SPLINE_CURVE_WITH_KNOTS('',3,(#148823,#148824,#148825,#148826),
 .UNSPECIFIED.,.F.,.F.,(4,4),(2.06733813100458,2.11814920352257),
 .UNSPECIFIED.);
#24008=B_SPLINE_CURVE_WITH_KNOTS('',3,(#148828,#148829,#148830,#148831),
 .UNSPECIFIED.,.F.,.F.,(4,4),(3.73816266106249,3.78897373354877),
 .UNSPECIFIED.);
#24009=B_SPLINE_CURVE_WITH_KNOTS('',3,(#148833,#148834,#148835,#148836,
#148837,#148838,#148839,#148840,#148841,#148842,#148843,#148844,#148845,
#148846,#148847,#148848,#148849),.UNSPECIFIED.,.F.,.F.,(4,2,2,2,3,2,2,4),
(0.0529024352792874,0.0551226000954993,0.0590534470363064,0.0612484958742183,
0.0634408290674978,0.0672969289527032,0.0711810086628473,0.0739890798962569),
 .UNSPECIFIED.);
#24010=B_SPLINE_CURVE_WITH_KNOTS('',3,(#148850,#148851,#148852,#148853),
 .UNSPECIFIED.,.F.,.F.,(4,4),(2.06733813090294,2.11814920352042),
 .UNSPECIFIED.);
#24011=B_SPLINE_CURVE_WITH_KNOTS('',3,(#148855,#148856,#148857,#148858),
 .UNSPECIFIED.,.F.,.F.,(4,4),(3.73816266145574,3.78897373392224),
 .UNSPECIFIED.);
#24012=B_SPLINE_CURVE_WITH_KNOTS('',3,(#148860,#148861,#148862,#148863,
#148864,#148865,#148866,#148867,#148868,#148869,#148870,#148871,#148872,
#148873,#148874,#148875,#148876),.UNSPECIFIED.,.F.,.F.,(4,2,2,2,3,2,2,4),
(0.0529024352447713,0.0551226000947896,0.059053447035766,0.0612484958737659,
0.0634408290671224,0.0672969289523521,0.0711810086623765,0.073989079947909),
 .UNSPECIFIED.);
#24013=B_SPLINE_CURVE_WITH_KNOTS('',3,(#148877,#148878,#148879,#148880),
 .UNSPECIFIED.,.F.,.F.,(4,4),(2.06733813079829,2.11814920332747),
 .UNSPECIFIED.);
#24014=B_SPLINE_CURVE_WITH_KNOTS('',3,(#148882,#148883,#148884,#148885),
 .UNSPECIFIED.,.F.,.F.,(4,4),(3.73816266052439,3.7889737331077),
 .UNSPECIFIED.);
#24015=B_SPLINE_CURVE_WITH_KNOTS('',3,(#148887,#148888,#148889,#148890,
#148891,#148892,#148893,#148894,#148895,#148896,#148897,#148898,#148899,
#148900,#148901,#148902,#148903),.UNSPECIFIED.,.F.,.F.,(4,2,2,2,3,2,2,4),
(0.0529024352696748,0.0551226000951075,0.0590534470356228,0.061248495873468,
0.0634408290667037,0.0672969289520287,0.0711810086624032,0.0739890799428344),
 .UNSPECIFIED.);
#24016=B_SPLINE_CURVE_WITH_KNOTS('',3,(#148904,#148905,#148906,#148907),
 .UNSPECIFIED.,.F.,.F.,(4,4),(2.06733813108993,2.11814920359329),
 .UNSPECIFIED.);
#24017=B_SPLINE_CURVE_WITH_KNOTS('',3,(#148909,#148910,#148911,#148912),
 .UNSPECIFIED.,.F.,.F.,(4,4),(3.73816266065588,3.7889737331094),
 .UNSPECIFIED.);
#24018=B_SPLINE_CURVE_WITH_KNOTS('',3,(#148914,#148915,#148916,#148917,
#148918,#148919,#148920,#148921,#148922,#148923,#148924,#148925,#148926,
#148927,#148928,#148929,#148930),.UNSPECIFIED.,.F.,.F.,(4,2,2,2,3,2,2,4),
(0.0529024352500216,0.0551226000953363,0.0590534470359648,0.0612484958738279,
0.0634408290670738,0.0672969289523469,0.0711810086626337,0.0739890799467816),
 .UNSPECIFIED.);
#24019=B_SPLINE_CURVE_WITH_KNOTS('',3,(#148931,#148932,#148933,#148934),
 .UNSPECIFIED.,.F.,.F.,(4,4),(2.06733813108585,2.1181492035795),
 .UNSPECIFIED.);
#24020=B_SPLINE_CURVE_WITH_KNOTS('',3,(#148936,#148937,#148938,#148939),
 .UNSPECIFIED.,.F.,.F.,(4,4),(3.73816265997327,3.78897373253894),
 .UNSPECIFIED.);
#24021=B_SPLINE_CURVE_WITH_KNOTS('',3,(#148941,#148942,#148943,#148944,
#148945,#148946,#148947,#148948,#148949,#148950,#148951,#148952,#148953,
#148954,#148955,#148956,#148957),.UNSPECIFIED.,.F.,.F.,(4,2,2,2,3,2,2,4),
(0.0529024352877148,0.0551226000962212,0.0590534470365158,0.0612484958742325,
0.063440829067356,0.0672969289526359,0.0711810086631708,0.0739890799431124),
 .UNSPECIFIED.);
#24022=B_SPLINE_CURVE_WITH_KNOTS('',3,(#148958,#148959,#148960,#148961),
 .UNSPECIFIED.,.F.,.F.,(4,4),(2.06733813118465,2.11814920367701),
 .UNSPECIFIED.);
#24023=B_SPLINE_CURVE_WITH_KNOTS('',3,(#148963,#148964,#148965,#148966),
 .UNSPECIFIED.,.F.,.F.,(4,4),(3.73816266083586,3.78897373340648),
 .UNSPECIFIED.);
#24024=B_SPLINE_CURVE_WITH_KNOTS('',3,(#148968,#148969,#148970,#148971,
#148972,#148973,#148974,#148975,#148976,#148977,#148978,#148979,#148980,
#148981,#148982,#148983,#148984),.UNSPECIFIED.,.F.,.F.,(4,2,2,2,3,2,2,4),
(0.0529024353273861,0.0551226000958364,0.0590534470365822,0.0612484958744578,
0.0634408290677049,0.0672969289528934,0.0711810086630778,0.0739890799285735),
 .UNSPECIFIED.);
#24025=B_SPLINE_CURVE_WITH_KNOTS('',3,(#148985,#148986,#148987,#148988),
 .UNSPECIFIED.,.F.,.F.,(4,4),(2.06733813097796,2.11814920353602),
 .UNSPECIFIED.);
#24026=B_SPLINE_CURVE_WITH_KNOTS('',3,(#148990,#148991,#148992,#148993),
 .UNSPECIFIED.,.F.,.F.,(4,4),(3.73816266096225,3.78897373348547),
 .UNSPECIFIED.);
#24027=B_SPLINE_CURVE_WITH_KNOTS('',3,(#148995,#148996,#148997,#148998,
#148999,#149000,#149001,#149002,#149003,#149004,#149005,#149006,#149007,
#149008,#149009,#149010,#149011),.UNSPECIFIED.,.F.,.F.,(4,2,2,2,3,2,2,4),
(0.052902435235209,0.0551226000951272,0.0590534470358533,0.0612484958737601,
0.0634408290670416,0.0672969289523034,0.0711810086625133,0.0739890799273062),
 .UNSPECIFIED.);
#24028=B_SPLINE_CURVE_WITH_KNOTS('',3,(#149012,#149013,#149014,#149015),
 .UNSPECIFIED.,.F.,.F.,(4,4),(2.06733813095919,2.11814920352003),
 .UNSPECIFIED.);
#24029=B_SPLINE_CURVE_WITH_KNOTS('',3,(#149017,#149018,#149019,#149020),
 .UNSPECIFIED.,.F.,.F.,(4,4),(3.73816266110557,3.78897373362395),
 .UNSPECIFIED.);
#24030=B_SPLINE_CURVE_WITH_KNOTS('',3,(#149022,#149023,#149024,#149025,
#149026,#149027,#149028,#149029,#149030,#149031,#149032,#149033,#149034,
#149035,#149036,#149037,#149038),.UNSPECIFIED.,.F.,.F.,(4,2,2,2,3,2,2,4),
(0.0529024352527248,0.0551226000944423,0.0590534470352124,0.0612484958731709,
0.0634408290665012,0.0672969289518157,0.0711810086619979,0.0739890799933279),
 .UNSPECIFIED.);
#24031=B_SPLINE_CURVE_WITH_KNOTS('',3,(#149039,#149040,#149041,#149042),
 .UNSPECIFIED.,.F.,.F.,(4,4),(2.06733813088428,2.11814920342807),
 .UNSPECIFIED.);
#24032=B_SPLINE_CURVE_WITH_KNOTS('',3,(#149044,#149045,#149046,#149047),
 .UNSPECIFIED.,.F.,.F.,(4,4),(3.73816266018992,3.78897373275654),
 .UNSPECIFIED.);
#24033=B_SPLINE_CURVE_WITH_KNOTS('',3,(#149049,#149050,#149051,#149052,
#149053,#149054,#149055,#149056,#149057,#149058,#149059,#149060,#149061,
#149062,#149063,#149064,#149065),.UNSPECIFIED.,.F.,.F.,(4,2,2,2,3,2,2,4),
(0.0529024352595687,0.0551226000960166,0.0590534470363857,0.0612484958741364,
0.0634408290672885,0.0672969289525699,0.0711810086630519,0.0739890799145621),
 .UNSPECIFIED.);
#24034=B_SPLINE_CURVE_WITH_KNOTS('',3,(#149066,#149067,#149068,#149069),
 .UNSPECIFIED.,.F.,.F.,(4,4),(2.06733813112861,2.11814920361968),
 .UNSPECIFIED.);
#24035=B_SPLINE_CURVE_WITH_KNOTS('',3,(#149071,#149072,#149073,#149074),
 .UNSPECIFIED.,.F.,.F.,(4,4),(3.73816266179589,3.78897373426471),
 .UNSPECIFIED.);
#24036=B_SPLINE_CURVE_WITH_KNOTS('',3,(#149076,#149077,#149078,#149079,
#149080,#149081,#149082,#149083,#149084,#149085,#149086,#149087,#149088,
#149089,#149090,#149091,#149092),.UNSPECIFIED.,.F.,.F.,(4,2,2,2,3,2,2,4),
(0.0529024352876567,0.0551226000943113,0.0590534470354802,0.0612484958735684,
0.0634408290669972,0.0672969289522185,0.0711810086620985,0.0739890800129455),
 .UNSPECIFIED.);
#24037=B_SPLINE_CURVE_WITH_KNOTS('',3,(#149093,#149094,#149095,#149096),
 .UNSPECIFIED.,.F.,.F.,(4,4),(2.06733813072275,2.11814920323567),
 .UNSPECIFIED.);
#24038=B_SPLINE_CURVE_WITH_KNOTS('',3,(#149098,#149099,#149100,#149101),
 .UNSPECIFIED.,.F.,.F.,(4,4),(3.73816266167531,3.78897373415517),
 .UNSPECIFIED.);
#24039=B_SPLINE_CURVE_WITH_KNOTS('',3,(#149103,#149104,#149105,#149106,
#149107,#149108,#149109,#149110,#149111,#149112,#149113,#149114,#149115,
#149116,#149117,#149118,#149119),.UNSPECIFIED.,.F.,.F.,(4,2,2,2,3,2,2,4),
(0.0529024353277232,0.0551226000949464,0.0590534470360541,0.0612484958740863,
0.0634408290674636,0.0672969289526391,0.0711810086625577,0.0739890799254936),
 .UNSPECIFIED.);
#24040=B_SPLINE_CURVE_WITH_KNOTS('',3,(#149120,#149121,#149122,#149123),
 .UNSPECIFIED.,.F.,.F.,(4,4),(2.06733813079588,2.11814920335918),
 .UNSPECIFIED.);
#24041=B_SPLINE_CURVE_WITH_KNOTS('',3,(#149125,#149126,#149127,#149128),
 .UNSPECIFIED.,.F.,.F.,(4,4),(3.73816265995722,3.78897373248134),
 .UNSPECIFIED.);
#24042=B_SPLINE_CURVE_WITH_KNOTS('',3,(#149130,#149131,#149132,#149133,
#149134,#149135,#149136,#149137,#149138,#149139,#149140,#149141,#149142,
#149143,#149144,#149145,#149146),.UNSPECIFIED.,.F.,.F.,(4,2,2,2,3,2,2,4),
(0.0529024352479053,0.0551226000966192,0.0590534470369545,0.0612484958746632,
0.0634408290677745,0.0672969289530026,0.0711810086634966,0.0739890798762164),
 .UNSPECIFIED.);
#24043=B_SPLINE_CURVE_WITH_KNOTS('',3,(#149147,#149148,#149149,#149150),
 .UNSPECIFIED.,.F.,.F.,(4,4),(2.0673381312259,2.11814920375009),
 .UNSPECIFIED.);
#24044=B_SPLINE_CURVE_WITH_KNOTS('',3,(#149152,#149153,#149154,#149155),
 .UNSPECIFIED.,.F.,.F.,(4,4),(3.73816266135447,3.78897373388666),
 .UNSPECIFIED.);
#24045=B_SPLINE_CURVE_WITH_KNOTS('',3,(#149157,#149158,#149159,#149160,
#149161,#149162,#149163,#149164,#149165,#149166,#149167,#149168,#149169,
#149170,#149171,#149172,#149173),.UNSPECIFIED.,.F.,.F.,(4,2,2,2,3,2,2,4),
(0.0529024352810996,0.0551226000946487,0.0590534470355495,0.0612484958735367,
0.0634408290668853,0.0672969289521484,0.0711810086622316,0.0739890799314191),
 .UNSPECIFIED.);
#24046=B_SPLINE_CURVE_WITH_KNOTS('',3,(#149174,#149175,#149176,#149177),
 .UNSPECIFIED.,.F.,.F.,(4,4),(2.06733813088284,2.11814920343982),
 .UNSPECIFIED.);
#24047=B_SPLINE_CURVE_WITH_KNOTS('',3,(#149179,#149180,#149181,#149182),
 .UNSPECIFIED.,.F.,.F.,(4,4),(3.73816266067428,3.78897373321881),
 .UNSPECIFIED.);
#24048=B_SPLINE_CURVE_WITH_KNOTS('',3,(#149184,#149185,#149186,#149187,
#149188,#149189,#149190,#149191,#149192,#149193,#149194,#149195,#149196,
#149197,#149198,#149199,#149200),.UNSPECIFIED.,.F.,.F.,(4,2,2,2,3,2,2,4),
(0.0529024352649618,0.0551226000945426,0.0590534470351731,0.0612484958730819,
0.0634408290663741,0.0672969289517207,0.0711810086620141,0.07398908000207),
 .UNSPECIFIED.);
#24049=B_SPLINE_CURVE_WITH_KNOTS('',3,(#149201,#149202,#149203,#149204),
 .UNSPECIFIED.,.F.,.F.,(4,4),(2.06733813102838,2.118149203558),
 .UNSPECIFIED.);
#24050=B_SPLINE_CURVE_WITH_KNOTS('',3,(#149206,#149207,#149208,#149209),
 .UNSPECIFIED.,.F.,.F.,(4,4),(3.73816266066757,3.78897373314874),
 .UNSPECIFIED.);
#24051=B_SPLINE_CURVE_WITH_KNOTS('',3,(#149211,#149212,#149213,#149214,
#149215,#149216,#149217,#149218,#149219,#149220,#149221,#149222,#149223,
#149224,#149225,#149226,#149227),.UNSPECIFIED.,.F.,.F.,(4,2,2,2,3,2,2,4),
(0.0529024352349786,0.055122600095423,0.0590534470359997,0.0612484958738441,
0.0634408290670744,0.0672969289523512,0.071181008662676,0.0739890799320359),
 .UNSPECIFIED.);
#24052=B_SPLINE_CURVE_WITH_KNOTS('',3,(#149228,#149229,#149230,#149231),
 .UNSPECIFIED.,.F.,.F.,(4,4),(2.06733813103437,2.11814920362244),
 .UNSPECIFIED.);
#24053=B_SPLINE_CURVE_WITH_KNOTS('',3,(#149233,#149234,#149235,#149236),
 .UNSPECIFIED.,.F.,.F.,(4,4),(3.73816266144136,3.78897373397411),
 .UNSPECIFIED.);
#24054=B_SPLINE_CURVE_WITH_KNOTS('',3,(#149238,#149239,#149240,#149241,
#149242,#149243,#149244,#149245,#149246,#149247,#149248,#149249,#149250,
#149251,#149252,#149253,#149254),.UNSPECIFIED.,.F.,.F.,(4,2,2,2,3,2,2,4),
(0.052902435296,0.0551226000943973,0.0590534470353996,0.061248495873431,
0.0634408290668166,0.067296928952072,0.0711810086620752,0.0739890800025833),
 .UNSPECIFIED.);
#24055=B_SPLINE_CURVE_WITH_KNOTS('',3,(#149255,#149256,#149257,#149258),
 .UNSPECIFIED.,.F.,.F.,(4,4),(2.06733813083286,2.11814920335294),
 .UNSPECIFIED.);
#24056=B_SPLINE_CURVE_WITH_KNOTS('',3,(#149260,#149261,#149262,#149263),
 .UNSPECIFIED.,.F.,.F.,(4,4),(3.73816266015891,3.78897373268002),
 .UNSPECIFIED.);
#24057=B_SPLINE_CURVE_WITH_KNOTS('',3,(#149265,#149266,#149267,#149268,
#149269,#149270,#149271,#149272,#149273,#149274,#149275,#149276,#149277,
#149278,#149279,#149280,#149281),.UNSPECIFIED.,.F.,.F.,(4,2,2,2,3,2,2,4),
(0.0529024352568632,0.0551226000954583,0.0590534470358464,0.0612484958736338,
0.0634408290668215,0.0672969289521498,0.0711810086626215,0.0739890799166402),
 .UNSPECIFIED.);
#24058=B_SPLINE_CURVE_WITH_KNOTS('',3,(#149282,#149283,#149284,#149285),
 .UNSPECIFIED.,.F.,.F.,(4,4),(2.06733813113834,2.11814920367071),
 .UNSPECIFIED.);
#24059=B_SPLINE_CURVE_WITH_KNOTS('',3,(#149287,#149288,#149289,#149290),
 .UNSPECIFIED.,.F.,.F.,(4,4),(3.7381626611044,3.78897373365368),
 .UNSPECIFIED.);
#24060=B_SPLINE_CURVE_WITH_KNOTS('',3,(#149292,#149293,#149294,#149295,
#149296,#149297,#149298,#149299,#149300,#149301,#149302,#149303,#149304,
#149305,#149306,#149307,#149308),.UNSPECIFIED.,.F.,.F.,(4,2,2,2,3,2,2,4),
(0.0529024352810882,0.0551226000949496,0.0590534470357903,0.0612484958737411,
0.063440829067058,0.0672969289523027,0.0711810086624234,0.0739890799781007),
 .UNSPECIFIED.);
#24061=B_SPLINE_CURVE_WITH_KNOTS('',3,(#149309,#149310,#149311,#149312),
 .UNSPECIFIED.,.F.,.F.,(4,4),(2.06733813095668,2.11814920343747),
 .UNSPECIFIED.);
#24062=B_SPLINE_CURVE_WITH_KNOTS('',3,(#149314,#149315,#149316,#149317),
 .UNSPECIFIED.,.F.,.F.,(4,4),(3.73816266102959,3.78897373355911),
 .UNSPECIFIED.);
#24063=B_SPLINE_CURVE_WITH_KNOTS('',3,(#149319,#149320,#149321,#149322,
#149323,#149324,#149325,#149326,#149327,#149328,#149329,#149330,#149331,
#149332,#149333,#149334,#149335),.UNSPECIFIED.,.F.,.F.,(4,2,2,2,3,2,2,4),
(0.0529024352096333,0.0551226000944241,0.0590534470351423,0.0612484958730844,
0.0634408290664034,0.0672969289517397,0.071181008661968,0.0739890799467927),
 .UNSPECIFIED.);
#24064=B_SPLINE_CURVE_WITH_KNOTS('',3,(#149336,#149337,#149338,#149339),
 .UNSPECIFIED.,.F.,.F.,(4,4),(2.06733813091365,2.11814920351671),
 .UNSPECIFIED.);
#24065=B_SPLINE_CURVE_WITH_KNOTS('',3,(#149341,#149342,#149343,#149344),
 .UNSPECIFIED.,.F.,.F.,(4,4),(3.73816266050385,3.78897373306035),
 .UNSPECIFIED.);
#24066=B_SPLINE_CURVE_WITH_KNOTS('',3,(#149346,#149347,#149348,#149349,
#149350,#149351,#149352,#149353,#149354,#149355,#149356,#149357,#149358,
#149359,#149360,#149361,#149362),.UNSPECIFIED.,.F.,.F.,(4,2,2,2,3,2,2,4),
(0.0529024352812999,0.0551226000952955,0.0590534470357909,0.0612484958736166,
0.0634408290668356,0.0672969289521453,0.0711810086625308,0.0739890799977917),
 .UNSPECIFIED.);
#24067=B_SPLINE_CURVE_WITH_KNOTS('',3,(#149363,#149364,#149365,#149366),
 .UNSPECIFIED.,.F.,.F.,(4,4),(2.06733813112279,2.11814920361366),
 .UNSPECIFIED.);
#24068=B_SPLINE_CURVE_WITH_KNOTS('',3,(#149368,#149369,#149370,#149371),
 .UNSPECIFIED.,.F.,.F.,(4,4),(3.73816266180585,3.78897373432959),
 .UNSPECIFIED.);
#24069=B_SPLINE_CURVE_WITH_KNOTS('',3,(#149373,#149374,#149375,#149376,
#149377,#149378,#149379,#149380,#149381,#149382,#149383,#149384,#149385,
#149386,#149387,#149388,#149389),.UNSPECIFIED.,.F.,.F.,(4,2,2,2,3,2,2,4),
(0.0529024353383955,0.0551226000952457,0.0590534470363997,0.0612484958744295,
0.063440829067801,0.0672969289529328,0.0711810086628092,0.0739890799666374),
 .UNSPECIFIED.);
#24070=B_SPLINE_CURVE_WITH_KNOTS('',3,(#149390,#149391,#149392,#149393),
 .UNSPECIFIED.,.F.,.F.,(4,4),(2.06733813079015,2.11814920328276),
 .UNSPECIFIED.);
#24071=B_SPLINE_CURVE_WITH_KNOTS('',3,(#149395,#149396,#149397,#149398),
 .UNSPECIFIED.,.F.,.F.,(4,4),(3.73816266000277,3.78897373256649),
 .UNSPECIFIED.);
#24072=B_SPLINE_CURVE_WITH_KNOTS('',3,(#149400,#149401,#149402,#149403,
#149404,#149405,#149406,#149407,#149408,#149409,#149410,#149411,#149412,
#149413,#149414,#149415,#149416),.UNSPECIFIED.,.F.,.F.,(4,2,2,2,3,2,2,4),
(0.0529024352884472,0.0551226000962587,0.0590534470366154,0.0612484958743516,
0.0634408290674888,0.0672969289527537,0.0711810086632452,0.0739890798862568),
 .UNSPECIFIED.);
#24073=B_SPLINE_CURVE_WITH_KNOTS('',3,(#149417,#149418,#149419,#149420),
 .UNSPECIFIED.,.F.,.F.,(4,4),(2.06733813118411,2.11814920373392),
 .UNSPECIFIED.);
#24074=B_SPLINE_CURVE_WITH_KNOTS('',3,(#149422,#149423,#149424,#149425),
 .UNSPECIFIED.,.F.,.F.,(4,4),(3.73816265981561,3.78897373232902),
 .UNSPECIFIED.);
#24075=B_SPLINE_CURVE_WITH_KNOTS('',3,(#149427,#149428,#149429,#149430,
#149431,#149432,#149433,#149434,#149435,#149436,#149437,#149438,#149439,
#149440,#149441,#149442,#149443),.UNSPECIFIED.,.F.,.F.,(4,2,2,2,3,2,2,4),
(0.0529024351998951,0.0551226000958251,0.0590534470360602,0.0612484958737785,
0.0634408290669098,0.0672969289522405,0.0711810086628216,0.0739890799252331),
 .UNSPECIFIED.);
#24076=B_SPLINE_CURVE_WITH_KNOTS('',3,(#149444,#149445,#149446,#149447),
 .UNSPECIFIED.,.F.,.F.,(4,4),(2.06733813124236,2.11814920376004),
 .UNSPECIFIED.);
#24077=B_SPLINE_CURVE_WITH_KNOTS('',3,(#149449,#149450,#149451,#149452),
 .UNSPECIFIED.,.F.,.F.,(4,4),(3.73816266168605,3.78897373417608),
 .UNSPECIFIED.);
#24078=B_SPLINE_CURVE_WITH_KNOTS('',3,(#149454,#149455,#149456,#149457,
#149458,#149459,#149460,#149461,#149462,#149463,#149464,#149465,#149466,
#149467,#149468,#149469,#149470),.UNSPECIFIED.,.F.,.F.,(4,2,2,2,3,2,2,4),
(0.0529024352984499,0.05512260009477,0.0590534470358401,0.0612484958738678,
0.0634408290672449,0.0672969289524419,0.0711810086623853,0.0739890800310274),
 .UNSPECIFIED.);
#24079=B_SPLINE_CURVE_WITH_KNOTS('',3,(#149471,#149472,#149473,#149474),
 .UNSPECIFIED.,.F.,.F.,(4,4),(2.06733813082859,2.11814920332163),
 .UNSPECIFIED.);
#24080=B_SPLINE_CURVE_WITH_KNOTS('',3,(#149476,#149477,#149478,#149479),
 .UNSPECIFIED.,.F.,.F.,(4,4),(3.73816266070724,3.78897373325739),
 .UNSPECIFIED.);
#24081=B_SPLINE_CURVE_WITH_KNOTS('',3,(#149481,#149482,#149483,#149484,
#149485,#149486,#149487,#149488,#149489,#149490,#149491,#149492,#149493,
#149494,#149495,#149496,#149497),.UNSPECIFIED.,.F.,.F.,(4,2,2,2,3,2,2,4),
(0.0529024352251411,0.0551226000947361,0.0590534470353222,0.0612484958732058,
0.0634408290664763,0.0672969289518134,0.0711810086621348,0.0739890799592117),
 .UNSPECIFIED.);
#24082=B_SPLINE_CURVE_WITH_KNOTS('',3,(#149498,#149499,#149500,#149501),
 .UNSPECIFIED.,.F.,.F.,(4,4),(2.06733813102795,2.1181492036115),
 .UNSPECIFIED.);
#24083=B_SPLINE_CURVE_WITH_KNOTS('',3,(#149503,#149504,#149505,#149506),
 .UNSPECIFIED.,.F.,.F.,(4,4),(3.73816266082592,3.78897373338695),
 .UNSPECIFIED.);
#24084=B_SPLINE_CURVE_WITH_KNOTS('',3,(#149508,#149509,#149510,#149511,
#149512,#149513,#149514,#149515,#149516,#149517,#149518,#149519,#149520,
#149521,#149522,#149523,#149524),.UNSPECIFIED.,.F.,.F.,(4,2,2,2,3,2,2,4),
(0.0529024352857602,0.0551226000951809,0.0590534470358672,0.0612484958737567,
0.0634408290670247,0.0672969289522904,0.0711810086625272,0.0739890799778034),
 .UNSPECIFIED.);
#24085=B_SPLINE_CURVE_WITH_KNOTS('',3,(#149525,#149526,#149527,#149528),
 .UNSPECIFIED.,.F.,.F.,(4,4),(2.06733813096253,2.11814920348551),
 .UNSPECIFIED.);
#24086=B_SPLINE_CURVE_WITH_KNOTS('',3,(#149530,#149531,#149532,#149533),
 .UNSPECIFIED.,.F.,.F.,(4,4),(3.73816266099154,3.78897373347697),
 .UNSPECIFIED.);
#24087=B_SPLINE_CURVE_WITH_KNOTS('',3,(#149535,#149536,#149537,#149538,
#149539,#149540,#149541,#149542,#149543,#149544,#149545,#149546,#149547,
#149548,#149549,#149550,#149551),.UNSPECIFIED.,.F.,.F.,(4,2,2,2,3,2,2,4),
(0.0529024352652794,0.0551226000958151,0.0590534470365479,0.061248495874416,
0.0634408290676581,0.0672969289528476,0.0711810086630389,0.0739890798870025),
 .UNSPECIFIED.);
#24088=B_SPLINE_CURVE_WITH_KNOTS('',3,(#149552,#149553,#149554,#149555),
 .UNSPECIFIED.,.F.,.F.,(4,4),(2.06733813099677,2.11814920357114),
 .UNSPECIFIED.);
#24089=B_SPLINE_CURVE_WITH_KNOTS('',3,(#149557,#149558,#149559,#149560),
 .UNSPECIFIED.,.F.,.F.,(4,4),(3.73816266177326,3.78897373423991),
 .UNSPECIFIED.);
#24090=B_SPLINE_CURVE_WITH_KNOTS('',3,(#149562,#149563,#149564,#149565,
#149566,#149567,#149568,#149569,#149570,#149571,#149572,#149573,#149574,
#149575,#149576,#149577,#149578),.UNSPECIFIED.,.F.,.F.,(4,2,2,2,3,2,2,4),
(0.0529024353175172,0.0551226000947811,0.0590534470359366,0.0612484958739924,
0.06344082906739,0.0672969289525678,0.0711810086624502,0.0739890799149026),
 .UNSPECIFIED.);
#24091=B_SPLINE_CURVE_WITH_KNOTS('',3,(#149579,#149580,#149581,#149582),
 .UNSPECIFIED.,.F.,.F.,(4,4),(2.06733813072299,2.11814920329931),
 .UNSPECIFIED.);
#24092=B_SPLINE_CURVE_WITH_KNOTS('',3,(#149584,#149585,#149586,#149587),
 .UNSPECIFIED.,.F.,.F.,(4,4),(3.73816266115613,3.78897373364958),
 .UNSPECIFIED.);
#24093=B_SPLINE_CURVE_WITH_KNOTS('',3,(#149589,#149590,#149591,#149592,
#149593,#149594,#149595,#149596,#149597,#149598,#149599,#149600,#149601,
#149602,#149603,#149604,#149605),.UNSPECIFIED.,.F.,.F.,(4,2,2,2,3,2,2,4),
(0.0529024352663513,0.0551226000950634,0.0590534470358615,0.0612484958737945,
0.063440829067096,0.0672969289523489,0.0711810086625087,0.0739890799450185),
 .UNSPECIFIED.);
#24094=B_SPLINE_CURVE_WITH_KNOTS('',3,(#149606,#149607,#149608,#149609),
 .UNSPECIFIED.,.F.,.F.,(4,4),(2.0673381309676,2.11814920343851),
 .UNSPECIFIED.);
#24095=B_SPLINE_CURVE_WITH_KNOTS('',3,(#149611,#149612,#149613,#149614),
 .UNSPECIFIED.,.F.,.F.,(4,4),(3.73816266123958,3.78897373374303),
 .UNSPECIFIED.);
#24096=B_SPLINE_CURVE_WITH_KNOTS('',3,(#149616,#149617,#149618,#149619,
#149620,#149621,#149622,#149623,#149624,#149625,#149626,#149627,#149628,
#149629,#149630,#149631,#149632),.UNSPECIFIED.,.F.,.F.,(4,2,2,2,3,2,2,4),
(0.0529024352695509,0.0551226000945128,0.0590534470353782,0.0612484958733598,
0.0634408290667064,0.0672969289519894,0.0711810086620986,0.0739890799729215),
 .UNSPECIFIED.);
#24097=B_SPLINE_CURVE_WITH_KNOTS('',3,(#149633,#149634,#149635,#149636),
 .UNSPECIFIED.,.F.,.F.,(4,4),(2.06733813089893,2.11814920345363),
 .UNSPECIFIED.);
#24098=B_SPLINE_CURVE_WITH_KNOTS('',3,(#149638,#149639,#149640,#149641),
 .UNSPECIFIED.,.F.,.F.,(4,4),(3.73816266031907,3.78897373284873),
 .UNSPECIFIED.);
#24099=B_SPLINE_CURVE_WITH_KNOTS('',3,(#149643,#149644,#149645,#149646,
#149647,#149648,#149649,#149650,#149651,#149652,#149653,#149654,#149655,
#149656,#149657,#149658,#149659),.UNSPECIFIED.,.F.,.F.,(4,2,2,2,3,2,2,4),
(0.0529024352652488,0.0551226000956238,0.0590534470360699,0.0612484958738631,
0.0634408290670526,0.0672969289523439,0.0711810086627632,0.0739890799683483),
 .UNSPECIFIED.);
#24100=B_SPLINE_CURVE_WITH_KNOTS('',3,(#149660,#149661,#149662,#149663),
 .UNSPECIFIED.,.F.,.F.,(4,4),(2.06733813117357,2.11814920366994),
 .UNSPECIFIED.);
#24101=B_SPLINE_CURVE_WITH_KNOTS('',3,(#149665,#149666,#149667,#149668),
 .UNSPECIFIED.,.F.,.F.,(4,4),(3.73816266063489,3.78897373319568),
 .UNSPECIFIED.);
#24102=B_SPLINE_CURVE_WITH_KNOTS('',3,(#149670,#149671,#149672,#149673,
#149674,#149675,#149676,#149677,#149678,#149679,#149680,#149681,#149682,
#149683,#149684,#149685,#149686),.UNSPECIFIED.,.F.,.F.,(4,2,2,2,3,2,2,4),
(0.0529024353177713,0.0551226000957727,0.0590534470364281,0.0612484958742786,
0.0634408290675083,0.0672969289527308,0.0711810086629895,0.0739890799725923),
 .UNSPECIFIED.);
#24103=B_SPLINE_CURVE_WITH_KNOTS('',3,(#149687,#149688,#149689,#149690),
 .UNSPECIFIED.,.F.,.F.,(4,4),(2.06733813102884,2.1181492034784),
 .UNSPECIFIED.);
#24104=B_SPLINE_CURVE_WITH_KNOTS('',3,(#149692,#149693,#149694,#149695),
 .UNSPECIFIED.,.F.,.F.,(4,4),(3.73816266078816,3.78897373330558),
 .UNSPECIFIED.);
#24105=B_SPLINE_CURVE_WITH_KNOTS('',3,(#149697,#149698,#149699,#149700,
#149701,#149702,#149703,#149704,#149705,#149706,#149707,#149708,#149709,
#149710,#149711,#149712,#149713),.UNSPECIFIED.,.F.,.F.,(4,2,2,2,3,2,2,4),
(0.052902435323927,0.0551226000960778,0.0590534470367477,0.061248495874586,
0.063440829067802,0.0672969289529904,0.0711810086632352,0.0739890799109451),
 .UNSPECIFIED.);
#24106=B_SPLINE_CURVE_WITH_KNOTS('',3,(#149714,#149715,#149716,#149717),
 .UNSPECIFIED.,.F.,.F.,(4,4),(2.0673381310135,2.11814920352267),
 .UNSPECIFIED.);
#24107=B_SPLINE_CURVE_WITH_KNOTS('',3,(#149718,#149719,#149720,#149721),
 .UNSPECIFIED.,.F.,.F.,(4,4),(3.73816266085093,3.78897373334859),
 .UNSPECIFIED.);
#24108=B_SPLINE_CURVE_WITH_KNOTS('',3,(#149726,#149727,#149728,#149729,
#149730,#149731,#149732,#149733,#149734,#149735),.UNSPECIFIED.,.F.,.F.,
(4,2,2,2,4),(0.0714824588585375,0.0744292845751612,0.0776622687682114,0.0817097633455992,
0.0826589280268188),.UNSPECIFIED.);
#24109=B_SPLINE_CURVE_WITH_KNOTS('',3,(#149736,#149737,#149738,#149739,
#149740,#149741),.UNSPECIFIED.,.F.,.F.,(4,2,4),(1.49996604605074,1.51351365753382,
1.57686258981781),.UNSPECIFIED.);
#24110=B_SPLINE_CURVE_WITH_KNOTS('',3,(#149743,#149744,#149745,#149746,
#149747,#149748),.UNSPECIFIED.,.F.,.F.,(4,2,4),(1.33957856730954,1.40292749963475,
1.41647511111458),.UNSPECIFIED.);
#24111=B_SPLINE_CURVE_WITH_KNOTS('',3,(#149750,#149751,#149752,#149753,
#149754,#149755,#149756,#149757,#149758,#149759,#149760,#149761,#149762,
#149763,#149764,#149765,#149766,#149767,#149768),.UNSPECIFIED.,.F.,.F.,
(4,2,2,2,3,2,2,2,4),(0.060099258269106,0.0615656153041754,0.0659612937711943,
0.0687970446775909,0.0714824588631871,0.074429284579545,0.0776622687720683,
0.0817097633487688,0.0826589280202759),.UNSPECIFIED.);
#24112=B_SPLINE_CURVE_WITH_KNOTS('',3,(#149769,#149770,#149771,#149772,
#149773,#149774),.UNSPECIFIED.,.F.,.F.,(4,2,4),(1.499966046113,1.51351365756774,
1.57686258990272),.UNSPECIFIED.);
#24113=B_SPLINE_CURVE_WITH_KNOTS('',3,(#149776,#149777,#149778,#149779,
#149780,#149781),.UNSPECIFIED.,.F.,.F.,(4,2,4),(1.33957856732956,1.40292749963323,
1.41647511110724),.UNSPECIFIED.);
#24114=B_SPLINE_CURVE_WITH_KNOTS('',3,(#149783,#149784,#149785,#149786,
#149787,#149788,#149789,#149790,#149791,#149792,#149793,#149794,#149795,
#149796,#149797,#149798,#149799,#149800,#149801),.UNSPECIFIED.,.F.,.F.,
(4,2,2,2,3,2,2,2,4),(0.060099258231316,0.0615656153015067,0.0659612937681578,
0.0687970446741911,0.0714824588595198,0.0744292845761485,0.077662268768905,
0.081709763345669,0.0826589280244342),.UNSPECIFIED.);
#24115=B_SPLINE_CURVE_WITH_KNOTS('',3,(#149802,#149803,#149804,#149805,
#149806,#149807),.UNSPECIFIED.,.F.,.F.,(4,2,4),(1.49996604607687,1.51351365757256,
1.5768625898645),.UNSPECIFIED.);
#24116=B_SPLINE_CURVE_WITH_KNOTS('',3,(#149809,#149810,#149811,#149812,
#149813,#149814),.UNSPECIFIED.,.F.,.F.,(4,2,4),(1.33957856716701,1.40292749942639,
1.41647511094955),.UNSPECIFIED.);
#24117=B_SPLINE_CURVE_WITH_KNOTS('',3,(#149816,#149817,#149818,#149819,
#149820,#149821,#149822,#149823,#149824,#149825,#149826,#149827,#149828,
#149829,#149830,#149831,#149832,#149833,#149834),.UNSPECIFIED.,.F.,.F.,
(4,2,2,2,3,2,2,2,4),(0.0600992582102493,0.0615656152977947,0.0659612937657737,
0.0687970446720995,0.0714824588576289,0.0744292845745221,0.0776622687668052,
0.0817097633421903,0.0826589280636074),.UNSPECIFIED.);
#24118=B_SPLINE_CURVE_WITH_KNOTS('',3,(#149835,#149836,#149837,#149838,
#149839,#149840),.UNSPECIFIED.,.F.,.F.,(4,2,4),(1.49996604614834,1.51351365759482,
1.5768625899084),.UNSPECIFIED.);
#24119=B_SPLINE_CURVE_WITH_KNOTS('',3,(#149842,#149843,#149844,#149845,
#149846,#149847),.UNSPECIFIED.,.F.,.F.,(4,2,4),(1.33957856752927,1.40292749981418,
1.41647511131301),.UNSPECIFIED.);
#24120=B_SPLINE_CURVE_WITH_KNOTS('',3,(#149849,#149850,#149851,#149852,
#149853,#149854,#149855,#149856,#149857,#149858,#149859,#149860,#149861,
#149862,#149863,#149864,#149865,#149866,#149867),.UNSPECIFIED.,.F.,.F.,
(4,2,2,2,3,2,2,2,4),(0.0600992581695721,0.0615656152962615,0.0659612937594313,
0.0687970446634821,0.0714824588473559,0.0744292845648293,0.0776622687592538,
0.0817097633381737,0.0826589280790036),.UNSPECIFIED.);
#24121=B_SPLINE_CURVE_WITH_KNOTS('',3,(#149868,#149869,#149870,#149871,
#149872,#149873),.UNSPECIFIED.,.F.,.F.,(4,2,4),(1.49996604595889,1.51351365749176,
1.57686258972957),.UNSPECIFIED.);
#24122=B_SPLINE_CURVE_WITH_KNOTS('',3,(#149875,#149876,#149877,#149878,
#149879,#149880),.UNSPECIFIED.,.F.,.F.,(4,2,4),(1.33957856752258,1.40292749978992,
1.41647511126154),.UNSPECIFIED.);
#24123=B_SPLINE_CURVE_WITH_KNOTS('',3,(#149882,#149883,#149884,#149885,
#149886,#149887,#149888,#149889,#149890,#149891,#149892,#149893,#149894,
#149895,#149896,#149897,#149898,#149899,#149900),.UNSPECIFIED.,.F.,.F.,
(4,2,2,2,3,2,2,2,4),(0.0600992582011184,0.0615656152986744,0.0659612937631065,
0.0687970446679523,0.0714824588524144,0.0744292845695169,0.0776622687632943,
0.0817097633414514,0.082658928035348),.UNSPECIFIED.);
#24124=B_SPLINE_CURVE_WITH_KNOTS('',3,(#149901,#149902,#149903,#149904,
#149905,#149906),.UNSPECIFIED.,.F.,.F.,(4,2,4),(1.49996604601399,1.51351365750487,
1.57686258982041),.UNSPECIFIED.);
#24125=B_SPLINE_CURVE_WITH_KNOTS('',3,(#149908,#149909,#149910,#149911,
#149912,#149913),.UNSPECIFIED.,.F.,.F.,(4,2,4),(1.33957856772149,1.40292750006868,
1.41647511150785),.UNSPECIFIED.);
#24126=B_SPLINE_CURVE_WITH_KNOTS('',3,(#149915,#149916,#149917,#149918,
#149919,#149920,#149921,#149922,#149923,#149924,#149925,#149926,#149927,
#149928,#149929,#149930,#149931,#149932,#149933),.UNSPECIFIED.,.F.,.F.,
(4,2,2,2,3,2,2,2,4),(0.0600992582193096,0.0615656153013013,0.0659612937627021,
0.0687970446664693,0.0714824588501472,0.0744292845671558,0.0776622687621161,
0.0817097633428454,0.0826589280107226),.UNSPECIFIED.);
#24127=B_SPLINE_CURVE_WITH_KNOTS('',3,(#149934,#149935,#149936,#149937,
#149938,#149939),.UNSPECIFIED.,.F.,.F.,(4,2,4),(1.49996604587209,1.51351365743327,
1.57686258967902),.UNSPECIFIED.);
#24128=B_SPLINE_CURVE_WITH_KNOTS('',3,(#149941,#149942,#149943,#149944,
#149945,#149946),.UNSPECIFIED.,.F.,.F.,(4,2,4),(1.33957856735936,1.40292749966726,
1.41647511117744),.UNSPECIFIED.);
#24129=B_SPLINE_CURVE_WITH_KNOTS('',3,(#149948,#149949,#149950,#149951,
#149952,#149953,#149954,#149955,#149956,#149957,#149958,#149959,#149960,
#149961,#149962,#149963,#149964,#149965,#149966),.UNSPECIFIED.,.F.,.F.,
(4,2,2,2,3,2,2,2,4),(0.0600992582674632,0.0615656153040191,0.065961293770234,
0.0687970446762131,0.071482458861508,0.0744292845779795,0.0776622687708636,
0.081709763348141,0.0826589280360798),.UNSPECIFIED.);
#24130=B_SPLINE_CURVE_WITH_KNOTS('',3,(#149967,#149968,#149969,#149970,
#149971,#149972),.UNSPECIFIED.,.F.,.F.,(4,2,4),(1.49996604600416,1.51351365750855,
1.57686258981381),.UNSPECIFIED.);
#24131=B_SPLINE_CURVE_WITH_KNOTS('',3,(#149974,#149975,#149976,#149977,
#149978,#149979),.UNSPECIFIED.,.F.,.F.,(4,2,4),(1.33957856738494,1.40292749967249,
1.41647511116503),.UNSPECIFIED.);
#24132=B_SPLINE_CURVE_WITH_KNOTS('',3,(#149981,#149982,#149983,#149984,
#149985,#149986,#149987,#149988,#149989,#149990,#149991,#149992,#149993,
#149994,#149995,#149996,#149997,#149998,#149999),.UNSPECIFIED.,.F.,.F.,
(4,2,2,2,3,2,2,2,4),(0.0600992582017652,0.0615656152976751,0.0659612937631273,
0.0687970446684009,0.0714824588531702,0.0744292845702252,0.0776622687635618,
0.0817097633408794,0.0826589280495392),.UNSPECIFIED.);
#24133=B_SPLINE_CURVE_WITH_KNOTS('',3,(#150000,#150001,#150002,#150003,
#150004,#150005),.UNSPECIFIED.,.F.,.F.,(4,2,4),(1.49996604604657,1.51351365754362,
1.57686258983577),.UNSPECIFIED.);
#24134=B_SPLINE_CURVE_WITH_KNOTS('',3,(#150007,#150008,#150009,#150010,
#150011,#150012),.UNSPECIFIED.,.F.,.F.,(4,2,4),(1.33957856727904,1.40292749957447,
1.41647511106941),.UNSPECIFIED.);
#24135=B_SPLINE_CURVE_WITH_KNOTS('',3,(#150014,#150015,#150016,#150017,
#150018,#150019,#150020,#150021,#150022,#150023,#150024,#150025,#150026,
#150027,#150028,#150029,#150030,#150031,#150032),.UNSPECIFIED.,.F.,.F.,
(4,2,2,2,3,2,2,2,4),(0.0600992581799993,0.0615656152943915,0.0659612937600584,
0.068797044664993,0.0714824588495034,0.0744292845670047,0.0776622687604493,
0.0817097633372922,0.0826589280917478),.UNSPECIFIED.);
#24136=B_SPLINE_CURVE_WITH_KNOTS('',3,(#150033,#150034,#150035,#150036,
#150037,#150038),.UNSPECIFIED.,.F.,.F.,(4,2,4),(1.49996604606282,1.51351365753196,
1.57686258981422),.UNSPECIFIED.);
#24137=B_SPLINE_CURVE_WITH_KNOTS('',3,(#150040,#150041,#150042,#150043,
#150044,#150045),.UNSPECIFIED.,.F.,.F.,(4,2,4),(1.33957856759873,1.40292749993747,
1.41647511140743),.UNSPECIFIED.);
#24138=B_SPLINE_CURVE_WITH_KNOTS('',3,(#150047,#150048,#150049,#150050,
#150051,#150052,#150053,#150054,#150055,#150056,#150057,#150058,#150059,
#150060,#150061,#150062,#150063,#150064,#150065),.UNSPECIFIED.,.F.,.F.,
(4,2,2,2,3,2,2,2,4),(0.0600992581996879,0.0615656152994879,0.0659612937614183,
0.0687970446653839,0.0714824588492078,0.0744292845662641,0.0776622687609925,
0.0817097633411702,0.0826589280132682),.UNSPECIFIED.);
#24139=B_SPLINE_CURVE_WITH_KNOTS('',3,(#150066,#150067,#150068,#150069,
#150070,#150071),.UNSPECIFIED.,.F.,.F.,(4,2,4),(1.49996604591879,1.51351365743313,
1.57686258971772),.UNSPECIFIED.);
#24140=B_SPLINE_CURVE_WITH_KNOTS('',3,(#150073,#150074,#150075,#150076,
#150077,#150078),.UNSPECIFIED.,.F.,.F.,(4,2,4),(1.3395785670504,1.40292749929253,
1.41647511082944),.UNSPECIFIED.);
#24141=B_SPLINE_CURVE_WITH_KNOTS('',3,(#150080,#150081,#150082,#150083,
#150084,#150085,#150086,#150087,#150088,#150089,#150090,#150091,#150092,
#150093,#150094,#150095,#150096,#150097,#150098),.UNSPECIFIED.,.F.,.F.,
(4,2,2,2,3,2,2,2,4),(0.0600992582212704,0.0615656152959939,0.065961293765843,
0.0687970446728489,0.0714824588588726,0.0744292845757802,0.0776622687673179,
0.0817097633411337,0.0826589280883185),.UNSPECIFIED.);
#24142=B_SPLINE_CURVE_WITH_KNOTS('',3,(#150099,#150100,#150101,#150102,
#150103,#150104),.UNSPECIFIED.,.F.,.F.,(4,2,4),(1.49996604617379,1.51351365761947,
1.5768625899443),.UNSPECIFIED.);
#24143=B_SPLINE_CURVE_WITH_KNOTS('',3,(#150106,#150107,#150108,#150109,
#150110,#150111),.UNSPECIFIED.,.F.,.F.,(4,2,4),(1.33957856714172,1.40292749936937,
1.41647511087422),.UNSPECIFIED.);
#24144=B_SPLINE_CURVE_WITH_KNOTS('',3,(#150113,#150114,#150115,#150116,
#150117,#150118,#150119,#150120,#150121,#150122,#150123,#150124,#150125,
#150126,#150127,#150128,#150129,#150130,#150131),.UNSPECIFIED.,.F.,.F.,
(4,2,2,2,3,2,2,2,4),(0.0600992582306656,0.0615656152998404,0.065961293769387,
0.0687970446765956,0.0714824588627838,0.0744292845793006,0.0776622687708418,
0.0817097633452896,0.0826589280442809),.UNSPECIFIED.);
#24145=B_SPLINE_CURVE_WITH_KNOTS('',3,(#150132,#150133,#150134,#150135,
#150136,#150137),.UNSPECIFIED.,.F.,.F.,(4,2,4),(1.4999660461885,1.51351365763824,
1.57686258995467),.UNSPECIFIED.);
#24146=B_SPLINE_CURVE_WITH_KNOTS('',3,(#150139,#150140,#150141,#150142,
#150143,#150144),.UNSPECIFIED.,.F.,.F.,(4,2,4),(1.33957856767546,1.402927500014,
1.41647511143919),.UNSPECIFIED.);
#24147=B_SPLINE_CURVE_WITH_KNOTS('',3,(#150146,#150147,#150148,#150149,
#150150,#150151,#150152,#150153,#150154,#150155,#150156,#150157,#150158,
#150159,#150160,#150161,#150162,#150163,#150164),.UNSPECIFIED.,.F.,.F.,
(4,2,2,2,3,2,2,2,4),(0.0600992582048306,0.0615656153055392,0.0659612937676691,
0.0687970446720172,0.0714824588561295,0.0744292845727573,0.0776622687673379,
0.081709763347868,0.082658927996682),.UNSPECIFIED.);
#24148=B_SPLINE_CURVE_WITH_KNOTS('',3,(#150165,#150166,#150167,#150168,
#150169,#150170),.UNSPECIFIED.,.F.,.F.,(4,2,4),(1.49996604592438,1.51351365744584,
1.57686258971838),.UNSPECIFIED.);
#24149=B_SPLINE_CURVE_WITH_KNOTS('',3,(#150172,#150173,#150174,#150175,
#150176,#150177),.UNSPECIFIED.,.F.,.F.,(4,2,4),(1.33957856718658,1.40292749947563,
1.41647511098612),.UNSPECIFIED.);
#24150=B_SPLINE_CURVE_WITH_KNOTS('',3,(#150179,#150180,#150181,#150182,
#150183,#150184,#150185,#150186,#150187,#150188,#150189,#150190,#150191,
#150192,#150193,#150194,#150195,#150196,#150197),.UNSPECIFIED.,.F.,.F.,
(4,2,2,2,3,2,2,2,4),(0.0600992581919431,0.0615656152953891,0.0659612937624275,
0.0687970446682301,0.0714824588533791,0.0744292845705114,0.0776622687632403,
0.0817097633391975,0.082658928079642),.UNSPECIFIED.);
#24151=B_SPLINE_CURVE_WITH_KNOTS('',3,(#150198,#150199,#150200,#150201,
#150202,#150203),.UNSPECIFIED.,.F.,.F.,(4,2,4),(1.49996604614892,1.51351365760524,
1.57686258992143),.UNSPECIFIED.);
#24152=B_SPLINE_CURVE_WITH_KNOTS('',3,(#150205,#150206,#150207,#150208,
#150209,#150210),.UNSPECIFIED.,.F.,.F.,(4,2,4),(1.33957856738739,1.40292749971882,
1.41647511118057),.UNSPECIFIED.);
#24153=B_SPLINE_CURVE_WITH_KNOTS('',3,(#150212,#150213,#150214,#150215,
#150216,#150217,#150218,#150219,#150220,#150221,#150222,#150223,#150224,
#150225,#150226,#150227,#150228,#150229,#150230),.UNSPECIFIED.,.F.,.F.,
(4,2,2,2,3,2,2,2,4),(0.0600992581812674,0.0615656152920304,0.0659612937560849,
0.0687970446603106,0.0714824588443023,0.0744292845619897,0.0776622687560912,
0.0817097633340036,0.0826589280667293),.UNSPECIFIED.);
#24154=B_SPLINE_CURVE_WITH_KNOTS('',3,(#150231,#150232,#150233,#150234,
#150235,#150236),.UNSPECIFIED.,.F.,.F.,(4,2,4),(1.49996604599013,1.51351365748729,
1.57686258978608),.UNSPECIFIED.);
#24155=B_SPLINE_CURVE_WITH_KNOTS('',3,(#150238,#150239,#150240,#150241,
#150242,#150243),.UNSPECIFIED.,.F.,.F.,(4,2,4),(1.33957856745805,1.40292749978122,
1.41647511124377),.UNSPECIFIED.);
#24156=B_SPLINE_CURVE_WITH_KNOTS('',3,(#150245,#150246,#150247,#150248,
#150249,#150250,#150251,#150252,#150253,#150254,#150255,#150256,#150257,
#150258,#150259,#150260,#150261,#150262,#150263),.UNSPECIFIED.,.F.,.F.,
(4,2,2,2,3,2,2,2,4),(0.0600992581991858,0.0615656152976462,0.0659612937615794,
0.0687970446662435,0.0714824588505711,0.074429284567676,0.0776622687616273,
0.08170976334013,0.0826589280525907),.UNSPECIFIED.);
#24157=B_SPLINE_CURVE_WITH_KNOTS('',3,(#150264,#150265,#150266,#150267,
#150268,#150269),.UNSPECIFIED.,.F.,.F.,(4,2,4),(1.49996604596708,1.51351365748614,
1.57686258973189),.UNSPECIFIED.);
#24158=B_SPLINE_CURVE_WITH_KNOTS('',3,(#150271,#150272,#150273,#150274,
#150275,#150276),.UNSPECIFIED.,.F.,.F.,(4,2,4),(1.33957856720859,1.40292749944731,
1.41647511096857),.UNSPECIFIED.);
#24159=B_SPLINE_CURVE_WITH_KNOTS('',3,(#150278,#150279,#150280,#150281,
#150282,#150283,#150284,#150285,#150286,#150287,#150288,#150289,#150290,
#150291,#150292,#150293,#150294,#150295,#150296),.UNSPECIFIED.,.F.,.F.,
(4,2,2,2,3,2,2,2,4),(0.0600992582031889,0.0615656152966673,0.0659612937648836,
0.0687970446710848,0.0714824588565221,0.0744292845736361,0.0776622687659337,
0.0817097633410083,0.0826589280509826),.UNSPECIFIED.);
#24160=B_SPLINE_CURVE_WITH_KNOTS('',3,(#150297,#150298,#150299,#150300,
#150301,#150302),.UNSPECIFIED.,.F.,.F.,(4,2,4),(1.49996604614752,1.51351365761189,
1.57686258994074),.UNSPECIFIED.);
#24161=B_SPLINE_CURVE_WITH_KNOTS('',3,(#150304,#150305,#150306,#150307,
#150308,#150309),.UNSPECIFIED.,.F.,.F.,(4,2,4),(1.33957856755016,1.40292749991405,
1.41647511134939),.UNSPECIFIED.);
#24162=B_SPLINE_CURVE_WITH_KNOTS('',3,(#150311,#150312,#150313,#150314,
#150315,#150316,#150317,#150318,#150319,#150320,#150321,#150322,#150323,
#150324,#150325,#150326,#150327,#150328,#150329),.UNSPECIFIED.,.F.,.F.,
(4,2,2,2,3,2,2,2,4),(0.0600992581724971,0.0615656152971063,0.0659612937590036,
0.0687970446626092,0.071482458846168,0.074429284563624,0.077662268758557,
0.0817097633385553,0.0826589280552966),.UNSPECIFIED.);
#24163=B_SPLINE_CURVE_WITH_KNOTS('',3,(#150330,#150331,#150332,#150333,
#150334,#150335),.UNSPECIFIED.,.F.,.F.,(4,2,4),(1.49996604592509,1.51351365746294,
1.57686258968125),.UNSPECIFIED.);
#24164=B_SPLINE_CURVE_WITH_KNOTS('',3,(#150337,#150338,#150339,#150340,
#150341,#150342),.UNSPECIFIED.,.F.,.F.,(4,2,4),(1.33957856728706,1.40292749954936,
1.41647511104989),.UNSPECIFIED.);
#24165=B_SPLINE_CURVE_WITH_KNOTS('',3,(#150344,#150345,#150346,#150347,
#150348,#150349,#150350,#150351,#150352,#150353,#150354,#150355,#150356,
#150357,#150358,#150359,#150360,#150361,#150362),.UNSPECIFIED.,.F.,.F.,
(4,2,2,2,3,2,2,2,4),(0.0600992581983925,0.0615656152984988,0.0659612937652178,
0.068797044671002,0.0714824588561452,0.0744292845731096,0.0776622687659398,
0.0817097633423463,0.0826589280639838),.UNSPECIFIED.);
#24166=B_SPLINE_CURVE_WITH_KNOTS('',3,(#150363,#150364,#150365,#150366,
#150367,#150368),.UNSPECIFIED.,.F.,.F.,(4,2,4),(1.49996604606541,1.51351365754495,
1.5768625898475),.UNSPECIFIED.);
#24167=B_SPLINE_CURVE_WITH_KNOTS('',3,(#150370,#150371,#150372,#150373,
#150374,#150375),.UNSPECIFIED.,.F.,.F.,(4,2,4),(1.339578567325,1.40292749961837,
1.41647511112636),.UNSPECIFIED.);
#24168=B_SPLINE_CURVE_WITH_KNOTS('',3,(#150377,#150378,#150379,#150380,
#150381,#150382,#150383,#150384,#150385,#150386,#150387,#150388,#150389,
#150390,#150391,#150392,#150393,#150394,#150395),.UNSPECIFIED.,.F.,.F.,
(4,2,2,2,3,2,2,2,4),(0.0600992581805974,0.0615656152925331,0.0659612937574204,
0.068797044661994,0.0714824588462428,0.0744292845638862,0.0776622687576387,
0.0817097633349189,0.0826589280661421),.UNSPECIFIED.);
#24169=B_SPLINE_CURVE_WITH_KNOTS('',3,(#150396,#150397,#150398,#150399,
#150400,#150401),.UNSPECIFIED.,.F.,.F.,(4,2,4),(1.49996604604551,1.51351365755335,
1.57686258982728),.UNSPECIFIED.);
#24170=B_SPLINE_CURVE_WITH_KNOTS('',3,(#150403,#150404,#150405,#150406,
#150407,#150408),.UNSPECIFIED.,.F.,.F.,(4,2,4),(1.33957856756908,1.40292749985976,
1.41647511133802),.UNSPECIFIED.);
#24171=B_SPLINE_CURVE_WITH_KNOTS('',3,(#150410,#150411,#150412,#150413,
#150414,#150415,#150416,#150417,#150418,#150419,#150420,#150421,#150422,
#150423,#150424,#150425,#150426,#150427,#150428),.UNSPECIFIED.,.F.,.F.,
(4,2,2,2,3,2,2,2,4),(0.0600992581791887,0.061565615297314,0.0659612937603919,
0.0687970446645219,0.071482458848452,0.0744292845657981,0.0776622687602112,
0.0817097633392904,0.0826589280661775),.UNSPECIFIED.);
#24172=B_SPLINE_CURVE_WITH_KNOTS('',3,(#150429,#150430,#150431,#150432,
#150433,#150434),.UNSPECIFIED.,.F.,.F.,(4,2,4),(1.4999660459877,1.51351365748924,
1.57686258975018),.UNSPECIFIED.);
#24173=B_SPLINE_CURVE_WITH_KNOTS('',3,(#150436,#150437,#150438,#150439,
#150440,#150441),.UNSPECIFIED.,.F.,.F.,(4,2,4),(1.33957856709288,1.40292749934161,
1.41647511088272),.UNSPECIFIED.);
#24174=B_SPLINE_CURVE_WITH_KNOTS('',3,(#150443,#150444,#150445,#150446,
#150447,#150448,#150449,#150450,#150451,#150452,#150453,#150454,#150455,
#150456,#150457,#150458,#150459,#150460,#150461),.UNSPECIFIED.,.F.,.F.,
(4,2,2,2,3,2,2,2,4),(0.0600992582807806,0.0615656153031256,0.0659612937734699,
0.0687970446812232,0.0714824588678127,0.0744292845840066,0.0776622687751647,
0.081709763349313,0.0826589280274163),.UNSPECIFIED.);
#24175=B_SPLINE_CURVE_WITH_KNOTS('',3,(#150462,#150463,#150464,#150465,
#150466,#150467),.UNSPECIFIED.,.F.,.F.,(4,2,4),(1.4999660461432,1.51351365759822,
1.57686258991855),.UNSPECIFIED.);
#24176=B_SPLINE_CURVE_WITH_KNOTS('',3,(#150469,#150470,#150471,#150472,
#150473,#150474),.UNSPECIFIED.,.F.,.F.,(4,2,4),(1.33957856765486,1.40292749999358,
1.41647511145339),.UNSPECIFIED.);
#24177=B_SPLINE_CURVE_WITH_KNOTS('',3,(#150476,#150477,#150478,#150479,
#150480,#150481,#150482,#150483,#150484,#150485,#150486,#150487,#150488,
#150489,#150490,#150491,#150492,#150493,#150494),.UNSPECIFIED.,.F.,.F.,
(4,2,2,2,3,2,2,2,4),(0.0600992582266854,0.0615656153023148,0.0659612937643017,
0.0687970446683665,0.0714824588522693,0.074429284569195,0.0776622687639236,
0.0817097633443078,0.0826589280394227),.UNSPECIFIED.);
#24178=B_SPLINE_CURVE_WITH_KNOTS('',3,(#150495,#150496,#150497,#150498,
#150499,#150500),.UNSPECIFIED.,.F.,.F.,(4,2,4),(1.49996604590169,1.51351365744857,
1.57686258967832),.UNSPECIFIED.);
#24179=B_SPLINE_CURVE_WITH_KNOTS('',3,(#150502,#150503,#150504,#150505,
#150506,#150507),.UNSPECIFIED.,.F.,.F.,(4,2,4),(1.33957856772042,1.40292750007181,
1.41647511151978),.UNSPECIFIED.);
#24180=B_SPLINE_CURVE_WITH_KNOTS('',3,(#150509,#150510,#150511,#150512,
#150513,#150514,#150515,#150516,#150517,#150518,#150519,#150520,#150521,
#150522,#150523,#150524,#150525,#150526,#150527),.UNSPECIFIED.,.F.,.F.,
(4,2,2,2,3,2,2,2,4),(0.0600992581728462,0.0615656152980507,0.0659612937585695,
0.068797044661703,0.0714824588449131,0.0744292845623147,0.0776622687577505,
0.0817097633388566,0.0826589280376275),.UNSPECIFIED.);
#24181=B_SPLINE_CURVE_WITH_KNOTS('',3,(#150528,#150529,#150530,#150531,
#150532,#150533),.UNSPECIFIED.,.F.,.F.,(4,2,4),(1.4999660458686,1.5135136573944,
1.576862589611),.UNSPECIFIED.);
#24182=B_SPLINE_CURVE_WITH_KNOTS('',3,(#150535,#150536,#150537,#150538,
#150539,#150540),.UNSPECIFIED.,.F.,.F.,(4,2,4),(1.33957856717928,1.4029274994472,
1.416475110961),.UNSPECIFIED.);
#24183=B_SPLINE_CURVE_WITH_KNOTS('',3,(#150542,#150543,#150544,#150545,
#150546,#150547,#150548,#150549,#150550,#150551,#150552,#150553,#150554,
#150555,#150556,#150557,#150558,#150559,#150560),.UNSPECIFIED.,.F.,.F.,
(4,2,2,2,3,2,2,2,4),(0.0600992582615478,0.061565615298571,0.0659612937676607,
0.0687970446745707,0.0714824588605384,0.0744292845772193,0.0776622687689834,
0.081709763343638,0.082658928152003),.UNSPECIFIED.);
#24184=B_SPLINE_CURVE_WITH_KNOTS('',3,(#150561,#150562,#150563,#150564,
#150565,#150566),.UNSPECIFIED.,.F.,.F.,(4,2,4),(1.49996604619025,1.51351365761973,
1.57686258985598),.UNSPECIFIED.);
#24185=B_SPLINE_CURVE_WITH_KNOTS('',3,(#150568,#150569,#150570,#150571,
#150572,#150573),.UNSPECIFIED.,.F.,.F.,(4,2,4),(1.33957856748694,1.40292749977602,
1.41647511126263),.UNSPECIFIED.);
#24186=B_SPLINE_CURVE_WITH_KNOTS('',3,(#150575,#150576,#150577,#150578,
#150579,#150580,#150581,#150582,#150583,#150584,#150585,#150586,#150587,
#150588,#150589,#150590,#150591,#150592,#150593),.UNSPECIFIED.,.F.,.F.,
(4,2,2,2,3,2,2,2,4),(0.0600992581602822,0.0615656152932241,0.0659612937568336,
0.0687970446610076,0.0714824588449648,0.0744292845625697,0.0776622687567982,
0.0817097633351034,0.0826589280710592),.UNSPECIFIED.);
#24187=B_SPLINE_CURVE_WITH_KNOTS('',3,(#150594,#150595,#150596,#150597,
#150598,#150599),.UNSPECIFIED.,.F.,.F.,(4,2,4),(1.49996604600395,1.51351365751376,
1.57686258978941),.UNSPECIFIED.);
#24188=B_SPLINE_CURVE_WITH_KNOTS('',3,(#150601,#150602,#150603,#150604,
#150605,#150606),.UNSPECIFIED.,.F.,.F.,(4,2,4),(1.33957856740119,1.40292749970377,
1.41647511119406),.UNSPECIFIED.);
#24189=B_SPLINE_CURVE_WITH_KNOTS('',3,(#150608,#150609,#150610,#150611,
#150612,#150613,#150614,#150615,#150616,#150617,#150618,#150619,#150620,
#150621,#150622,#150623,#150624,#150625,#150626),.UNSPECIFIED.,.F.,.F.,
(4,2,2,2,3,2,2,2,4),(0.060099258212016,0.0615656152975696,0.065961293762618,
0.0687970446677243,0.0714824588523708,0.0744292845694441,0.077662268762938,
0.0817097633405424,0.0826589280599493),.UNSPECIFIED.);
#24190=B_SPLINE_CURVE_WITH_KNOTS('',3,(#150627,#150628,#150629,#150630,
#150631,#150632),.UNSPECIFIED.,.F.,.F.,(4,2,4),(1.49996604599116,1.51351365749285,
1.57686258976734),.UNSPECIFIED.);
#24191=B_SPLINE_CURVE_WITH_KNOTS('',3,(#150634,#150635,#150636,#150637,
#150638,#150639),.UNSPECIFIED.,.F.,.F.,(4,2,4),(1.33957856732668,1.4029274996563,
1.41647511113565),.UNSPECIFIED.);
#24192=B_SPLINE_CURVE_WITH_KNOTS('',3,(#150641,#150642,#150643,#150644,
#150645,#150646,#150647,#150648,#150649,#150650,#150651,#150652,#150653,
#150654,#150655,#150656,#150657,#150658,#150659),.UNSPECIFIED.,.F.,.F.,
(4,2,2,2,3,2,2,2,4),(0.0600992582419533,0.0615656153042786,0.0659612937703273,
0.0687970446762605,0.0714824588615259,0.0744292845780137,0.0776622687709749,
0.0817097633483941,0.0826589280099401),.UNSPECIFIED.);
#24193=B_SPLINE_CURVE_WITH_KNOTS('',3,(#150660,#150661,#150662,#150663,
#150664,#150665),.UNSPECIFIED.,.F.,.F.,(4,2,4),(1.49996604605517,1.51351365754508,
1.57686258984243),.UNSPECIFIED.);
#24194=B_SPLINE_CURVE_WITH_KNOTS('',3,(#150667,#150668,#150669,#150670,
#150671,#150672),.UNSPECIFIED.,.F.,.F.,(4,2,4),(1.33957856704589,1.4029274993359,
1.41647511085871),.UNSPECIFIED.);
#24195=B_SPLINE_CURVE_WITH_KNOTS('',3,(#150674,#150675,#150676,#150677,
#150678,#150679,#150680,#150681,#150682,#150683,#150684,#150685,#150686,
#150687,#150688,#150689,#150690,#150691,#150692),.UNSPECIFIED.,.F.,.F.,
(4,2,2,2,3,2,2,2,4),(0.060099258257199,0.0615656153000239,0.0659612937700476,
0.0687970446774007,0.0714824588636833,0.0744292845802365,0.0776622687716015,
0.0817097633456108,0.0826589280505602),.UNSPECIFIED.);
#24196=B_SPLINE_CURVE_WITH_KNOTS('',3,(#150693,#150694,#150695,#150696,
#150697,#150698),.UNSPECIFIED.,.F.,.F.,(4,2,4),(1.49996604621862,1.51351365765759,
1.57686259000692),.UNSPECIFIED.);
#24197=B_SPLINE_CURVE_WITH_KNOTS('',3,(#150700,#150701,#150702,#150703,
#150704,#150705),.UNSPECIFIED.,.F.,.F.,(4,2,4),(1.3395785672913,1.40292749959559,
1.41647511108348),.UNSPECIFIED.);
#24198=B_SPLINE_CURVE_WITH_KNOTS('',3,(#150707,#150708,#150709,#150710,
#150711,#150712,#150713,#150714,#150715,#150716,#150717,#150718,#150719,
#150720,#150721,#150722,#150723,#150724,#150725),.UNSPECIFIED.,.F.,.F.,
(4,2,2,2,3,2,2,2,4),(0.0600992582270211,0.0615656152977835,0.0659612937639702,
0.0687970446695299,0.0714824588545066,0.074429284571517,0.0776622687645759,
0.0817097633413757,0.0826589280368495),.UNSPECIFIED.);
#24199=B_SPLINE_CURVE_WITH_KNOTS('',3,(#150726,#150727,#150728,#150729,
#150730,#150731),.UNSPECIFIED.,.F.,.F.,(4,2,4),(1.49996604605924,1.51351365751903,
1.57686258982276),.UNSPECIFIED.);
#24200=B_SPLINE_CURVE_WITH_KNOTS('',3,(#150733,#150734,#150735,#150736,
#150737,#150738),.UNSPECIFIED.,.F.,.F.,(4,2,4),(1.33957856731211,1.40292749955525,
1.4164751110542),.UNSPECIFIED.);
#24201=B_SPLINE_CURVE_WITH_KNOTS('',3,(#150740,#150741,#150742,#150743,
#150744,#150745,#150746,#150747,#150748,#150749,#150750,#150751,#150752,
#150753,#150754,#150755,#150756,#150757,#150758),.UNSPECIFIED.,.F.,.F.,
(4,2,2,2,3,2,2,2,4),(0.060099258176978,0.0615656152948672,0.0659612937615021,
0.0687970446670143,0.0714824588519459,0.074429284569227,0.0776622687621662,
0.0817097633383036,0.0826589280868534),.UNSPECIFIED.);
#24202=B_SPLINE_CURVE_WITH_KNOTS('',3,(#150759,#150760,#150761,#150762,
#150763,#150764),.UNSPECIFIED.,.F.,.F.,(4,2,4),(1.49996604610752,1.51351365759858,
1.57686258989254),.UNSPECIFIED.);
#24203=B_SPLINE_CURVE_WITH_KNOTS('',3,(#150766,#150767,#150768,#150769,
#150770,#150771),.UNSPECIFIED.,.F.,.F.,(4,2,4),(1.33957856760233,1.4029274999419,
1.41647511136569),.UNSPECIFIED.);
#24204=B_SPLINE_CURVE_WITH_KNOTS('',3,(#150773,#150774,#150775,#150776,
#150777,#150778,#150779,#150780,#150781,#150782,#150783,#150784,#150785,
#150786,#150787,#150788,#150789,#150790,#150791),.UNSPECIFIED.,.F.,.F.,
(4,2,2,2,3,2,2,2,4),(0.0600992582006083,0.0615656152993787,0.0659612937621229,
0.0687970446662533,0.0714824588501957,0.074429284567377,0.077662268761885,
0.0817097633414269,0.0826589280679091),.UNSPECIFIED.);
#24205=B_SPLINE_CURVE_WITH_KNOTS('',3,(#150792,#150793,#150794,#150795,
#150796,#150797),.UNSPECIFIED.,.F.,.F.,(4,2,4),(1.49996604589159,1.51351365742793,
1.5768625896485),.UNSPECIFIED.);
#24206=B_SPLINE_CURVE_WITH_KNOTS('',3,(#150799,#150800,#150801,#150802,
#150803,#150804),.UNSPECIFIED.,.F.,.F.,(4,2,4),(1.33957856743351,1.40292749973926,
1.41647511120219),.UNSPECIFIED.);
#24207=B_SPLINE_CURVE_WITH_KNOTS('',3,(#150806,#150807,#150808,#150809,
#150810,#150811,#150812,#150813,#150814,#150815,#150816,#150817,#150818,
#150819,#150820,#150821,#150822,#150823,#150824),.UNSPECIFIED.,.F.,.F.,
(4,2,2,2,3,2,2,2,4),(0.060099258224181,0.0615656153018815,0.0659612937669439,
0.0687970446723313,0.071482458857192,0.0744292845739036,0.0776622687673117,
0.0817097633452999,0.0826589280405905),.UNSPECIFIED.);
#24208=B_SPLINE_CURVE_WITH_KNOTS('',3,(#150825,#150826,#150827,#150828,
#150829,#150830),.UNSPECIFIED.,.F.,.F.,(4,2,4),(1.4999660459941,1.51351365749675,
1.57686258976619),.UNSPECIFIED.);
#24209=B_SPLINE_CURVE_WITH_KNOTS('',3,(#150832,#150833,#150834,#150835,
#150836,#150837),.UNSPECIFIED.,.F.,.F.,(4,2,4),(1.33957856743393,1.40292749973875,
1.41647511122195),.UNSPECIFIED.);
#24210=B_SPLINE_CURVE_WITH_KNOTS('',3,(#150839,#150840,#150841,#150842,
#150843,#150844,#150845,#150846,#150847,#150848,#150849,#150850,#150851,
#150852,#150853,#150854,#150855,#150856,#150857),.UNSPECIFIED.,.F.,.F.,
(4,2,2,2,3,2,2,2,4),(0.0600992582578962,0.0615656153040005,0.0659612937693774,
0.0687970446751162,0.0714824588602392,0.0744292845766818,0.0776622687698639,
0.0817097633478017,0.0826589280085131),.UNSPECIFIED.);
#24211=B_SPLINE_CURVE_WITH_KNOTS('',3,(#150858,#150859,#150860,#150861,
#150862,#150863),.UNSPECIFIED.,.F.,.F.,(4,2,4),(1.49996604599272,1.51351365750804,
1.5768625897927),.UNSPECIFIED.);
#24212=B_SPLINE_CURVE_WITH_KNOTS('',3,(#150865,#150866,#150867,#150868,
#150869,#150870),.UNSPECIFIED.,.F.,.F.,(4,2,4),(1.33957856741527,1.40292749969865,
1.41647511118214),.UNSPECIFIED.);
#24213=B_SPLINE_CURVE_WITH_KNOTS('',3,(#150872,#150873,#150874,#150875,
#150876,#150877,#150878,#150879,#150880,#150881,#150882,#150883,#150884,
#150885,#150886,#150887,#150888,#150889,#150890),.UNSPECIFIED.,.F.,.F.,
(4,2,2,2,3,2,2,2,4),(-0.0111764691682505,-0.0102273044870354,-0.00617980990966401,
-0.00294682571662145,0.,0.00268541418514354,0.005521165090919,0.00991684355683096,
0.0113832006132941),.UNSPECIFIED.);
#24214=B_SPLINE_CURVE_WITH_KNOTS('',3,(#150891,#150892,#150893,#150894,
#150895,#150896),.UNSPECIFIED.,.F.,.F.,(4,2,4),(1.49996604605074,1.51351365753382,
1.57686258981781),.UNSPECIFIED.);
#24215=B_SPLINE_CURVE_WITH_KNOTS('',3,(#150898,#150899,#150900,#150901,
#150902,#150903),.UNSPECIFIED.,.F.,.F.,(4,2,4),(1.33957856730954,1.40292749963475,
1.41647511111458),.UNSPECIFIED.);
#24216=B_SPLINE_CURVE_WITH_KNOTS('',3,(#150905,#150906,#150907,#150908,
#150909,#150910,#150911,#150912,#150913,#150914,#150915,#150916,#150917,
#150918,#150919,#150920,#150921,#150922,#150923),.UNSPECIFIED.,.F.,.F.,
(4,2,2,2,3,2,2,2,4),(0.0600992582697307,0.061565615304837,0.065961293771895,
0.0687970446782751,0.0714824588638683,0.0744292845802308,0.0776622687727685,
0.0817097633495057,0.0826589280210248),.UNSPECIFIED.);
#24217=B_SPLINE_CURVE_WITH_KNOTS('',3,(#150924,#150925,#150926,#150927,
#150928,#150929),.UNSPECIFIED.,.F.,.F.,(4,2,4),(1.499966046113,1.51351365756774,
1.57686258990272),.UNSPECIFIED.);
#24218=B_SPLINE_CURVE_WITH_KNOTS('',3,(#150931,#150932,#150933,#150934,
#150935,#150936),.UNSPECIFIED.,.F.,.F.,(4,2,4),(1.33957856732956,1.40292749963323,
1.41647511110724),.UNSPECIFIED.);
#24219=B_SPLINE_CURVE_WITH_KNOTS('',3,(#150938,#150939,#150940,#150941,
#150942,#150943,#150944,#150945,#150946,#150947,#150948,#150949,#150950,
#150951,#150952,#150953,#150954,#150955,#150956),.UNSPECIFIED.,.F.,.F.,
(4,2,2,2,3,2,2,2,4),(0.0600992582313051,0.06156561530149,0.0659612937681241,
0.0687970446741513,0.0714824588594794,0.0744292845761104,0.0776622687688761,
0.0817097633456649,0.0826589280244371),.UNSPECIFIED.);
#24220=B_SPLINE_CURVE_WITH_KNOTS('',3,(#150957,#150958,#150959,#150960,
#150961,#150962),.UNSPECIFIED.,.F.,.F.,(4,2,4),(1.49996604607698,1.51351365757267,
1.57686258986461),.UNSPECIFIED.);
#24221=B_SPLINE_CURVE_WITH_KNOTS('',3,(#150964,#150965,#150966,#150967,
#150968,#150969),.UNSPECIFIED.,.F.,.F.,(4,2,4),(1.33957856716701,1.40292749942639,
1.41647511094955),.UNSPECIFIED.);
#24222=B_SPLINE_CURVE_WITH_KNOTS('',3,(#150971,#150972,#150973,#150974,
#150975,#150976,#150977,#150978,#150979,#150980,#150981,#150982,#150983,
#150984,#150985,#150986,#150987,#150988,#150989),.UNSPECIFIED.,.F.,.F.,
(4,2,2,2,3,2,2,2,4),(0.0600992582098331,0.0615656152973585,0.0659612937652959,
0.0687970446716145,0.0714824588571425,0.0744292845740375,0.0776622687663252,
0.081709763341718,0.0826589280631378),.UNSPECIFIED.);
#24223=B_SPLINE_CURVE_WITH_KNOTS('',3,(#150990,#150991,#150992,#150993,
#150994,#150995),.UNSPECIFIED.,.F.,.F.,(4,2,4),(1.49996604614834,1.51351365759482,
1.5768625899084),.UNSPECIFIED.);
#24224=B_SPLINE_CURVE_WITH_KNOTS('',3,(#150997,#150998,#150999,#151000,
#151001,#151002),.UNSPECIFIED.,.F.,.F.,(4,2,4),(1.33957856752927,1.40292749981418,
1.41647511131301),.UNSPECIFIED.);
#24225=B_SPLINE_CURVE_WITH_KNOTS('',3,(#151004,#151005,#151006,#151007,
#151008,#151009,#151010,#151011,#151012,#151013,#151014,#151015,#151016,
#151017,#151018,#151019,#151020,#151021,#151022),.UNSPECIFIED.,.F.,.F.,
(4,2,2,2,3,2,2,2,4),(0.0600992581691034,0.0615656152957655,0.0659612937588952,
0.0687970446629439,0.0714824588468164,0.0744292845642891,0.0776622687587119,
0.0817097633376232,0.08265892807845),.UNSPECIFIED.);
#24226=B_SPLINE_CURVE_WITH_KNOTS('',3,(#151023,#151024,#151025,#151026,
#151027,#151028),.UNSPECIFIED.,.F.,.F.,(4,2,4),(1.49996604595889,1.51351365749176,
1.57686258972957),.UNSPECIFIED.);
#24227=B_SPLINE_CURVE_WITH_KNOTS('',3,(#151030,#151031,#151032,#151033,
#151034,#151035),.UNSPECIFIED.,.F.,.F.,(4,2,4),(1.33957856752258,1.40292749978992,
1.41647511126154),.UNSPECIFIED.);
#24228=B_SPLINE_CURVE_WITH_KNOTS('',3,(#151037,#151038,#151039,#151040,
#151041,#151042,#151043,#151044,#151045,#151046,#151047,#151048,#151049,
#151050,#151051,#151052,#151053,#151054,#151055),.UNSPECIFIED.,.F.,.F.,
(4,2,2,2,3,2,2,2,4),(0.0600992582008816,0.06156561529844,0.0659612937628877,
0.0687970446677415,0.0714824588522039,0.0744292845693024,0.0776622687630662,
0.0817097633411937,0.0826589280350822),.UNSPECIFIED.);
#24229=B_SPLINE_CURVE_WITH_KNOTS('',3,(#151056,#151057,#151058,#151059,
#151060,#151061),.UNSPECIFIED.,.F.,.F.,(4,2,4),(1.49996604601405,1.51351365750494,
1.57686258982047),.UNSPECIFIED.);
#24230=B_SPLINE_CURVE_WITH_KNOTS('',3,(#151063,#151064,#151065,#151066,
#151067,#151068),.UNSPECIFIED.,.F.,.F.,(4,2,4),(1.33957856772149,1.40292750006868,
1.41647511150784),.UNSPECIFIED.);
#24231=B_SPLINE_CURVE_WITH_KNOTS('',3,(#151070,#151071,#151072,#151073,
#151074,#151075,#151076,#151077,#151078,#151079,#151080,#151081,#151082,
#151083,#151084,#151085,#151086,#151087,#151088),.UNSPECIFIED.,.F.,.F.,
(4,2,2,2,3,2,2,2,4),(0.0600992582202586,0.0615656153022612,0.0659612937636604,
0.0687970446674222,0.0714824588511022,0.0744292845681201,0.0776622687631126,
0.0817097633439068,0.0826589280118024),.UNSPECIFIED.);
#24232=B_SPLINE_CURVE_WITH_KNOTS('',3,(#151089,#151090,#151091,#151092,
#151093,#151094),.UNSPECIFIED.,.F.,.F.,(4,2,4),(1.49996604587209,1.51351365743327,
1.57686258967902),.UNSPECIFIED.);
#24233=B_SPLINE_CURVE_WITH_KNOTS('',3,(#151096,#151097,#151098,#151099,
#151100,#151101),.UNSPECIFIED.,.F.,.F.,(4,2,4),(1.33957856735936,1.40292749966726,
1.41647511117744),.UNSPECIFIED.);
#24234=B_SPLINE_CURVE_WITH_KNOTS('',3,(#151103,#151104,#151105,#151106,
#151107,#151108,#151109,#151110,#151111,#151112,#151113,#151114,#151115,
#151116,#151117,#151118,#151119,#151120,#151121),.UNSPECIFIED.,.F.,.F.,
(4,2,2,2,3,2,2,2,4),(0.060099258266917,0.0615656153034342,0.0659612937695933,
0.0687970446755725,0.0714824588608685,0.0744292845773433,0.0776622687702354,
0.08170976334752,0.0826589280354621),.UNSPECIFIED.);
#24235=B_SPLINE_CURVE_WITH_KNOTS('',3,(#151122,#151123,#151124,#151125,
#151126,#151127),.UNSPECIFIED.,.F.,.F.,(4,2,4),(1.49996604600415,1.51351365750855,
1.57686258981381),.UNSPECIFIED.);
#24236=B_SPLINE_CURVE_WITH_KNOTS('',3,(#151129,#151130,#151131,#151132,
#151133,#151134),.UNSPECIFIED.,.F.,.F.,(4,2,4),(1.33957856738494,1.40292749967249,
1.41647511116503),.UNSPECIFIED.);
#24237=B_SPLINE_CURVE_WITH_KNOTS('',3,(#151136,#151137,#151138,#151139,
#151140,#151141,#151142,#151143,#151144,#151145,#151146,#151147,#151148,
#151149,#151150,#151151,#151152,#151153,#151154),.UNSPECIFIED.,.F.,.F.,
(4,2,2,2,3,2,2,2,4),(0.0600992582018194,0.0615656152977379,0.0659612937632103,
0.0687970446684834,0.0714824588532511,0.0744292845703054,0.0776622687636379,
0.0817097633409366,0.0826589280495915),.UNSPECIFIED.);
#24238=B_SPLINE_CURVE_WITH_KNOTS('',3,(#151155,#151156,#151157,#151158,
#151159,#151160),.UNSPECIFIED.,.F.,.F.,(4,2,4),(1.49996604604657,1.51351365754362,
1.57686258983577),.UNSPECIFIED.);
#24239=B_SPLINE_CURVE_WITH_KNOTS('',3,(#151162,#151163,#151164,#151165,
#151166,#151167),.UNSPECIFIED.,.F.,.F.,(4,2,4),(1.33957856727904,1.40292749957447,
1.41647511106942),.UNSPECIFIED.);
#24240=B_SPLINE_CURVE_WITH_KNOTS('',3,(#151169,#151170,#151171,#151172,
#151173,#151174,#151175,#151176,#151177,#151178,#151179,#151180,#151181,
#151182,#151183,#151184,#151185,#151186,#151187),.UNSPECIFIED.,.F.,.F.,
(4,2,2,2,3,2,2,2,4),(0.0600992581788355,0.0615656152931474,0.0659612937586987,
0.0687970446636357,0.071482458848146,0.0744292845656479,0.077662268759093,
0.0817097633359387,0.082658928090395),.UNSPECIFIED.);
#24241=B_SPLINE_CURVE_WITH_KNOTS('',3,(#151188,#151189,#151190,#151191,
#151192,#151193),.UNSPECIFIED.,.F.,.F.,(4,2,4),(1.49996604606282,1.51351365753196,
1.57686258981422),.UNSPECIFIED.);
#24242=B_SPLINE_CURVE_WITH_KNOTS('',3,(#151195,#151196,#151197,#151198,
#151199,#151200),.UNSPECIFIED.,.F.,.F.,(4,2,4),(1.33957856759874,1.40292749993747,
1.41647511140743),.UNSPECIFIED.);
#24243=B_SPLINE_CURVE_WITH_KNOTS('',3,(#151202,#151203,#151204,#151205,
#151206,#151207,#151208,#151209,#151210,#151211,#151212,#151213,#151214,
#151215,#151216,#151217,#151218,#151219,#151220),.UNSPECIFIED.,.F.,.F.,
(4,2,2,2,3,2,2,2,4),(0.0600992582012018,0.0615656153010839,0.0659612937631288,
0.0687970446670921,0.0714824588509169,0.0744292845679796,0.0776622687627298,
0.0817097633429504,0.08265892801506),.UNSPECIFIED.);
#24244=B_SPLINE_CURVE_WITH_KNOTS('',3,(#151221,#151222,#151223,#151224,
#151225,#151226),.UNSPECIFIED.,.F.,.F.,(4,2,4),(1.49996604591879,1.51351365743313,
1.57686258971772),.UNSPECIFIED.);
#24245=B_SPLINE_CURVE_WITH_KNOTS('',3,(#151228,#151229,#151230,#151231,
#151232,#151233),.UNSPECIFIED.,.F.,.F.,(4,2,4),(1.3395785670504,1.40292749929253,
1.41647511082944),.UNSPECIFIED.);
#24246=B_SPLINE_CURVE_WITH_KNOTS('',3,(#151235,#151236,#151237,#151238,
#151239,#151240,#151241,#151242,#151243,#151244,#151245,#151246,#151247,
#151248,#151249,#151250,#151251,#151252,#151253),.UNSPECIFIED.,.F.,.F.,
(4,2,2,2,3,2,2,2,4),(0.0600992582211251,0.0615656152958374,0.0659612937656703,
0.0687970446726791,0.0714824588587041,0.0744292845756083,0.0776622687671392,
0.0817097633409514,0.0826589280881341),.UNSPECIFIED.);
#24247=B_SPLINE_CURVE_WITH_KNOTS('',3,(#151254,#151255,#151256,#151257,
#151258,#151259),.UNSPECIFIED.,.F.,.F.,(4,2,4),(1.49996604617379,1.51351365761947,
1.5768625899443),.UNSPECIFIED.);
#24248=B_SPLINE_CURVE_WITH_KNOTS('',3,(#151261,#151262,#151263,#151264,
#151265,#151266),.UNSPECIFIED.,.F.,.F.,(4,2,4),(1.33957856714172,1.40292749936937,
1.41647511087422),.UNSPECIFIED.);
#24249=B_SPLINE_CURVE_WITH_KNOTS('',3,(#151268,#151269,#151270,#151271,
#151272,#151273,#151274,#151275,#151276,#151277,#151278,#151279,#151280,
#151281,#151282,#151283,#151284,#151285,#151286),.UNSPECIFIED.,.F.,.F.,
(4,2,2,2,3,2,2,2,4),(0.0600992582311416,0.0615656153003289,0.0659612937699029,
0.0687970446771266,0.0714824588633188,0.0744292845798336,0.0776622687713656,
0.0817097633457816,0.0826589280447636),.UNSPECIFIED.);
#24250=B_SPLINE_CURVE_WITH_KNOTS('',3,(#151287,#151288,#151289,#151290,
#151291,#151292),.UNSPECIFIED.,.F.,.F.,(4,2,4),(1.4999660461885,1.51351365763824,
1.57686258995467),.UNSPECIFIED.);
#24251=B_SPLINE_CURVE_WITH_KNOTS('',3,(#151294,#151295,#151296,#151297,
#151298,#151299),.UNSPECIFIED.,.F.,.F.,(4,2,4),(1.33957856767546,1.402927500014,
1.41647511143919),.UNSPECIFIED.);
#24252=B_SPLINE_CURVE_WITH_KNOTS('',3,(#151301,#151302,#151303,#151304,
#151305,#151306,#151307,#151308,#151309,#151310,#151311,#151312,#151313,
#151314,#151315,#151316,#151317,#151318,#151319),.UNSPECIFIED.,.F.,.F.,
(4,2,2,2,3,2,2,2,4),(0.0600992582047541,0.0615656153054466,0.0659612937675513,
0.0687970446718945,0.0714824588560064,0.0744292845726366,0.0776622687672277,
0.0817097633477888,0.0826589279966098),.UNSPECIFIED.);
#24253=B_SPLINE_CURVE_WITH_KNOTS('',3,(#151320,#151321,#151322,#151323,
#151324,#151325),.UNSPECIFIED.,.F.,.F.,(4,2,4),(1.49996604592437,1.51351365744584,
1.57686258971838),.UNSPECIFIED.);
#24254=B_SPLINE_CURVE_WITH_KNOTS('',3,(#151327,#151328,#151329,#151330,
#151331,#151332),.UNSPECIFIED.,.F.,.F.,(4,2,4),(1.33957856718658,1.40292749947563,
1.41647511098612),.UNSPECIFIED.);
#24255=B_SPLINE_CURVE_WITH_KNOTS('',3,(#151334,#151335,#151336,#151337,
#151338,#151339,#151340,#151341,#151342,#151343,#151344,#151345,#151346,
#151347,#151348,#151349,#151350,#151351,#151352),.UNSPECIFIED.,.F.,.F.,
(4,2,2,2,3,2,2,2,4),(0.0600992581925589,0.0615656152960413,0.0659612937631332,
0.0687970446689342,0.0714824588540824,0.0744292845712135,0.0776622687639362,
0.0817097633398639,0.0826589280802992),.UNSPECIFIED.);
#24256=B_SPLINE_CURVE_WITH_KNOTS('',3,(#151353,#151354,#151355,#151356,
#151357,#151358),.UNSPECIFIED.,.F.,.F.,(4,2,4),(1.49996604614893,1.51351365760524,
1.57686258992143),.UNSPECIFIED.);
#24257=B_SPLINE_CURVE_WITH_KNOTS('',3,(#151360,#151361,#151362,#151363,
#151364,#151365),.UNSPECIFIED.,.F.,.F.,(4,2,4),(1.33957856738739,1.40292749971882,
1.41647511118057),.UNSPECIFIED.);
#24258=B_SPLINE_CURVE_WITH_KNOTS('',3,(#151367,#151368,#151369,#151370,
#151371,#151372,#151373,#151374,#151375,#151376,#151377,#151378,#151379,
#151380,#151381,#151382,#151383,#151384,#151385),.UNSPECIFIED.,.F.,.F.,
(4,2,2,2,3,2,2,2,4),(0.0600992581815467,0.0615656152923098,0.0659612937563671,
0.0687970446605909,0.0714824588445816,0.0744292845622686,0.07766226875637,
0.0817097633342855,0.082658928067012),.UNSPECIFIED.);
#24259=B_SPLINE_CURVE_WITH_KNOTS('',3,(#151386,#151387,#151388,#151389,
#151390,#151391),.UNSPECIFIED.,.F.,.F.,(4,2,4),(1.49996604599013,1.51351365748729,
1.57686258978608),.UNSPECIFIED.);
#24260=B_SPLINE_CURVE_WITH_KNOTS('',3,(#151393,#151394,#151395,#151396,
#151397,#151398),.UNSPECIFIED.,.F.,.F.,(4,2,4),(1.33957856745805,1.40292749978122,
1.41647511124377),.UNSPECIFIED.);
#24261=B_SPLINE_CURVE_WITH_KNOTS('',3,(#151400,#151401,#151402,#151403,
#151404,#151405,#151406,#151407,#151408,#151409,#151410,#151411,#151412,
#151413,#151414,#151415,#151416,#151417,#151418),.UNSPECIFIED.,.F.,.F.,
(4,2,2,2,3,2,2,2,4),(0.060099258200665,0.0615656152991906,0.0659612937632194,
0.0687970446678825,0.0714824588522107,0.0744292845693193,0.0776622687632825,
0.0817097633418088,0.0826589280542763),.UNSPECIFIED.);
#24262=B_SPLINE_CURVE_WITH_KNOTS('',3,(#151419,#151420,#151421,#151422,
#151423,#151424),.UNSPECIFIED.,.F.,.F.,(4,2,4),(1.49996604596708,1.51351365748613,
1.57686258973189),.UNSPECIFIED.);
#24263=B_SPLINE_CURVE_WITH_KNOTS('',3,(#151426,#151427,#151428,#151429,
#151430,#151431),.UNSPECIFIED.,.F.,.F.,(4,2,4),(1.33957856720859,1.40292749944731,
1.41647511096857),.UNSPECIFIED.);
#24264=B_SPLINE_CURVE_WITH_KNOTS('',3,(#151433,#151434,#151435,#151436,
#151437,#151438,#151439,#151440,#151441,#151442,#151443,#151444,#151445,
#151446,#151447,#151448,#151449,#151450,#151451),.UNSPECIFIED.,.F.,.F.,
(4,2,2,2,3,2,2,2,4),(0.0600992582017895,0.0615656152951978,0.0659612937633217,
0.0687970446695219,0.0714824588549564,0.0744292845720686,0.0776622687643598,
0.0817097633394204,0.0826589280493914),.UNSPECIFIED.);
#24265=B_SPLINE_CURVE_WITH_KNOTS('',3,(#151452,#151453,#151454,#151455,
#151456,#151457),.UNSPECIFIED.,.F.,.F.,(4,2,4),(1.49996604614752,1.51351365761189,
1.57686258994074),.UNSPECIFIED.);
#24266=B_SPLINE_CURVE_WITH_KNOTS('',3,(#151459,#151460,#151461,#151462,
#151463,#151464),.UNSPECIFIED.,.F.,.F.,(4,2,4),(1.33957856755016,1.40292749991405,
1.41647511134939),.UNSPECIFIED.);
#24267=B_SPLINE_CURVE_WITH_KNOTS('',3,(#151466,#151467,#151468,#151469,
#151470,#151471,#151472,#151473,#151474,#151475,#151476,#151477,#151478,
#151479,#151480,#151481,#151482,#151483,#151484),.UNSPECIFIED.,.F.,.F.,
(4,2,2,2,3,2,2,2,4),(0.0600992581724155,0.0615656152970366,0.0659612937589684,
0.0687970446625868,0.0714824588461473,0.074429284563595,0.0776622687585028,
0.0817097633384532,0.0826589280551801),.UNSPECIFIED.);
#24268=B_SPLINE_CURVE_WITH_KNOTS('',3,(#151485,#151486,#151487,#151488,
#151489,#151490),.UNSPECIFIED.,.F.,.F.,(4,2,4),(1.49996604592509,1.51351365746294,
1.57686258968125),.UNSPECIFIED.);
#24269=B_SPLINE_CURVE_WITH_KNOTS('',3,(#151492,#151493,#151494,#151495,
#151496,#151497),.UNSPECIFIED.,.F.,.F.,(4,2,4),(1.33957856728705,1.40292749954936,
1.41647511104988),.UNSPECIFIED.);
#24270=B_SPLINE_CURVE_WITH_KNOTS('',3,(#151499,#151500,#151501,#151502,
#151503,#151504,#151505,#151506,#151507,#151508,#151509,#151510,#151511,
#151512,#151513,#151514,#151515,#151516,#151517),.UNSPECIFIED.,.F.,.F.,
(4,2,2,2,3,2,2,2,4),(0.0600992581982055,0.0615656152983017,0.0659612937650131,
0.0687970446708029,0.0714824588559478,0.0744292845729105,0.0776622687657356,
0.0817097633421375,0.0826589280637736),.UNSPECIFIED.);
#24271=B_SPLINE_CURVE_WITH_KNOTS('',3,(#151518,#151519,#151520,#151521,
#151522,#151523),.UNSPECIFIED.,.F.,.F.,(4,2,4),(1.49996604606541,1.51351365754495,
1.5768625898475),.UNSPECIFIED.);
#24272=B_SPLINE_CURVE_WITH_KNOTS('',3,(#151525,#151526,#151527,#151528,
#151529,#151530),.UNSPECIFIED.,.F.,.F.,(4,2,4),(1.339578567325,1.40292749961837,
1.41647511112636),.UNSPECIFIED.);
#24273=B_SPLINE_CURVE_WITH_KNOTS('',3,(#151532,#151533,#151534,#151535,
#151536,#151537,#151538,#151539,#151540,#151541,#151542,#151543,#151544,
#151545,#151546,#151547,#151548,#151549,#151550),.UNSPECIFIED.,.F.,.F.,
(4,2,2,2,3,2,2,2,4),(0.0600992581809373,0.0615656152928883,0.0659612937578001,
0.0687970446623745,0.0714824588466231,0.074429284564271,0.0776622687580358,
0.0817097633353215,0.0826589280665468),.UNSPECIFIED.);
#24274=B_SPLINE_CURVE_WITH_KNOTS('',3,(#151551,#151552,#151553,#151554,
#151555,#151556),.UNSPECIFIED.,.F.,.F.,(4,2,4),(1.49996604604552,1.51351365755335,
1.57686258982728),.UNSPECIFIED.);
#24275=B_SPLINE_CURVE_WITH_KNOTS('',3,(#151558,#151559,#151560,#151561,
#151562,#151563),.UNSPECIFIED.,.F.,.F.,(4,2,4),(1.33957856756908,1.40292749985976,
1.41647511133802),.UNSPECIFIED.);
#24276=B_SPLINE_CURVE_WITH_KNOTS('',3,(#151565,#151566,#151567,#151568,
#151569,#151570,#151571,#151572,#151573,#151574,#151575,#151576,#151577,
#151578,#151579,#151580,#151581,#151582,#151583),.UNSPECIFIED.,.F.,.F.,
(4,2,2,2,3,2,2,2,4),(0.0600992581792367,0.061565615297372,0.0659612937604539,
0.0687970446645766,0.0714824588485057,0.0744292845658528,0.0776622687602686,
0.0817097633393586,0.0826589280662485),.UNSPECIFIED.);
#24277=B_SPLINE_CURVE_WITH_KNOTS('',3,(#151584,#151585,#151586,#151587,
#151588,#151589),.UNSPECIFIED.,.F.,.F.,(4,2,4),(1.4999660459877,1.51351365748924,
1.57686258975018),.UNSPECIFIED.);
#24278=B_SPLINE_CURVE_WITH_KNOTS('',3,(#151591,#151592,#151593,#151594,
#151595,#151596),.UNSPECIFIED.,.F.,.F.,(4,2,4),(1.33957856709288,1.40292749934161,
1.41647511088272),.UNSPECIFIED.);
#24279=B_SPLINE_CURVE_WITH_KNOTS('',3,(#151598,#151599,#151600,#151601,
#151602,#151603,#151604,#151605,#151606,#151607,#151608,#151609,#151610,
#151611,#151612,#151613,#151614,#151615,#151616),.UNSPECIFIED.,.F.,.F.,
(4,2,2,2,3,2,2,2,4),(0.0600992582805735,0.0615656153028816,0.065961293773175,
0.0687970446809335,0.0714824588675231,0.07442928458371,0.0776622687748456,
0.0817097633489511,0.0826589280270409),.UNSPECIFIED.);
#24280=B_SPLINE_CURVE_WITH_KNOTS('',3,(#151617,#151618,#151619,#151620,
#151621,#151622),.UNSPECIFIED.,.F.,.F.,(4,2,4),(1.4999660461432,1.51351365759822,
1.57686258991855),.UNSPECIFIED.);
#24281=B_SPLINE_CURVE_WITH_KNOTS('',3,(#151624,#151625,#151626,#151627,
#151628,#151629),.UNSPECIFIED.,.F.,.F.,(4,2,4),(1.33957856765486,1.40292749999358,
1.41647511145339),.UNSPECIFIED.);
#24282=B_SPLINE_CURVE_WITH_KNOTS('',3,(#151631,#151632,#151633,#151634,
#151635,#151636,#151637,#151638,#151639,#151640,#151641,#151642,#151643,
#151644,#151645,#151646,#151647,#151648,#151649),.UNSPECIFIED.,.F.,.F.,
(4,2,2,2,3,2,2,2,4),(0.0600992582262742,0.0615656153018907,0.0659612937638662,
0.0687970446679375,0.0714824588518414,0.0744292845687624,0.0776622687634731,
0.0817097633438245,0.0826589280389295),.UNSPECIFIED.);
#24283=B_SPLINE_CURVE_WITH_KNOTS('',3,(#151650,#151651,#151652,#151653,
#151654,#151655),.UNSPECIFIED.,.F.,.F.,(4,2,4),(1.49996604590169,1.51351365744857,
1.57686258967832),.UNSPECIFIED.);
#24284=B_SPLINE_CURVE_WITH_KNOTS('',3,(#151657,#151658,#151659,#151660,
#151661,#151662),.UNSPECIFIED.,.F.,.F.,(4,2,4),(1.33957856772042,1.40292750007181,
1.41647511151978),.UNSPECIFIED.);
#24285=B_SPLINE_CURVE_WITH_KNOTS('',3,(#151664,#151665,#151666,#151667,
#151668,#151669,#151670,#151671,#151672,#151673,#151674,#151675,#151676,
#151677,#151678,#151679,#151680,#151681,#151682),.UNSPECIFIED.,.F.,.F.,
(4,2,2,2,3,2,2,2,4),(0.0600992581730512,0.0615656152982502,0.0659612937587487,
0.0687970446618746,0.0714824588450843,0.0744292845624935,0.0776622687579553,
0.0817097633391145,0.0826589280378999),.UNSPECIFIED.);
#24286=B_SPLINE_CURVE_WITH_KNOTS('',3,(#151683,#151684,#151685,#151686,
#151687,#151688),.UNSPECIFIED.,.F.,.F.,(4,2,4),(1.4999660458686,1.5135136573944,
1.576862589611),.UNSPECIFIED.);
#24287=B_SPLINE_CURVE_WITH_KNOTS('',3,(#151690,#151691,#151692,#151693,
#151694,#151695),.UNSPECIFIED.,.F.,.F.,(4,2,4),(1.33957856717928,1.4029274994472,
1.416475110961),.UNSPECIFIED.);
#24288=B_SPLINE_CURVE_WITH_KNOTS('',3,(#151697,#151698,#151699,#151700,
#151701,#151702,#151703,#151704,#151705,#151706,#151707,#151708,#151709,
#151710,#151711,#151712,#151713,#151714,#151715),.UNSPECIFIED.,.F.,.F.,
(4,2,2,2,3,2,2,2,4),(0.0600992582613176,0.0615656152983437,0.0659612937674522,
0.0687970446743743,0.0714824588603425,0.0744292845770165,0.0776622687687574,
0.0817097633433523,0.082658928151699),.UNSPECIFIED.);
#24289=B_SPLINE_CURVE_WITH_KNOTS('',3,(#151716,#151717,#151718,#151719,
#151720,#151721),.UNSPECIFIED.,.F.,.F.,(4,2,4),(1.49996604619025,1.51351365761973,
1.57686258985598),.UNSPECIFIED.);
#24290=B_SPLINE_CURVE_WITH_KNOTS('',3,(#151723,#151724,#151725,#151726,
#151727,#151728),.UNSPECIFIED.,.F.,.F.,(4,2,4),(1.33957856748694,1.40292749977602,
1.41647511126263),.UNSPECIFIED.);
#24291=B_SPLINE_CURVE_WITH_KNOTS('',3,(#151730,#151731,#151732,#151733,
#151734,#151735,#151736,#151737,#151738,#151739,#151740,#151741,#151742,
#151743,#151744,#151745,#151746,#151747,#151748),.UNSPECIFIED.,.F.,.F.,
(4,2,2,2,3,2,2,2,4),(0.0600992581608641,0.0615656152938688,0.0659612937575722,
0.0687970446617445,0.0714824588456999,0.0744292845632993,0.0776622687575126,
0.0817097633357957,0.0826589280717446),.UNSPECIFIED.);
#24292=B_SPLINE_CURVE_WITH_KNOTS('',3,(#151749,#151750,#151751,#151752,
#151753,#151754),.UNSPECIFIED.,.F.,.F.,(4,2,4),(1.49996604600395,1.51351365751376,
1.57686258978941),.UNSPECIFIED.);
#24293=B_SPLINE_CURVE_WITH_KNOTS('',3,(#151756,#151757,#151758,#151759,
#151760,#151761),.UNSPECIFIED.,.F.,.F.,(4,2,4),(1.33957856740119,1.40292749970377,
1.41647511119406),.UNSPECIFIED.);
#24294=B_SPLINE_CURVE_WITH_KNOTS('',3,(#151763,#151764,#151765,#151766,
#151767,#151768,#151769,#151770,#151771,#151772,#151773,#151774,#151775,
#151776,#151777,#151778,#151779,#151780,#151781),.UNSPECIFIED.,.F.,.F.,
(4,2,2,2,3,2,2,2,4),(0.0600992582120315,0.0615656152975978,0.0659612937626651,
0.0687970446677665,0.071482458852412,0.0744292845694908,0.077662268763002,
0.0817097633406405,0.0826589280600578),.UNSPECIFIED.);
#24295=B_SPLINE_CURVE_WITH_KNOTS('',3,(#151782,#151783,#151784,#151785,
#151786,#151787),.UNSPECIFIED.,.F.,.F.,(4,2,4),(1.49996604599116,1.51351365749285,
1.57686258976734),.UNSPECIFIED.);
#24296=B_SPLINE_CURVE_WITH_KNOTS('',3,(#151789,#151790,#151791,#151792,
#151793,#151794),.UNSPECIFIED.,.F.,.F.,(4,2,4),(1.33957856732664,1.40292749965626,
1.4164751111356),.UNSPECIFIED.);
#24297=B_SPLINE_CURVE_WITH_KNOTS('',3,(#151796,#151797,#151798,#151799,
#151800,#151801,#151802,#151803,#151804,#151805,#151806,#151807,#151808,
#151809,#151810,#151811,#151812,#151813,#151814),.UNSPECIFIED.,.F.,.F.,
(4,2,2,2,3,2,2,2,4),(0.0600992582417298,0.0615656153040711,0.0659612937701545,
0.0687970446760882,0.0714824588613524,0.0744292845778339,0.0776622687707767,
0.0817097633481624,0.0826589280096967),.UNSPECIFIED.);
#24298=B_SPLINE_CURVE_WITH_KNOTS('',3,(#151815,#151816,#151817,#151818,
#151819,#151820),.UNSPECIFIED.,.F.,.F.,(4,2,4),(1.49996604605517,1.51351365754508,
1.57686258984243),.UNSPECIFIED.);
#24299=B_SPLINE_CURVE_WITH_KNOTS('',3,(#151822,#151823,#151824,#151825,
#151826,#151827),.UNSPECIFIED.,.F.,.F.,(4,2,4),(1.33957856704589,1.4029274993359,
1.41647511085871),.UNSPECIFIED.);
#24300=B_SPLINE_CURVE_WITH_KNOTS('',3,(#151829,#151830,#151831,#151832,
#151833,#151834,#151835,#151836,#151837,#151838,#151839,#151840,#151841,
#151842,#151843,#151844,#151845,#151846,#151847),.UNSPECIFIED.,.F.,.F.,
(4,2,2,2,3,2,2,2,4),(0.0600992582564895,0.0615656152993143,0.065961293769343,
0.0687970446766933,0.0714824588629754,0.07442928457953,0.0776622687708993,
0.0817097633449113,0.0826589280498623),.UNSPECIFIED.);
#24301=B_SPLINE_CURVE_WITH_KNOTS('',3,(#151848,#151849,#151850,#151851,
#151852,#151853),.UNSPECIFIED.,.F.,.F.,(4,2,4),(1.49996604621862,1.51351365765759,
1.57686259000693),.UNSPECIFIED.);
#24302=B_SPLINE_CURVE_WITH_KNOTS('',3,(#151855,#151856,#151857,#151858,
#151859,#151860),.UNSPECIFIED.,.F.,.F.,(4,2,4),(1.3395785672913,1.40292749959559,
1.41647511108348),.UNSPECIFIED.);
#24303=B_SPLINE_CURVE_WITH_KNOTS('',3,(#151862,#151863,#151864,#151865,
#151866,#151867,#151868,#151869,#151870,#151871,#151872,#151873,#151874,
#151875,#151876,#151877,#151878,#151879,#151880),.UNSPECIFIED.,.F.,.F.,
(4,2,2,2,3,2,2,2,4),(0.0600992582278879,0.0615656152986711,0.0659612937648786,
0.0687970446704373,0.0714824588554149,0.0744292845724269,0.0776622687654903,
0.0817097633423073,0.0826589280377865),.UNSPECIFIED.);
#24304=B_SPLINE_CURVE_WITH_KNOTS('',3,(#151881,#151882,#151883,#151884,
#151885,#151886),.UNSPECIFIED.,.F.,.F.,(4,2,4),(1.49996604605924,1.51351365751903,
1.57686258982277),.UNSPECIFIED.);
#24305=B_SPLINE_CURVE_WITH_KNOTS('',3,(#151888,#151889,#151890,#151891,
#151892,#151893),.UNSPECIFIED.,.F.,.F.,(4,2,4),(1.33957856731205,1.4029274995552,
1.41647511105415),.UNSPECIFIED.);
#24306=B_SPLINE_CURVE_WITH_KNOTS('',3,(#151895,#151896,#151897,#151898,
#151899,#151900,#151901,#151902,#151903,#151904,#151905,#151906,#151907,
#151908,#151909,#151910,#151911,#151912,#151913),.UNSPECIFIED.,.F.,.F.,
(4,2,2,2,3,2,2,2,4),(0.0600992581771638,0.0615656152950589,0.0659612937616956,
0.0687970446672038,0.0714824588521353,0.0744292845694206,0.0776622687623728,
0.0817097633385307,0.0826589280870864),.UNSPECIFIED.);
#24307=B_SPLINE_CURVE_WITH_KNOTS('',3,(#151914,#151915,#151916,#151917,
#151918,#151919),.UNSPECIFIED.,.F.,.F.,(4,2,4),(1.49996604610752,1.51351365759858,
1.57686258989254),.UNSPECIFIED.);
#24308=B_SPLINE_CURVE_WITH_KNOTS('',3,(#151921,#151922,#151923,#151924,
#151925,#151926),.UNSPECIFIED.,.F.,.F.,(4,2,4),(1.33957856760233,1.4029274999419,
1.41647511136569),.UNSPECIFIED.);
#24309=B_SPLINE_CURVE_WITH_KNOTS('',3,(#151928,#151929,#151930,#151931,
#151932,#151933,#151934,#151935,#151936,#151937,#151938,#151939,#151940,
#151941,#151942,#151943,#151944,#151945,#151946),.UNSPECIFIED.,.F.,.F.,
(4,2,2,2,3,2,2,2,4),(0.0600992582006101,0.0615656152993682,0.0659612937620992,
0.068797044666235,0.0714824588501786,0.0744292845673599,0.0776622687618674,
0.0817097633414001,0.0826589280678798),.UNSPECIFIED.);
#24310=B_SPLINE_CURVE_WITH_KNOTS('',3,(#151947,#151948,#151949,#151950,
#151951,#151952),.UNSPECIFIED.,.F.,.F.,(4,2,4),(1.49996604589165,1.51351365742799,
1.57686258964856),.UNSPECIFIED.);
#24311=B_SPLINE_CURVE_WITH_KNOTS('',3,(#151954,#151955,#151956,#151957,
#151958,#151959),.UNSPECIFIED.,.F.,.F.,(4,2,4),(1.33957856743351,1.40292749973926,
1.41647511120219),.UNSPECIFIED.);
#24312=B_SPLINE_CURVE_WITH_KNOTS('',3,(#151961,#151962,#151963,#151964,
#151965,#151966,#151967,#151968,#151969,#151970,#151971,#151972,#151973,
#151974,#151975,#151976,#151977,#151978,#151979),.UNSPECIFIED.,.F.,.F.,
(4,2,2,2,3,2,2,2,4),(0.060099258224775,0.0615656153025146,0.0659612937676359,
0.0687970446730238,0.0714824588578852,0.0744292845745959,0.0776622687680001,
0.0817097633459842,0.0826589280412753),.UNSPECIFIED.);
#24313=B_SPLINE_CURVE_WITH_KNOTS('',3,(#151980,#151981,#151982,#151983,
#151984,#151985),.UNSPECIFIED.,.F.,.F.,(4,2,4),(1.49996604599409,1.51351365749675,
1.57686258976619),.UNSPECIFIED.);
#24314=B_SPLINE_CURVE_WITH_KNOTS('',3,(#151987,#151988,#151989,#151990,
#151991,#151992),.UNSPECIFIED.,.F.,.F.,(4,2,4),(1.33957856743393,1.40292749973875,
1.41647511122195),.UNSPECIFIED.);
#24315=B_SPLINE_CURVE_WITH_KNOTS('',3,(#151994,#151995,#151996,#151997,
#151998,#151999,#152000,#152001,#152002,#152003,#152004,#152005,#152006,
#152007,#152008,#152009,#152010,#152011,#152012),.UNSPECIFIED.,.F.,.F.,
(4,2,2,2,3,2,2,2,4),(0.0600992582585029,0.0615656153046349,0.0659612937700477,
0.0687970446757806,0.0714824588609026,0.0744292845773481,0.0776622687705401,
0.0817097633484953,0.0826589280092112),.UNSPECIFIED.);
#24316=B_SPLINE_CURVE_WITH_KNOTS('',3,(#152013,#152014,#152015,#152016,
#152017,#152018),.UNSPECIFIED.,.F.,.F.,(4,2,4),(1.49996604599272,1.51351365750805,
1.5768625897927),.UNSPECIFIED.);
#24317=B_SPLINE_CURVE_WITH_KNOTS('',3,(#152020,#152021,#152022,#152023,
#152024,#152025),.UNSPECIFIED.,.F.,.F.,(4,2,4),(1.33957856741527,1.40292749969865,
1.41647511118214),.UNSPECIFIED.);
#24318=B_SPLINE_CURVE_WITH_KNOTS('',3,(#152026,#152027,#152028,#152029,
#152030,#152031,#152032,#152033,#152034,#152035),.UNSPECIFIED.,.F.,.F.,
(4,2,2,2,4),(0.0600992582453176,0.0615656153017531,0.0659612937676228,0.0687970446733949,
0.0714824588585375),.UNSPECIFIED.);
#28290=LINE('',#147769,#32092);
#28291=LINE('',#147777,#32093);
#28292=LINE('',#147785,#32094);
#28293=LINE('',#147793,#32095);
#28294=LINE('',#147800,#32096);
#28295=LINE('',#147806,#32097);
#28296=LINE('',#147813,#32098);
#28297=LINE('',#147820,#32099);
#28298=LINE('',#147823,#32100);
#28299=LINE('',#147825,#32101);
#28300=LINE('',#148785,#32102);
#28301=LINE('',#149724,#32103);
#28302=LINE('',#152038,#32104);
#28303=LINE('',#152041,#32105);
#28304=LINE('',#152399,#32106);
#28305=LINE('',#152405,#32107);
#28306=LINE('',#152488,#32108);
#28307=LINE('',#152491,#32109);
#28308=LINE('',#152497,#32110);
#28309=LINE('',#152500,#32111);
#28310=LINE('',#152504,#32112);
#28311=LINE('',#152506,#32113);
#28312=LINE('',#152508,#32114);
#28313=LINE('',#152512,#32115);
#28314=LINE('',#152518,#32116);
#28315=LINE('',#152521,#32117);
#28316=LINE('',#152527,#32118);
#28317=LINE('',#152530,#32119);
#28318=LINE('',#152536,#32120);
#28319=LINE('',#152539,#32121);
#28320=LINE('',#152545,#32122);
#28321=LINE('',#152548,#32123);
#28322=LINE('',#152550,#32124);
#28323=LINE('',#152841,#32125);
#28324=LINE('',#152847,#32126);
#28325=LINE('',#152851,#32127);
#28326=LINE('',#152856,#32128);
#28327=LINE('',#152864,#32129);
#28328=LINE('',#152866,#32130);
#28329=LINE('',#152870,#32131);
#28330=LINE('',#152873,#32132);
#28331=LINE('',#152876,#32133);
#28332=LINE('',#152878,#32134);
#28333=LINE('',#152882,#32135);
#28334=LINE('',#152884,#32136);
#28335=LINE('',#152888,#32137);
#28336=LINE('',#152890,#32138);
#28337=LINE('',#152894,#32139);
#28338=LINE('',#152898,#32140);
#28339=LINE('',#152902,#32141);
#28340=LINE('',#152905,#32142);
#28341=LINE('',#152908,#32143);
#28342=LINE('',#152910,#32144);
#28343=LINE('',#152914,#32145);
#28344=LINE('',#152916,#32146);
#28345=LINE('',#152920,#32147);
#28346=LINE('',#152923,#32148);
#28347=LINE('',#152926,#32149);
#28348=LINE('',#152928,#32150);
#28349=LINE('',#152933,#32151);
#28350=LINE('',#152937,#32152);
#28351=LINE('',#152940,#32153);
#28352=LINE('',#152943,#32154);
#28353=LINE('',#152946,#32155);
#28354=LINE('',#152948,#32156);
#28355=LINE('',#152952,#32157);
#28356=LINE('',#152955,#32158);
#28357=LINE('',#152958,#32159);
#28358=LINE('',#152960,#32160);
#28359=LINE('',#152964,#32161);
#28360=LINE('',#152966,#32162);
#28361=LINE('',#152970,#32163);
#28362=LINE('',#152973,#32164);
#28363=LINE('',#152976,#32165);
#28364=LINE('',#152978,#32166);
#28365=LINE('',#152982,#32167);
#28366=LINE('',#152985,#32168);
#28367=LINE('',#152988,#32169);
#28368=LINE('',#152991,#32170);
#28369=LINE('',#152994,#32171);
#28370=LINE('',#152997,#32172);
#28371=LINE('',#153000,#32173);
#28372=LINE('',#153002,#32174);
#28373=LINE('',#153006,#32175);
#28374=LINE('',#153009,#32176);
#28375=LINE('',#153012,#32177);
#28376=LINE('',#153014,#32178);
#28377=LINE('',#153018,#32179);
#28378=LINE('',#153020,#32180);
#28379=LINE('',#153024,#32181);
#28380=LINE('',#153027,#32182);
#28381=LINE('',#153030,#32183);
#28382=LINE('',#153032,#32184);
#28383=LINE('',#153036,#32185);
#28384=LINE('',#153039,#32186);
#28385=LINE('',#153042,#32187);
#28386=LINE('',#153045,#32188);
#28387=LINE('',#153048,#32189);
#28388=LINE('',#153051,#32190);
#28389=LINE('',#153054,#32191);
#28390=LINE('',#153056,#32192);
#28391=LINE('',#153060,#32193);
#28392=LINE('',#153062,#32194);
#28393=LINE('',#153066,#32195);
#28394=LINE('',#153068,#32196);
#28395=LINE('',#153252,#32197);
#28396=LINE('',#153253,#32198);
#28397=LINE('',#153255,#32199);
#28398=LINE('',#153257,#32200);
#28399=LINE('',#153260,#32201);
#28400=LINE('',#153262,#32202);
#28401=LINE('',#153265,#32203);
#28402=LINE('',#153267,#32204);
#28403=LINE('',#153270,#32205);
#28404=LINE('',#153272,#32206);
#28405=LINE('',#153275,#32207);
#28406=LINE('',#153277,#32208);
#28407=LINE('',#153280,#32209);
#28408=LINE('',#153282,#32210);
#28409=LINE('',#153285,#32211);
#28410=LINE('',#153287,#32212);
#28411=LINE('',#153290,#32213);
#28412=LINE('',#153292,#32214);
#28413=LINE('',#153295,#32215);
#28414=LINE('',#153297,#32216);
#28415=LINE('',#153300,#32217);
#28416=LINE('',#153302,#32218);
#28417=LINE('',#153305,#32219);
#28418=LINE('',#153307,#32220);
#28419=LINE('',#153310,#32221);
#28420=LINE('',#153312,#32222);
#28421=LINE('',#153315,#32223);
#28422=LINE('',#153317,#32224);
#28423=LINE('',#153320,#32225);
#28424=LINE('',#153322,#32226);
#28425=LINE('',#153325,#32227);
#28426=LINE('',#153327,#32228);
#28427=LINE('',#153330,#32229);
#28428=LINE('',#153332,#32230);
#28429=LINE('',#153335,#32231);
#28430=LINE('',#153337,#32232);
#28431=LINE('',#153340,#32233);
#28432=LINE('',#153342,#32234);
#28433=LINE('',#153345,#32235);
#28434=LINE('',#153347,#32236);
#28435=LINE('',#153350,#32237);
#28436=LINE('',#153352,#32238);
#28437=LINE('',#153355,#32239);
#28438=LINE('',#153357,#32240);
#28439=LINE('',#153360,#32241);
#28440=LINE('',#153362,#32242);
#28441=LINE('',#153365,#32243);
#28442=LINE('',#153367,#32244);
#28443=LINE('',#153370,#32245);
#28444=LINE('',#153372,#32246);
#28445=LINE('',#153375,#32247);
#28446=LINE('',#153377,#32248);
#28447=LINE('',#153380,#32249);
#28448=LINE('',#153383,#32250);
#28449=LINE('',#153386,#32251);
#28450=LINE('',#153388,#32252);
#28451=LINE('',#153391,#32253);
#28452=LINE('',#153393,#32254);
#28453=LINE('',#153396,#32255);
#28454=LINE('',#153398,#32256);
#28455=LINE('',#153401,#32257);
#28456=LINE('',#153403,#32258);
#28457=LINE('',#153406,#32259);
#28458=LINE('',#153409,#32260);
#28459=LINE('',#153412,#32261);
#28460=LINE('',#153414,#32262);
#28461=LINE('',#153417,#32263);
#28462=LINE('',#153419,#32264);
#28463=LINE('',#153422,#32265);
#28464=LINE('',#153424,#32266);
#28465=LINE('',#153427,#32267);
#28466=LINE('',#153429,#32268);
#28467=LINE('',#153438,#32269);
#28468=LINE('',#153439,#32270);
#28469=LINE('',#153440,#32271);
#28470=LINE('',#153444,#32272);
#28471=LINE('',#153450,#32273);
#28472=LINE('',#153456,#32274);
#28473=LINE('',#153461,#32275);
#28474=LINE('',#153462,#32276);
#28475=LINE('',#153463,#32277);
#28476=LINE('',#153466,#32278);
#28477=LINE('',#153475,#32279);
#28478=LINE('',#153479,#32280);
#28479=LINE('',#153482,#32281);
#28480=LINE('',#153483,#32282);
#28481=LINE('',#153486,#32283);
#28482=LINE('',#153491,#32284);
#28483=LINE('',#153496,#32285);
#28484=LINE('',#153497,#32286);
#28485=LINE('',#153498,#32287);
#28486=LINE('',#153502,#32288);
#32092=VECTOR('',#111922,2.9);
#32093=VECTOR('',#111931,1.5);
#32094=VECTOR('',#111940,1.5);
#32095=VECTOR('',#111949,8.8);
#32096=VECTOR('',#111958,1.7);
#32097=VECTOR('',#111965,1.7);
#32098=VECTOR('',#111972,3.3);
#32099=VECTOR('',#111981,2.5);
#32100=VECTOR('',#111986,1.5);
#32101=VECTOR('',#111989,1.5);
#32102=VECTOR('',#111992,9.);
#32103=VECTOR('',#111997,9.);
#32104=VECTOR('',#112000,3.5);
#32105=VECTOR('',#112005,2.5);
#32106=VECTOR('',#112716,1.);
#32107=VECTOR('',#112723,1.);
#32108=VECTOR('',#112824,2.3);
#32109=VECTOR('',#112827,2.3);
#32110=VECTOR('',#112832,2.3);
#32111=VECTOR('',#112835,2.299999999);
#32112=VECTOR('',#112840,3.5);
#32113=VECTOR('',#112843,1.5);
#32114=VECTOR('',#112846,1.5);
#32115=VECTOR('',#112851,3.);
#32116=VECTOR('',#112856,5.);
#32117=VECTOR('',#112859,5.);
#32118=VECTOR('',#112864,5.);
#32119=VECTOR('',#112867,5.);
#32120=VECTOR('',#112872,5.);
#32121=VECTOR('',#112875,5.);
#32122=VECTOR('',#112880,5.);
#32123=VECTOR('',#112883,5.);
#32124=VECTOR('',#112886,1.5);
#32125=VECTOR('',#113181,1.40306029339696);
#32126=VECTOR('',#113186,1.40306029339696);
#32127=VECTOR('',#113189,1.40306029339696);
#32128=VECTOR('',#113194,1.40306029339696);
#32129=VECTOR('',#113203,5.);
#32130=VECTOR('',#113204,5.);
#32131=VECTOR('',#113209,5.);
#32132=VECTOR('',#113212,5.);
#32133=VECTOR('',#113215,5.);
#32134=VECTOR('',#113216,5.);
#32135=VECTOR('',#113221,5.);
#32136=VECTOR('',#113222,5.);
#32137=VECTOR('',#113227,5.);
#32138=VECTOR('',#113228,5.);
#32139=VECTOR('',#113233,5.);
#32140=VECTOR('',#113238,5.);
#32141=VECTOR('',#113243,5.);
#32142=VECTOR('',#113246,5.);
#32143=VECTOR('',#113249,5.);
#32144=VECTOR('',#113250,5.);
#32145=VECTOR('',#113255,5.);
#32146=VECTOR('',#113256,5.);
#32147=VECTOR('',#113261,5.);
#32148=VECTOR('',#113264,5.);
#32149=VECTOR('',#113267,5.);
#32150=VECTOR('',#113268,5.);
#32151=VECTOR('',#113275,5.);
#32152=VECTOR('',#113280,5.);
#32153=VECTOR('',#113283,5.);
#32154=VECTOR('',#113286,5.);
#32155=VECTOR('',#113289,5.);
#32156=VECTOR('',#113290,5.);
#32157=VECTOR('',#113295,5.);
#32158=VECTOR('',#113298,5.);
#32159=VECTOR('',#113301,5.);
#32160=VECTOR('',#113302,5.);
#32161=VECTOR('',#113307,5.);
#32162=VECTOR('',#113308,5.);
#32163=VECTOR('',#113313,5.);
#32164=VECTOR('',#113316,5.);
#32165=VECTOR('',#113319,5.);
#32166=VECTOR('',#113320,5.);
#32167=VECTOR('',#113325,5.);
#32168=VECTOR('',#113328,5.);
#32169=VECTOR('',#113331,5.);
#32170=VECTOR('',#113334,5.);
#32171=VECTOR('',#113337,5.);
#32172=VECTOR('',#113340,5.);
#32173=VECTOR('',#113343,5.);
#32174=VECTOR('',#113344,5.);
#32175=VECTOR('',#113349,5.);
#32176=VECTOR('',#113352,5.);
#32177=VECTOR('',#113355,5.);
#32178=VECTOR('',#113356,5.);
#32179=VECTOR('',#113361,5.);
#32180=VECTOR('',#113362,5.);
#32181=VECTOR('',#113367,5.);
#32182=VECTOR('',#113370,5.);
#32183=VECTOR('',#113373,5.);
#32184=VECTOR('',#113374,5.);
#32185=VECTOR('',#113379,5.);
#32186=VECTOR('',#113382,5.);
#32187=VECTOR('',#113385,5.);
#32188=VECTOR('',#113388,5.);
#32189=VECTOR('',#113391,5.);
#32190=VECTOR('',#113394,5.);
#32191=VECTOR('',#113397,5.);
#32192=VECTOR('',#113398,5.);
#32193=VECTOR('',#113403,5.);
#32194=VECTOR('',#113404,5.);
#32195=VECTOR('',#113409,5.);
#32196=VECTOR('',#113410,5.);
#32197=VECTOR('',#113633,5.);
#32198=VECTOR('',#113634,5.);
#32199=VECTOR('',#113637,5.);
#32200=VECTOR('',#113640,5.);
#32201=VECTOR('',#113645,5.);
#32202=VECTOR('',#113648,5.);
#32203=VECTOR('',#113653,5.);
#32204=VECTOR('',#113656,5.);
#32205=VECTOR('',#113661,5.);
#32206=VECTOR('',#113664,5.);
#32207=VECTOR('',#113669,5.);
#32208=VECTOR('',#113672,5.);
#32209=VECTOR('',#113677,5.);
#32210=VECTOR('',#113680,5.);
#32211=VECTOR('',#113685,5.);
#32212=VECTOR('',#113688,5.);
#32213=VECTOR('',#113693,5.);
#32214=VECTOR('',#113696,5.);
#32215=VECTOR('',#113701,5.);
#32216=VECTOR('',#113704,5.);
#32217=VECTOR('',#113709,5.);
#32218=VECTOR('',#113712,5.);
#32219=VECTOR('',#113717,5.);
#32220=VECTOR('',#113720,5.);
#32221=VECTOR('',#113725,5.);
#32222=VECTOR('',#113728,5.);
#32223=VECTOR('',#113733,5.);
#32224=VECTOR('',#113736,5.);
#32225=VECTOR('',#113741,5.);
#32226=VECTOR('',#113744,5.);
#32227=VECTOR('',#113749,5.);
#32228=VECTOR('',#113752,5.);
#32229=VECTOR('',#113757,5.);
#32230=VECTOR('',#113760,5.);
#32231=VECTOR('',#113765,5.);
#32232=VECTOR('',#113768,5.);
#32233=VECTOR('',#113773,5.);
#32234=VECTOR('',#113776,5.);
#32235=VECTOR('',#113781,5.);
#32236=VECTOR('',#113784,5.);
#32237=VECTOR('',#113789,5.);
#32238=VECTOR('',#113792,5.);
#32239=VECTOR('',#113797,5.);
#32240=VECTOR('',#113800,5.);
#32241=VECTOR('',#113805,5.);
#32242=VECTOR('',#113808,5.);
#32243=VECTOR('',#113813,5.);
#32244=VECTOR('',#113816,5.);
#32245=VECTOR('',#113821,5.);
#32246=VECTOR('',#113824,5.);
#32247=VECTOR('',#113829,5.);
#32248=VECTOR('',#113832,5.);
#32249=VECTOR('',#113837,5.);
#32250=VECTOR('',#113842,5.);
#32251=VECTOR('',#113847,5.);
#32252=VECTOR('',#113850,5.);
#32253=VECTOR('',#113855,5.);
#32254=VECTOR('',#113858,5.);
#32255=VECTOR('',#113863,5.);
#32256=VECTOR('',#113866,5.);
#32257=VECTOR('',#113871,5.);
#32258=VECTOR('',#113874,5.);
#32259=VECTOR('',#113879,5.);
#32260=VECTOR('',#113884,5.);
#32261=VECTOR('',#113889,5.);
#32262=VECTOR('',#113892,5.);
#32263=VECTOR('',#113897,5.);
#32264=VECTOR('',#113900,5.);
#32265=VECTOR('',#113905,5.);
#32266=VECTOR('',#113908,5.);
#32267=VECTOR('',#113913,5.);
#32268=VECTOR('',#113916,5.);
#32269=VECTOR('',#113929,2.3);
#32270=VECTOR('',#113930,1.40306029239696);
#32271=VECTOR('',#113931,1.40306029239696);
#32272=VECTOR('',#113934,2.3);
#32273=VECTOR('',#113941,2.3);
#32274=VECTOR('',#113948,2.3);
#32275=VECTOR('',#113955,2.3);
#32276=VECTOR('',#113956,1.40306029239696);
#32277=VECTOR('',#113957,1.40306029239696);
#32278=VECTOR('',#113960,2.3);
#32279=VECTOR('',#113973,2.3);
#32280=VECTOR('',#113976,2.3);
#32281=VECTOR('',#113981,1.40306029339696);
#32282=VECTOR('',#113982,1.40306029239696);
#32283=VECTOR('',#113985,2.3);
#32284=VECTOR('',#113992,2.3);
#32285=VECTOR('',#113997,2.3);
#32286=VECTOR('',#113998,1.40306029339696);
#32287=VECTOR('',#113999,1.40306029239696);
#32288=VECTOR('',#114002,2.3);
#36496=VERTEX_POINT('',#145875);
#36497=VERTEX_POINT('',#145876);
#36498=VERTEX_POINT('',#145887);
#36499=VERTEX_POINT('',#145889);
#36500=VERTEX_POINT('',#145902);
#36501=VERTEX_POINT('',#145903);
#36502=VERTEX_POINT('',#145914);
#36503=VERTEX_POINT('',#145916);
#36504=VERTEX_POINT('',#145929);
#36505=VERTEX_POINT('',#145930);
#36506=VERTEX_POINT('',#145941);
#36507=VERTEX_POINT('',#145943);
#36508=VERTEX_POINT('',#145956);
#36509=VERTEX_POINT('',#145957);
#36510=VERTEX_POINT('',#145968);
#36511=VERTEX_POINT('',#145970);
#36512=VERTEX_POINT('',#145983);
#36513=VERTEX_POINT('',#145984);
#36514=VERTEX_POINT('',#145995);
#36515=VERTEX_POINT('',#145997);
#36516=VERTEX_POINT('',#146010);
#36517=VERTEX_POINT('',#146011);
#36518=VERTEX_POINT('',#146022);
#36519=VERTEX_POINT('',#146024);
#36520=VERTEX_POINT('',#146037);
#36521=VERTEX_POINT('',#146038);
#36522=VERTEX_POINT('',#146049);
#36523=VERTEX_POINT('',#146051);
#36524=VERTEX_POINT('',#146064);
#36525=VERTEX_POINT('',#146065);
#36526=VERTEX_POINT('',#146076);
#36527=VERTEX_POINT('',#146078);
#36528=VERTEX_POINT('',#146091);
#36529=VERTEX_POINT('',#146092);
#36530=VERTEX_POINT('',#146103);
#36531=VERTEX_POINT('',#146105);
#36532=VERTEX_POINT('',#146118);
#36533=VERTEX_POINT('',#146119);
#36534=VERTEX_POINT('',#146130);
#36535=VERTEX_POINT('',#146132);
#36536=VERTEX_POINT('',#146145);
#36537=VERTEX_POINT('',#146146);
#36538=VERTEX_POINT('',#146157);
#36539=VERTEX_POINT('',#146159);
#36540=VERTEX_POINT('',#146172);
#36541=VERTEX_POINT('',#146173);
#36542=VERTEX_POINT('',#146184);
#36543=VERTEX_POINT('',#146186);
#36544=VERTEX_POINT('',#146199);
#36545=VERTEX_POINT('',#146200);
#36546=VERTEX_POINT('',#146211);
#36547=VERTEX_POINT('',#146213);
#36548=VERTEX_POINT('',#146226);
#36549=VERTEX_POINT('',#146227);
#36550=VERTEX_POINT('',#146238);
#36551=VERTEX_POINT('',#146240);
#36552=VERTEX_POINT('',#146253);
#36553=VERTEX_POINT('',#146254);
#36554=VERTEX_POINT('',#146265);
#36555=VERTEX_POINT('',#146267);
#36556=VERTEX_POINT('',#146280);
#36557=VERTEX_POINT('',#146281);
#36558=VERTEX_POINT('',#146292);
#36559=VERTEX_POINT('',#146294);
#36560=VERTEX_POINT('',#146307);
#36561=VERTEX_POINT('',#146308);
#36562=VERTEX_POINT('',#146319);
#36563=VERTEX_POINT('',#146321);
#36564=VERTEX_POINT('',#146334);
#36565=VERTEX_POINT('',#146335);
#36566=VERTEX_POINT('',#146346);
#36567=VERTEX_POINT('',#146348);
#36568=VERTEX_POINT('',#146361);
#36569=VERTEX_POINT('',#146362);
#36570=VERTEX_POINT('',#146373);
#36571=VERTEX_POINT('',#146375);
#36572=VERTEX_POINT('',#146388);
#36573=VERTEX_POINT('',#146389);
#36574=VERTEX_POINT('',#146400);
#36575=VERTEX_POINT('',#146402);
#36576=VERTEX_POINT('',#146415);
#36577=VERTEX_POINT('',#146416);
#36578=VERTEX_POINT('',#146427);
#36579=VERTEX_POINT('',#146429);
#36580=VERTEX_POINT('',#146442);
#36581=VERTEX_POINT('',#146443);
#36582=VERTEX_POINT('',#146454);
#36583=VERTEX_POINT('',#146456);
#36584=VERTEX_POINT('',#146469);
#36585=VERTEX_POINT('',#146470);
#36586=VERTEX_POINT('',#146481);
#36587=VERTEX_POINT('',#146483);
#36588=VERTEX_POINT('',#146496);
#36589=VERTEX_POINT('',#146497);
#36590=VERTEX_POINT('',#146508);
#36591=VERTEX_POINT('',#146510);
#36592=VERTEX_POINT('',#146523);
#36593=VERTEX_POINT('',#146524);
#36594=VERTEX_POINT('',#146535);
#36595=VERTEX_POINT('',#146537);
#36596=VERTEX_POINT('',#146550);
#36597=VERTEX_POINT('',#146551);
#36598=VERTEX_POINT('',#146562);
#36599=VERTEX_POINT('',#146564);
#36600=VERTEX_POINT('',#146577);
#36601=VERTEX_POINT('',#146578);
#36602=VERTEX_POINT('',#146589);
#36603=VERTEX_POINT('',#146591);
#36604=VERTEX_POINT('',#146604);
#36605=VERTEX_POINT('',#146605);
#36606=VERTEX_POINT('',#146616);
#36607=VERTEX_POINT('',#146618);
#36608=VERTEX_POINT('',#146631);
#36609=VERTEX_POINT('',#146632);
#36610=VERTEX_POINT('',#146643);
#36611=VERTEX_POINT('',#146645);
#36612=VERTEX_POINT('',#146658);
#36613=VERTEX_POINT('',#146659);
#36614=VERTEX_POINT('',#146670);
#36615=VERTEX_POINT('',#146672);
#36616=VERTEX_POINT('',#146685);
#36617=VERTEX_POINT('',#146686);
#36618=VERTEX_POINT('',#146697);
#36619=VERTEX_POINT('',#146699);
#36620=VERTEX_POINT('',#146712);
#36621=VERTEX_POINT('',#146713);
#36622=VERTEX_POINT('',#146724);
#36623=VERTEX_POINT('',#146726);
#36624=VERTEX_POINT('',#146739);
#36625=VERTEX_POINT('',#146740);
#36626=VERTEX_POINT('',#146751);
#36627=VERTEX_POINT('',#146753);
#36628=VERTEX_POINT('',#146766);
#36629=VERTEX_POINT('',#146767);
#36630=VERTEX_POINT('',#146778);
#36631=VERTEX_POINT('',#146780);
#36632=VERTEX_POINT('',#146793);
#36633=VERTEX_POINT('',#146794);
#36634=VERTEX_POINT('',#146805);
#36635=VERTEX_POINT('',#146807);
#36636=VERTEX_POINT('',#146820);
#36637=VERTEX_POINT('',#146821);
#36638=VERTEX_POINT('',#146832);
#36639=VERTEX_POINT('',#146834);
#36640=VERTEX_POINT('',#146847);
#36641=VERTEX_POINT('',#146848);
#36642=VERTEX_POINT('',#146859);
#36643=VERTEX_POINT('',#146861);
#36644=VERTEX_POINT('',#146874);
#36645=VERTEX_POINT('',#146875);
#36646=VERTEX_POINT('',#146886);
#36647=VERTEX_POINT('',#146888);
#36648=VERTEX_POINT('',#146901);
#36649=VERTEX_POINT('',#146902);
#36650=VERTEX_POINT('',#146913);
#36651=VERTEX_POINT('',#146915);
#36652=VERTEX_POINT('',#146928);
#36653=VERTEX_POINT('',#146929);
#36654=VERTEX_POINT('',#146940);
#36655=VERTEX_POINT('',#146942);
#36656=VERTEX_POINT('',#146955);
#36657=VERTEX_POINT('',#146956);
#36658=VERTEX_POINT('',#146967);
#36659=VERTEX_POINT('',#146969);
#36660=VERTEX_POINT('',#146982);
#36661=VERTEX_POINT('',#146983);
#36662=VERTEX_POINT('',#146994);
#36663=VERTEX_POINT('',#146996);
#36664=VERTEX_POINT('',#147009);
#36665=VERTEX_POINT('',#147010);
#36666=VERTEX_POINT('',#147021);
#36667=VERTEX_POINT('',#147023);
#36668=VERTEX_POINT('',#147036);
#36669=VERTEX_POINT('',#147037);
#36670=VERTEX_POINT('',#147048);
#36671=VERTEX_POINT('',#147050);
#36672=VERTEX_POINT('',#147063);
#36673=VERTEX_POINT('',#147064);
#36674=VERTEX_POINT('',#147075);
#36675=VERTEX_POINT('',#147077);
#36676=VERTEX_POINT('',#147090);
#36677=VERTEX_POINT('',#147091);
#36678=VERTEX_POINT('',#147102);
#36679=VERTEX_POINT('',#147104);
#36680=VERTEX_POINT('',#147117);
#36681=VERTEX_POINT('',#147118);
#36682=VERTEX_POINT('',#147129);
#36683=VERTEX_POINT('',#147131);
#36684=VERTEX_POINT('',#147144);
#36685=VERTEX_POINT('',#147145);
#36686=VERTEX_POINT('',#147156);
#36687=VERTEX_POINT('',#147158);
#36688=VERTEX_POINT('',#147171);
#36689=VERTEX_POINT('',#147172);
#36690=VERTEX_POINT('',#147183);
#36691=VERTEX_POINT('',#147185);
#36692=VERTEX_POINT('',#147198);
#36693=VERTEX_POINT('',#147199);
#36694=VERTEX_POINT('',#147210);
#36695=VERTEX_POINT('',#147212);
#36696=VERTEX_POINT('',#147225);
#36697=VERTEX_POINT('',#147226);
#36698=VERTEX_POINT('',#147237);
#36699=VERTEX_POINT('',#147239);
#36700=VERTEX_POINT('',#147252);
#36701=VERTEX_POINT('',#147253);
#36702=VERTEX_POINT('',#147264);
#36703=VERTEX_POINT('',#147266);
#36704=VERTEX_POINT('',#147279);
#36705=VERTEX_POINT('',#147280);
#36706=VERTEX_POINT('',#147291);
#36707=VERTEX_POINT('',#147293);
#36708=VERTEX_POINT('',#147306);
#36709=VERTEX_POINT('',#147307);
#36710=VERTEX_POINT('',#147318);
#36711=VERTEX_POINT('',#147320);
#36712=VERTEX_POINT('',#147333);
#36713=VERTEX_POINT('',#147334);
#36714=VERTEX_POINT('',#147345);
#36715=VERTEX_POINT('',#147347);
#36716=VERTEX_POINT('',#147360);
#36717=VERTEX_POINT('',#147361);
#36718=VERTEX_POINT('',#147372);
#36719=VERTEX_POINT('',#147374);
#36720=VERTEX_POINT('',#147387);
#36721=VERTEX_POINT('',#147388);
#36722=VERTEX_POINT('',#147399);
#36723=VERTEX_POINT('',#147401);
#36724=VERTEX_POINT('',#147414);
#36725=VERTEX_POINT('',#147415);
#36726=VERTEX_POINT('',#147426);
#36727=VERTEX_POINT('',#147428);
#36728=VERTEX_POINT('',#147441);
#36729=VERTEX_POINT('',#147442);
#36730=VERTEX_POINT('',#147453);
#36731=VERTEX_POINT('',#147455);
#36732=VERTEX_POINT('',#147468);
#36733=VERTEX_POINT('',#147469);
#36734=VERTEX_POINT('',#147480);
#36735=VERTEX_POINT('',#147482);
#36736=VERTEX_POINT('',#147495);
#36737=VERTEX_POINT('',#147496);
#36738=VERTEX_POINT('',#147507);
#36739=VERTEX_POINT('',#147509);
#36740=VERTEX_POINT('',#147522);
#36741=VERTEX_POINT('',#147523);
#36742=VERTEX_POINT('',#147534);
#36743=VERTEX_POINT('',#147536);
#36744=VERTEX_POINT('',#147549);
#36745=VERTEX_POINT('',#147550);
#36746=VERTEX_POINT('',#147561);
#36747=VERTEX_POINT('',#147563);
#36748=VERTEX_POINT('',#147576);
#36749=VERTEX_POINT('',#147577);
#36750=VERTEX_POINT('',#147588);
#36751=VERTEX_POINT('',#147590);
#36752=VERTEX_POINT('',#147603);
#36753=VERTEX_POINT('',#147604);
#36754=VERTEX_POINT('',#147615);
#36755=VERTEX_POINT('',#147617);
#36756=VERTEX_POINT('',#147630);
#36757=VERTEX_POINT('',#147631);
#36758=VERTEX_POINT('',#147642);
#36759=VERTEX_POINT('',#147644);
#36760=VERTEX_POINT('',#147657);
#36761=VERTEX_POINT('',#147658);
#36762=VERTEX_POINT('',#147669);
#36763=VERTEX_POINT('',#147671);
#36764=VERTEX_POINT('',#147684);
#36765=VERTEX_POINT('',#147685);
#36766=VERTEX_POINT('',#147696);
#36767=VERTEX_POINT('',#147698);
#36768=VERTEX_POINT('',#147711);
#36769=VERTEX_POINT('',#147712);
#36770=VERTEX_POINT('',#147723);
#36771=VERTEX_POINT('',#147725);
#36772=VERTEX_POINT('',#147738);
#36773=VERTEX_POINT('',#147739);
#36774=VERTEX_POINT('',#147750);
#36775=VERTEX_POINT('',#147752);
#36776=VERTEX_POINT('',#147765);
#36777=VERTEX_POINT('',#147766);
#36778=VERTEX_POINT('',#147768);
#36779=VERTEX_POINT('',#147773);
#36780=VERTEX_POINT('',#147774);
#36781=VERTEX_POINT('',#147776);
#36782=VERTEX_POINT('',#147781);
#36783=VERTEX_POINT('',#147782);
#36784=VERTEX_POINT('',#147784);
#36785=VERTEX_POINT('',#147789);
#36786=VERTEX_POINT('',#147790);
#36787=VERTEX_POINT('',#147792);
#36788=VERTEX_POINT('',#147797);
#36789=VERTEX_POINT('',#147799);
#36790=VERTEX_POINT('',#147803);
#36791=VERTEX_POINT('',#147805);
#36792=VERTEX_POINT('',#147809);
#36793=VERTEX_POINT('',#147810);
#36794=VERTEX_POINT('',#147812);
#36795=VERTEX_POINT('',#147817);
#36796=VERTEX_POINT('',#147819);
#36797=VERTEX_POINT('',#147827);
#36798=VERTEX_POINT('',#147828);
#36799=VERTEX_POINT('',#147850);
#36800=VERTEX_POINT('',#147855);
#36801=VERTEX_POINT('',#147877);
#36802=VERTEX_POINT('',#147882);
#36803=VERTEX_POINT('',#147904);
#36804=VERTEX_POINT('',#147909);
#36805=VERTEX_POINT('',#147931);
#36806=VERTEX_POINT('',#147936);
#36807=VERTEX_POINT('',#147958);
#36808=VERTEX_POINT('',#147963);
#36809=VERTEX_POINT('',#147985);
#36810=VERTEX_POINT('',#147990);
#36811=VERTEX_POINT('',#148012);
#36812=VERTEX_POINT('',#148017);
#36813=VERTEX_POINT('',#148039);
#36814=VERTEX_POINT('',#148044);
#36815=VERTEX_POINT('',#148066);
#36816=VERTEX_POINT('',#148071);
#36817=VERTEX_POINT('',#148093);
#36818=VERTEX_POINT('',#148098);
#36819=VERTEX_POINT('',#148120);
#36820=VERTEX_POINT('',#148125);
#36821=VERTEX_POINT('',#148147);
#36822=VERTEX_POINT('',#148152);
#36823=VERTEX_POINT('',#148174);
#36824=VERTEX_POINT('',#148179);
#36825=VERTEX_POINT('',#148201);
#36826=VERTEX_POINT('',#148206);
#36827=VERTEX_POINT('',#148228);
#36828=VERTEX_POINT('',#148233);
#36829=VERTEX_POINT('',#148255);
#36830=VERTEX_POINT('',#148260);
#36831=VERTEX_POINT('',#148282);
#36832=VERTEX_POINT('',#148287);
#36833=VERTEX_POINT('',#148309);
#36834=VERTEX_POINT('',#148314);
#36835=VERTEX_POINT('',#148336);
#36836=VERTEX_POINT('',#148341);
#36837=VERTEX_POINT('',#148363);
#36838=VERTEX_POINT('',#148368);
#36839=VERTEX_POINT('',#148390);
#36840=VERTEX_POINT('',#148395);
#36841=VERTEX_POINT('',#148417);
#36842=VERTEX_POINT('',#148422);
#36843=VERTEX_POINT('',#148444);
#36844=VERTEX_POINT('',#148449);
#36845=VERTEX_POINT('',#148471);
#36846=VERTEX_POINT('',#148476);
#36847=VERTEX_POINT('',#148498);
#36848=VERTEX_POINT('',#148503);
#36849=VERTEX_POINT('',#148525);
#36850=VERTEX_POINT('',#148530);
#36851=VERTEX_POINT('',#148552);
#36852=VERTEX_POINT('',#148557);
#36853=VERTEX_POINT('',#148579);
#36854=VERTEX_POINT('',#148584);
#36855=VERTEX_POINT('',#148606);
#36856=VERTEX_POINT('',#148611);
#36857=VERTEX_POINT('',#148633);
#36858=VERTEX_POINT('',#148638);
#36859=VERTEX_POINT('',#148660);
#36860=VERTEX_POINT('',#148665);
#36861=VERTEX_POINT('',#148687);
#36862=VERTEX_POINT('',#148692);
#36863=VERTEX_POINT('',#148714);
#36864=VERTEX_POINT('',#148719);
#36865=VERTEX_POINT('',#148741);
#36866=VERTEX_POINT('',#148746);
#36867=VERTEX_POINT('',#148768);
#36868=VERTEX_POINT('',#148773);
#36869=VERTEX_POINT('',#148784);
#36870=VERTEX_POINT('',#148787);
#36871=VERTEX_POINT('',#148800);
#36872=VERTEX_POINT('',#148805);
#36873=VERTEX_POINT('',#148827);
#36874=VERTEX_POINT('',#148832);
#36875=VERTEX_POINT('',#148854);
#36876=VERTEX_POINT('',#148859);
#36877=VERTEX_POINT('',#148881);
#36878=VERTEX_POINT('',#148886);
#36879=VERTEX_POINT('',#148908);
#36880=VERTEX_POINT('',#148913);
#36881=VERTEX_POINT('',#148935);
#36882=VERTEX_POINT('',#148940);
#36883=VERTEX_POINT('',#148962);
#36884=VERTEX_POINT('',#148967);
#36885=VERTEX_POINT('',#148989);
#36886=VERTEX_POINT('',#148994);
#36887=VERTEX_POINT('',#149016);
#36888=VERTEX_POINT('',#149021);
#36889=VERTEX_POINT('',#149043);
#36890=VERTEX_POINT('',#149048);
#36891=VERTEX_POINT('',#149070);
#36892=VERTEX_POINT('',#149075);
#36893=VERTEX_POINT('',#149097);
#36894=VERTEX_POINT('',#149102);
#36895=VERTEX_POINT('',#149124);
#36896=VERTEX_POINT('',#149129);
#36897=VERTEX_POINT('',#149151);
#36898=VERTEX_POINT('',#149156);
#36899=VERTEX_POINT('',#149178);
#36900=VERTEX_POINT('',#149183);
#36901=VERTEX_POINT('',#149205);
#36902=VERTEX_POINT('',#149210);
#36903=VERTEX_POINT('',#149232);
#36904=VERTEX_POINT('',#149237);
#36905=VERTEX_POINT('',#149259);
#36906=VERTEX_POINT('',#149264);
#36907=VERTEX_POINT('',#149286);
#36908=VERTEX_POINT('',#149291);
#36909=VERTEX_POINT('',#149313);
#36910=VERTEX_POINT('',#149318);
#36911=VERTEX_POINT('',#149340);
#36912=VERTEX_POINT('',#149345);
#36913=VERTEX_POINT('',#149367);
#36914=VERTEX_POINT('',#149372);
#36915=VERTEX_POINT('',#149394);
#36916=VERTEX_POINT('',#149399);
#36917=VERTEX_POINT('',#149421);
#36918=VERTEX_POINT('',#149426);
#36919=VERTEX_POINT('',#149448);
#36920=VERTEX_POINT('',#149453);
#36921=VERTEX_POINT('',#149475);
#36922=VERTEX_POINT('',#149480);
#36923=VERTEX_POINT('',#149502);
#36924=VERTEX_POINT('',#149507);
#36925=VERTEX_POINT('',#149529);
#36926=VERTEX_POINT('',#149534);
#36927=VERTEX_POINT('',#149556);
#36928=VERTEX_POINT('',#149561);
#36929=VERTEX_POINT('',#149583);
#36930=VERTEX_POINT('',#149588);
#36931=VERTEX_POINT('',#149610);
#36932=VERTEX_POINT('',#149615);
#36933=VERTEX_POINT('',#149637);
#36934=VERTEX_POINT('',#149642);
#36935=VERTEX_POINT('',#149664);
#36936=VERTEX_POINT('',#149669);
#36937=VERTEX_POINT('',#149691);
#36938=VERTEX_POINT('',#149696);
#36939=VERTEX_POINT('',#149723);
#36940=VERTEX_POINT('',#149725);
#36941=VERTEX_POINT('',#149742);
#36942=VERTEX_POINT('',#149749);
#36943=VERTEX_POINT('',#149775);
#36944=VERTEX_POINT('',#149782);
#36945=VERTEX_POINT('',#149808);
#36946=VERTEX_POINT('',#149815);
#36947=VERTEX_POINT('',#149841);
#36948=VERTEX_POINT('',#149848);
#36949=VERTEX_POINT('',#149874);
#36950=VERTEX_POINT('',#149881);
#36951=VERTEX_POINT('',#149907);
#36952=VERTEX_POINT('',#149914);
#36953=VERTEX_POINT('',#149940);
#36954=VERTEX_POINT('',#149947);
#36955=VERTEX_POINT('',#149973);
#36956=VERTEX_POINT('',#149980);
#36957=VERTEX_POINT('',#150006);
#36958=VERTEX_POINT('',#150013);
#36959=VERTEX_POINT('',#150039);
#36960=VERTEX_POINT('',#150046);
#36961=VERTEX_POINT('',#150072);
#36962=VERTEX_POINT('',#150079);
#36963=VERTEX_POINT('',#150105);
#36964=VERTEX_POINT('',#150112);
#36965=VERTEX_POINT('',#150138);
#36966=VERTEX_POINT('',#150145);
#36967=VERTEX_POINT('',#150171);
#36968=VERTEX_POINT('',#150178);
#36969=VERTEX_POINT('',#150204);
#36970=VERTEX_POINT('',#150211);
#36971=VERTEX_POINT('',#150237);
#36972=VERTEX_POINT('',#150244);
#36973=VERTEX_POINT('',#150270);
#36974=VERTEX_POINT('',#150277);
#36975=VERTEX_POINT('',#150303);
#36976=VERTEX_POINT('',#150310);
#36977=VERTEX_POINT('',#150336);
#36978=VERTEX_POINT('',#150343);
#36979=VERTEX_POINT('',#150369);
#36980=VERTEX_POINT('',#150376);
#36981=VERTEX_POINT('',#150402);
#36982=VERTEX_POINT('',#150409);
#36983=VERTEX_POINT('',#150435);
#36984=VERTEX_POINT('',#150442);
#36985=VERTEX_POINT('',#150468);
#36986=VERTEX_POINT('',#150475);
#36987=VERTEX_POINT('',#150501);
#36988=VERTEX_POINT('',#150508);
#36989=VERTEX_POINT('',#150534);
#36990=VERTEX_POINT('',#150541);
#36991=VERTEX_POINT('',#150567);
#36992=VERTEX_POINT('',#150574);
#36993=VERTEX_POINT('',#150600);
#36994=VERTEX_POINT('',#150607);
#36995=VERTEX_POINT('',#150633);
#36996=VERTEX_POINT('',#150640);
#36997=VERTEX_POINT('',#150666);
#36998=VERTEX_POINT('',#150673);
#36999=VERTEX_POINT('',#150699);
#37000=VERTEX_POINT('',#150706);
#37001=VERTEX_POINT('',#150732);
#37002=VERTEX_POINT('',#150739);
#37003=VERTEX_POINT('',#150765);
#37004=VERTEX_POINT('',#150772);
#37005=VERTEX_POINT('',#150798);
#37006=VERTEX_POINT('',#150805);
#37007=VERTEX_POINT('',#150831);
#37008=VERTEX_POINT('',#150838);
#37009=VERTEX_POINT('',#150864);
#37010=VERTEX_POINT('',#150871);
#37011=VERTEX_POINT('',#150897);
#37012=VERTEX_POINT('',#150904);
#37013=VERTEX_POINT('',#150930);
#37014=VERTEX_POINT('',#150937);
#37015=VERTEX_POINT('',#150963);
#37016=VERTEX_POINT('',#150970);
#37017=VERTEX_POINT('',#150996);
#37018=VERTEX_POINT('',#151003);
#37019=VERTEX_POINT('',#151029);
#37020=VERTEX_POINT('',#151036);
#37021=VERTEX_POINT('',#151062);
#37022=VERTEX_POINT('',#151069);
#37023=VERTEX_POINT('',#151095);
#37024=VERTEX_POINT('',#151102);
#37025=VERTEX_POINT('',#151128);
#37026=VERTEX_POINT('',#151135);
#37027=VERTEX_POINT('',#151161);
#37028=VERTEX_POINT('',#151168);
#37029=VERTEX_POINT('',#151194);
#37030=VERTEX_POINT('',#151201);
#37031=VERTEX_POINT('',#151227);
#37032=VERTEX_POINT('',#151234);
#37033=VERTEX_POINT('',#151260);
#37034=VERTEX_POINT('',#151267);
#37035=VERTEX_POINT('',#151293);
#37036=VERTEX_POINT('',#151300);
#37037=VERTEX_POINT('',#151326);
#37038=VERTEX_POINT('',#151333);
#37039=VERTEX_POINT('',#151359);
#37040=VERTEX_POINT('',#151366);
#37041=VERTEX_POINT('',#151392);
#37042=VERTEX_POINT('',#151399);
#37043=VERTEX_POINT('',#151425);
#37044=VERTEX_POINT('',#151432);
#37045=VERTEX_POINT('',#151458);
#37046=VERTEX_POINT('',#151465);
#37047=VERTEX_POINT('',#151491);
#37048=VERTEX_POINT('',#151498);
#37049=VERTEX_POINT('',#151524);
#37050=VERTEX_POINT('',#151531);
#37051=VERTEX_POINT('',#151557);
#37052=VERTEX_POINT('',#151564);
#37053=VERTEX_POINT('',#151590);
#37054=VERTEX_POINT('',#151597);
#37055=VERTEX_POINT('',#151623);
#37056=VERTEX_POINT('',#151630);
#37057=VERTEX_POINT('',#151656);
#37058=VERTEX_POINT('',#151663);
#37059=VERTEX_POINT('',#151689);
#37060=VERTEX_POINT('',#151696);
#37061=VERTEX_POINT('',#151722);
#37062=VERTEX_POINT('',#151729);
#37063=VERTEX_POINT('',#151755);
#37064=VERTEX_POINT('',#151762);
#37065=VERTEX_POINT('',#151788);
#37066=VERTEX_POINT('',#151795);
#37067=VERTEX_POINT('',#151821);
#37068=VERTEX_POINT('',#151828);
#37069=VERTEX_POINT('',#151854);
#37070=VERTEX_POINT('',#151861);
#37071=VERTEX_POINT('',#151887);
#37072=VERTEX_POINT('',#151894);
#37073=VERTEX_POINT('',#151920);
#37074=VERTEX_POINT('',#151927);
#37075=VERTEX_POINT('',#151953);
#37076=VERTEX_POINT('',#151960);
#37077=VERTEX_POINT('',#151986);
#37078=VERTEX_POINT('',#151993);
#37079=VERTEX_POINT('',#152019);
#37080=VERTEX_POINT('',#152037);
#37081=VERTEX_POINT('',#152396);
#37082=VERTEX_POINT('',#152398);
#37083=VERTEX_POINT('',#152402);
#37084=VERTEX_POINT('',#152404);
#37085=VERTEX_POINT('',#152408);
#37086=VERTEX_POINT('',#152410);
#37087=VERTEX_POINT('',#152414);
#37088=VERTEX_POINT('',#152416);
#37089=VERTEX_POINT('',#152420);
#37090=VERTEX_POINT('',#152421);
#37091=VERTEX_POINT('',#152423);
#37092=VERTEX_POINT('',#152428);
#37093=VERTEX_POINT('',#152430);
#37094=VERTEX_POINT('',#152434);
#37095=VERTEX_POINT('',#152436);
#37096=VERTEX_POINT('',#152438);
#37097=VERTEX_POINT('',#152442);
#37098=VERTEX_POINT('',#152443);
#37099=VERTEX_POINT('',#152445);
#37100=VERTEX_POINT('',#152447);
#37101=VERTEX_POINT('',#152451);
#37102=VERTEX_POINT('',#152452);
#37103=VERTEX_POINT('',#152454);
#37104=VERTEX_POINT('',#152456);
#37105=VERTEX_POINT('',#152460);
#37106=VERTEX_POINT('',#152462);
#37107=VERTEX_POINT('',#152464);
#37108=VERTEX_POINT('',#152468);
#37109=VERTEX_POINT('',#152470);
#37110=VERTEX_POINT('',#152472);
#37111=VERTEX_POINT('',#152476);
#37112=VERTEX_POINT('',#152478);
#37113=VERTEX_POINT('',#152480);
#37114=VERTEX_POINT('',#152484);
#37115=VERTEX_POINT('',#152485);
#37116=VERTEX_POINT('',#152487);
#37117=VERTEX_POINT('',#152489);
#37118=VERTEX_POINT('',#152493);
#37119=VERTEX_POINT('',#152494);
#37120=VERTEX_POINT('',#152496);
#37121=VERTEX_POINT('',#152498);
#37122=VERTEX_POINT('',#152502);
#37123=VERTEX_POINT('',#152510);
#37124=VERTEX_POINT('',#152514);
#37125=VERTEX_POINT('',#152515);
#37126=VERTEX_POINT('',#152517);
#37127=VERTEX_POINT('',#152519);
#37128=VERTEX_POINT('',#152523);
#37129=VERTEX_POINT('',#152524);
#37130=VERTEX_POINT('',#152526);
#37131=VERTEX_POINT('',#152528);
#37132=VERTEX_POINT('',#152532);
#37133=VERTEX_POINT('',#152533);
#37134=VERTEX_POINT('',#152535);
#37135=VERTEX_POINT('',#152537);
#37136=VERTEX_POINT('',#152541);
#37137=VERTEX_POINT('',#152542);
#37138=VERTEX_POINT('',#152544);
#37139=VERTEX_POINT('',#152546);
#37140=VERTEX_POINT('',#152552);
#37141=VERTEX_POINT('',#152553);
#37142=VERTEX_POINT('',#152555);
#37143=VERTEX_POINT('',#152557);
#37144=VERTEX_POINT('',#152559);
#37145=VERTEX_POINT('',#152561);
#37146=VERTEX_POINT('',#152563);
#37147=VERTEX_POINT('',#152565);
#37148=VERTEX_POINT('',#152567);
#37149=VERTEX_POINT('',#152569);
#37150=VERTEX_POINT('',#152571);
#37151=VERTEX_POINT('',#152573);
#37152=VERTEX_POINT('',#152575);
#37153=VERTEX_POINT('',#152577);
#37154=VERTEX_POINT('',#152579);
#37155=VERTEX_POINT('',#152581);
#37156=VERTEX_POINT('',#152583);
#37157=VERTEX_POINT('',#152585);
#37158=VERTEX_POINT('',#152587);
#37159=VERTEX_POINT('',#152589);
#37160=VERTEX_POINT('',#152591);
#37161=VERTEX_POINT('',#152593);
#37162=VERTEX_POINT('',#152595);
#37163=VERTEX_POINT('',#152597);
#37164=VERTEX_POINT('',#152599);
#37165=VERTEX_POINT('',#152601);
#37166=VERTEX_POINT('',#152603);
#37167=VERTEX_POINT('',#152605);
#37168=VERTEX_POINT('',#152607);
#37169=VERTEX_POINT('',#152609);
#37170=VERTEX_POINT('',#152612);
#37171=VERTEX_POINT('',#152614);
#37172=VERTEX_POINT('',#152617);
#37173=VERTEX_POINT('',#152619);
#37174=VERTEX_POINT('',#152621);
#37175=VERTEX_POINT('',#152623);
#37176=VERTEX_POINT('',#152625);
#37177=VERTEX_POINT('',#152627);
#37178=VERTEX_POINT('',#152629);
#37179=VERTEX_POINT('',#152631);
#37180=VERTEX_POINT('',#152633);
#37181=VERTEX_POINT('',#152635);
#37182=VERTEX_POINT('',#152637);
#37183=VERTEX_POINT('',#152639);
#37184=VERTEX_POINT('',#152641);
#37185=VERTEX_POINT('',#152643);
#37186=VERTEX_POINT('',#152645);
#37187=VERTEX_POINT('',#152647);
#37188=VERTEX_POINT('',#152649);
#37189=VERTEX_POINT('',#152651);
#37190=VERTEX_POINT('',#152653);
#37191=VERTEX_POINT('',#152655);
#37192=VERTEX_POINT('',#152657);
#37193=VERTEX_POINT('',#152659);
#37194=VERTEX_POINT('',#152661);
#37195=VERTEX_POINT('',#152663);
#37196=VERTEX_POINT('',#152665);
#37197=VERTEX_POINT('',#152667);
#37198=VERTEX_POINT('',#152669);
#37199=VERTEX_POINT('',#152671);
#37200=VERTEX_POINT('',#152673);
#37201=VERTEX_POINT('',#152675);
#37202=VERTEX_POINT('',#152677);
#37203=VERTEX_POINT('',#152679);
#37204=VERTEX_POINT('',#152681);
#37205=VERTEX_POINT('',#152683);
#37206=VERTEX_POINT('',#152685);
#37207=VERTEX_POINT('',#152687);
#37208=VERTEX_POINT('',#152689);
#37209=VERTEX_POINT('',#152691);
#37210=VERTEX_POINT('',#152693);
#37211=VERTEX_POINT('',#152695);
#37212=VERTEX_POINT('',#152697);
#37213=VERTEX_POINT('',#152699);
#37214=VERTEX_POINT('',#152701);
#37215=VERTEX_POINT('',#152703);
#37216=VERTEX_POINT('',#152705);
#37217=VERTEX_POINT('',#152707);
#37218=VERTEX_POINT('',#152709);
#37219=VERTEX_POINT('',#152711);
#37220=VERTEX_POINT('',#152713);
#37221=VERTEX_POINT('',#152715);
#37222=VERTEX_POINT('',#152717);
#37223=VERTEX_POINT('',#152719);
#37224=VERTEX_POINT('',#152721);
#37225=VERTEX_POINT('',#152723);
#37226=VERTEX_POINT('',#152725);
#37227=VERTEX_POINT('',#152727);
#37228=VERTEX_POINT('',#152729);
#37229=VERTEX_POINT('',#152731);
#37230=VERTEX_POINT('',#152733);
#37231=VERTEX_POINT('',#152735);
#37232=VERTEX_POINT('',#152737);
#37233=VERTEX_POINT('',#152739);
#37234=VERTEX_POINT('',#152741);
#37235=VERTEX_POINT('',#152743);
#37236=VERTEX_POINT('',#152745);
#37237=VERTEX_POINT('',#152747);
#37238=VERTEX_POINT('',#152749);
#37239=VERTEX_POINT('',#152751);
#37240=VERTEX_POINT('',#152753);
#37241=VERTEX_POINT('',#152755);
#37242=VERTEX_POINT('',#152757);
#37243=VERTEX_POINT('',#152759);
#37244=VERTEX_POINT('',#152761);
#37245=VERTEX_POINT('',#152763);
#37246=VERTEX_POINT('',#152765);
#37247=VERTEX_POINT('',#152767);
#37248=VERTEX_POINT('',#152769);
#37249=VERTEX_POINT('',#152771);
#37250=VERTEX_POINT('',#152773);
#37251=VERTEX_POINT('',#152775);
#37252=VERTEX_POINT('',#152777);
#37253=VERTEX_POINT('',#152779);
#37254=VERTEX_POINT('',#152781);
#37255=VERTEX_POINT('',#152783);
#37256=VERTEX_POINT('',#152786);
#37257=VERTEX_POINT('',#152788);
#37258=VERTEX_POINT('',#152791);
#37259=VERTEX_POINT('',#152793);
#37260=VERTEX_POINT('',#152795);
#37261=VERTEX_POINT('',#152797);
#37262=VERTEX_POINT('',#152799);
#37263=VERTEX_POINT('',#152801);
#37264=VERTEX_POINT('',#152803);
#37265=VERTEX_POINT('',#152805);
#37266=VERTEX_POINT('',#152807);
#37267=VERTEX_POINT('',#152809);
#37268=VERTEX_POINT('',#152811);
#37269=VERTEX_POINT('',#152813);
#37270=VERTEX_POINT('',#152815);
#37271=VERTEX_POINT('',#152817);
#37272=VERTEX_POINT('',#152819);
#37273=VERTEX_POINT('',#152821);
#37274=VERTEX_POINT('',#152823);
#37275=VERTEX_POINT('',#152825);
#37276=VERTEX_POINT('',#152827);
#37277=VERTEX_POINT('',#152829);
#37278=VERTEX_POINT('',#152831);
#37279=VERTEX_POINT('',#152833);
#37280=VERTEX_POINT('',#152836);
#37281=VERTEX_POINT('',#152837);
#37282=VERTEX_POINT('',#152839);
#37283=VERTEX_POINT('',#152842);
#37284=VERTEX_POINT('',#152844);
#37285=VERTEX_POINT('',#152846);
#37286=VERTEX_POINT('',#152849);
#37287=VERTEX_POINT('',#152850);
#37288=VERTEX_POINT('',#152852);
#37289=VERTEX_POINT('',#152855);
#37290=VERTEX_POINT('',#152857);
#37291=VERTEX_POINT('',#152859);
#37292=VERTEX_POINT('',#152863);
#37293=VERTEX_POINT('',#152865);
#37294=VERTEX_POINT('',#152869);
#37295=VERTEX_POINT('',#152871);
#37296=VERTEX_POINT('',#152875);
#37297=VERTEX_POINT('',#152877);
#37298=VERTEX_POINT('',#152881);
#37299=VERTEX_POINT('',#152883);
#37300=VERTEX_POINT('',#152887);
#37301=VERTEX_POINT('',#152889);
#37302=VERTEX_POINT('',#152893);
#37303=VERTEX_POINT('',#152897);
#37304=VERTEX_POINT('',#152901);
#37305=VERTEX_POINT('',#152903);
#37306=VERTEX_POINT('',#152907);
#37307=VERTEX_POINT('',#152909);
#37308=VERTEX_POINT('',#152913);
#37309=VERTEX_POINT('',#152915);
#37310=VERTEX_POINT('',#152919);
#37311=VERTEX_POINT('',#152921);
#37312=VERTEX_POINT('',#152925);
#37313=VERTEX_POINT('',#152927);
#37314=VERTEX_POINT('',#152931);
#37315=VERTEX_POINT('',#152935);
#37316=VERTEX_POINT('',#152939);
#37317=VERTEX_POINT('',#152941);
#37318=VERTEX_POINT('',#152945);
#37319=VERTEX_POINT('',#152947);
#37320=VERTEX_POINT('',#152951);
#37321=VERTEX_POINT('',#152953);
#37322=VERTEX_POINT('',#152957);
#37323=VERTEX_POINT('',#152959);
#37324=VERTEX_POINT('',#152963);
#37325=VERTEX_POINT('',#152965);
#37326=VERTEX_POINT('',#152969);
#37327=VERTEX_POINT('',#152971);
#37328=VERTEX_POINT('',#152975);
#37329=VERTEX_POINT('',#152977);
#37330=VERTEX_POINT('',#152981);
#37331=VERTEX_POINT('',#152983);
#37332=VERTEX_POINT('',#152987);
#37333=VERTEX_POINT('',#152989);
#37334=VERTEX_POINT('',#152993);
#37335=VERTEX_POINT('',#152995);
#37336=VERTEX_POINT('',#152999);
#37337=VERTEX_POINT('',#153001);
#37338=VERTEX_POINT('',#153005);
#37339=VERTEX_POINT('',#153007);
#37340=VERTEX_POINT('',#153011);
#37341=VERTEX_POINT('',#153013);
#37342=VERTEX_POINT('',#153017);
#37343=VERTEX_POINT('',#153019);
#37344=VERTEX_POINT('',#153023);
#37345=VERTEX_POINT('',#153025);
#37346=VERTEX_POINT('',#153029);
#37347=VERTEX_POINT('',#153031);
#37348=VERTEX_POINT('',#153035);
#37349=VERTEX_POINT('',#153037);
#37350=VERTEX_POINT('',#153041);
#37351=VERTEX_POINT('',#153043);
#37352=VERTEX_POINT('',#153047);
#37353=VERTEX_POINT('',#153049);
#37354=VERTEX_POINT('',#153053);
#37355=VERTEX_POINT('',#153055);
#37356=VERTEX_POINT('',#153059);
#37357=VERTEX_POINT('',#153061);
#37358=VERTEX_POINT('',#153065);
#37359=VERTEX_POINT('',#153067);
#37360=VERTEX_POINT('',#153071);
#37361=VERTEX_POINT('',#153073);
#37362=VERTEX_POINT('',#153075);
#37363=VERTEX_POINT('',#153078);
#37364=VERTEX_POINT('',#153080);
#37365=VERTEX_POINT('',#153083);
#37366=VERTEX_POINT('',#153085);
#37367=VERTEX_POINT('',#153088);
#37368=VERTEX_POINT('',#153090);
#37369=VERTEX_POINT('',#153093);
#37370=VERTEX_POINT('',#153095);
#37371=VERTEX_POINT('',#153098);
#37372=VERTEX_POINT('',#153101);
#37373=VERTEX_POINT('',#153104);
#37374=VERTEX_POINT('',#153106);
#37375=VERTEX_POINT('',#153108);
#37376=VERTEX_POINT('',#153110);
#37377=VERTEX_POINT('',#153112);
#37378=VERTEX_POINT('',#153114);
#37379=VERTEX_POINT('',#153117);
#37380=VERTEX_POINT('',#153119);
#37381=VERTEX_POINT('',#153122);
#37382=VERTEX_POINT('',#153124);
#37383=VERTEX_POINT('',#153127);
#37384=VERTEX_POINT('',#153129);
#37385=VERTEX_POINT('',#153132);
#37386=VERTEX_POINT('',#153134);
#37387=VERTEX_POINT('',#153137);
#37388=VERTEX_POINT('',#153139);
#37389=VERTEX_POINT('',#153142);
#37390=VERTEX_POINT('',#153144);
#37391=VERTEX_POINT('',#153147);
#37392=VERTEX_POINT('',#153149);
#37393=VERTEX_POINT('',#153152);
#37394=VERTEX_POINT('',#153154);
#37395=VERTEX_POINT('',#153157);
#37396=VERTEX_POINT('',#153159);
#37397=VERTEX_POINT('',#153162);
#37398=VERTEX_POINT('',#153164);
#37399=VERTEX_POINT('',#153167);
#37400=VERTEX_POINT('',#153169);
#37401=VERTEX_POINT('',#153172);
#37402=VERTEX_POINT('',#153174);
#37403=VERTEX_POINT('',#153177);
#37404=VERTEX_POINT('',#153179);
#37405=VERTEX_POINT('',#153182);
#37406=VERTEX_POINT('',#153184);
#37407=VERTEX_POINT('',#153187);
#37408=VERTEX_POINT('',#153189);
#37409=VERTEX_POINT('',#153192);
#37410=VERTEX_POINT('',#153194);
#37411=VERTEX_POINT('',#153197);
#37412=VERTEX_POINT('',#153199);
#37413=VERTEX_POINT('',#153202);
#37414=VERTEX_POINT('',#153204);
#37415=VERTEX_POINT('',#153207);
#37416=VERTEX_POINT('',#153209);
#37417=VERTEX_POINT('',#153212);
#37418=VERTEX_POINT('',#153215);
#37419=VERTEX_POINT('',#153218);
#37420=VERTEX_POINT('',#153220);
#37421=VERTEX_POINT('',#153223);
#37422=VERTEX_POINT('',#153225);
#37423=VERTEX_POINT('',#153228);
#37424=VERTEX_POINT('',#153230);
#37425=VERTEX_POINT('',#153233);
#37426=VERTEX_POINT('',#153235);
#37427=VERTEX_POINT('',#153238);
#37428=VERTEX_POINT('',#153240);
#37429=VERTEX_POINT('',#153243);
#37430=VERTEX_POINT('',#153245);
#37431=VERTEX_POINT('',#153248);
#37432=VERTEX_POINT('',#153436);
#37433=VERTEX_POINT('',#153437);
#37434=VERTEX_POINT('',#153442);
#37435=VERTEX_POINT('',#153443);
#37436=VERTEX_POINT('',#153448);
#37437=VERTEX_POINT('',#153449);
#37438=VERTEX_POINT('',#153454);
#37439=VERTEX_POINT('',#153455);
#37440=VERTEX_POINT('',#153460);
#37441=VERTEX_POINT('',#153465);
#37442=VERTEX_POINT('',#153473);
#37443=VERTEX_POINT('',#153474);
#37444=VERTEX_POINT('',#153476);
#37445=VERTEX_POINT('',#153478);
#37446=VERTEX_POINT('',#153485);
#37447=VERTEX_POINT('',#153490);
#37448=VERTEX_POINT('',#153494);
#37449=VERTEX_POINT('',#153495);
#37450=VERTEX_POINT('',#153500);
#37451=VERTEX_POINT('',#153501);
#46419=EDGE_CURVE('',#36496,#36497,#23757,.T.);
#46420=EDGE_CURVE('',#36496,#36498,#19464,.T.);
#46421=EDGE_CURVE('',#36499,#36498,#23758,.T.);
#46422=EDGE_CURVE('',#36497,#36499,#19465,.T.);
#46423=EDGE_CURVE('',#36500,#36501,#23759,.T.);
#46424=EDGE_CURVE('',#36500,#36502,#19466,.T.);
#46425=EDGE_CURVE('',#36503,#36502,#23760,.T.);
#46426=EDGE_CURVE('',#36501,#36503,#19467,.T.);
#46427=EDGE_CURVE('',#36504,#36505,#23761,.T.);
#46428=EDGE_CURVE('',#36504,#36506,#19468,.T.);
#46429=EDGE_CURVE('',#36507,#36506,#23762,.T.);
#46430=EDGE_CURVE('',#36505,#36507,#19469,.T.);
#46431=EDGE_CURVE('',#36508,#36509,#23763,.T.);
#46432=EDGE_CURVE('',#36508,#36510,#19470,.T.);
#46433=EDGE_CURVE('',#36511,#36510,#23764,.T.);
#46434=EDGE_CURVE('',#36509,#36511,#19471,.T.);
#46435=EDGE_CURVE('',#36512,#36513,#23765,.T.);
#46436=EDGE_CURVE('',#36512,#36514,#19472,.T.);
#46437=EDGE_CURVE('',#36515,#36514,#23766,.T.);
#46438=EDGE_CURVE('',#36513,#36515,#19473,.T.);
#46439=EDGE_CURVE('',#36516,#36517,#23767,.T.);
#46440=EDGE_CURVE('',#36516,#36518,#19474,.T.);
#46441=EDGE_CURVE('',#36519,#36518,#23768,.T.);
#46442=EDGE_CURVE('',#36517,#36519,#19475,.T.);
#46443=EDGE_CURVE('',#36520,#36521,#23769,.T.);
#46444=EDGE_CURVE('',#36520,#36522,#19476,.T.);
#46445=EDGE_CURVE('',#36523,#36522,#23770,.T.);
#46446=EDGE_CURVE('',#36521,#36523,#19477,.T.);
#46447=EDGE_CURVE('',#36524,#36525,#23771,.T.);
#46448=EDGE_CURVE('',#36524,#36526,#19478,.T.);
#46449=EDGE_CURVE('',#36527,#36526,#23772,.T.);
#46450=EDGE_CURVE('',#36525,#36527,#19479,.T.);
#46451=EDGE_CURVE('',#36528,#36529,#23773,.T.);
#46452=EDGE_CURVE('',#36528,#36530,#19480,.T.);
#46453=EDGE_CURVE('',#36531,#36530,#23774,.T.);
#46454=EDGE_CURVE('',#36529,#36531,#19481,.T.);
#46455=EDGE_CURVE('',#36532,#36533,#23775,.T.);
#46456=EDGE_CURVE('',#36532,#36534,#19482,.T.);
#46457=EDGE_CURVE('',#36535,#36534,#23776,.T.);
#46458=EDGE_CURVE('',#36533,#36535,#19483,.T.);
#46459=EDGE_CURVE('',#36536,#36537,#23777,.T.);
#46460=EDGE_CURVE('',#36536,#36538,#19484,.T.);
#46461=EDGE_CURVE('',#36539,#36538,#23778,.T.);
#46462=EDGE_CURVE('',#36537,#36539,#19485,.T.);
#46463=EDGE_CURVE('',#36540,#36541,#23779,.T.);
#46464=EDGE_CURVE('',#36540,#36542,#19486,.T.);
#46465=EDGE_CURVE('',#36543,#36542,#23780,.T.);
#46466=EDGE_CURVE('',#36541,#36543,#19487,.T.);
#46467=EDGE_CURVE('',#36544,#36545,#23781,.T.);
#46468=EDGE_CURVE('',#36544,#36546,#19488,.T.);
#46469=EDGE_CURVE('',#36547,#36546,#23782,.T.);
#46470=EDGE_CURVE('',#36545,#36547,#19489,.T.);
#46471=EDGE_CURVE('',#36548,#36549,#23783,.T.);
#46472=EDGE_CURVE('',#36548,#36550,#19490,.T.);
#46473=EDGE_CURVE('',#36551,#36550,#23784,.T.);
#46474=EDGE_CURVE('',#36549,#36551,#19491,.T.);
#46475=EDGE_CURVE('',#36552,#36553,#23785,.T.);
#46476=EDGE_CURVE('',#36552,#36554,#19492,.T.);
#46477=EDGE_CURVE('',#36555,#36554,#23786,.T.);
#46478=EDGE_CURVE('',#36553,#36555,#19493,.T.);
#46479=EDGE_CURVE('',#36556,#36557,#23787,.T.);
#46480=EDGE_CURVE('',#36556,#36558,#19494,.T.);
#46481=EDGE_CURVE('',#36559,#36558,#23788,.T.);
#46482=EDGE_CURVE('',#36557,#36559,#19495,.T.);
#46483=EDGE_CURVE('',#36560,#36561,#23789,.T.);
#46484=EDGE_CURVE('',#36560,#36562,#19496,.T.);
#46485=EDGE_CURVE('',#36563,#36562,#23790,.T.);
#46486=EDGE_CURVE('',#36561,#36563,#19497,.T.);
#46487=EDGE_CURVE('',#36564,#36565,#23791,.T.);
#46488=EDGE_CURVE('',#36564,#36566,#19498,.T.);
#46489=EDGE_CURVE('',#36567,#36566,#23792,.T.);
#46490=EDGE_CURVE('',#36565,#36567,#19499,.T.);
#46491=EDGE_CURVE('',#36568,#36569,#23793,.T.);
#46492=EDGE_CURVE('',#36568,#36570,#19500,.T.);
#46493=EDGE_CURVE('',#36571,#36570,#23794,.T.);
#46494=EDGE_CURVE('',#36569,#36571,#19501,.T.);
#46495=EDGE_CURVE('',#36572,#36573,#23795,.T.);
#46496=EDGE_CURVE('',#36572,#36574,#19502,.T.);
#46497=EDGE_CURVE('',#36575,#36574,#23796,.T.);
#46498=EDGE_CURVE('',#36573,#36575,#19503,.T.);
#46499=EDGE_CURVE('',#36576,#36577,#23797,.T.);
#46500=EDGE_CURVE('',#36576,#36578,#19504,.T.);
#46501=EDGE_CURVE('',#36579,#36578,#23798,.T.);
#46502=EDGE_CURVE('',#36577,#36579,#19505,.T.);
#46503=EDGE_CURVE('',#36580,#36581,#23799,.T.);
#46504=EDGE_CURVE('',#36580,#36582,#19506,.T.);
#46505=EDGE_CURVE('',#36583,#36582,#23800,.T.);
#46506=EDGE_CURVE('',#36581,#36583,#19507,.T.);
#46507=EDGE_CURVE('',#36584,#36585,#23801,.T.);
#46508=EDGE_CURVE('',#36584,#36586,#19508,.T.);
#46509=EDGE_CURVE('',#36587,#36586,#23802,.T.);
#46510=EDGE_CURVE('',#36585,#36587,#19509,.T.);
#46511=EDGE_CURVE('',#36588,#36589,#23803,.T.);
#46512=EDGE_CURVE('',#36588,#36590,#19510,.T.);
#46513=EDGE_CURVE('',#36591,#36590,#23804,.T.);
#46514=EDGE_CURVE('',#36589,#36591,#19511,.T.);
#46515=EDGE_CURVE('',#36592,#36593,#23805,.T.);
#46516=EDGE_CURVE('',#36592,#36594,#19512,.T.);
#46517=EDGE_CURVE('',#36595,#36594,#23806,.T.);
#46518=EDGE_CURVE('',#36593,#36595,#19513,.T.);
#46519=EDGE_CURVE('',#36596,#36597,#23807,.T.);
#46520=EDGE_CURVE('',#36596,#36598,#19514,.T.);
#46521=EDGE_CURVE('',#36599,#36598,#23808,.T.);
#46522=EDGE_CURVE('',#36597,#36599,#19515,.T.);
#46523=EDGE_CURVE('',#36600,#36601,#23809,.T.);
#46524=EDGE_CURVE('',#36600,#36602,#19516,.T.);
#46525=EDGE_CURVE('',#36603,#36602,#23810,.T.);
#46526=EDGE_CURVE('',#36601,#36603,#19517,.T.);
#46527=EDGE_CURVE('',#36604,#36605,#23811,.T.);
#46528=EDGE_CURVE('',#36604,#36606,#19518,.T.);
#46529=EDGE_CURVE('',#36607,#36606,#23812,.T.);
#46530=EDGE_CURVE('',#36605,#36607,#19519,.T.);
#46531=EDGE_CURVE('',#36608,#36609,#23813,.T.);
#46532=EDGE_CURVE('',#36608,#36610,#19520,.T.);
#46533=EDGE_CURVE('',#36611,#36610,#23814,.T.);
#46534=EDGE_CURVE('',#36609,#36611,#19521,.T.);
#46535=EDGE_CURVE('',#36612,#36613,#23815,.T.);
#46536=EDGE_CURVE('',#36612,#36614,#19522,.T.);
#46537=EDGE_CURVE('',#36615,#36614,#23816,.T.);
#46538=EDGE_CURVE('',#36613,#36615,#19523,.T.);
#46539=EDGE_CURVE('',#36616,#36617,#23817,.T.);
#46540=EDGE_CURVE('',#36616,#36618,#19524,.T.);
#46541=EDGE_CURVE('',#36619,#36618,#23818,.T.);
#46542=EDGE_CURVE('',#36617,#36619,#19525,.T.);
#46543=EDGE_CURVE('',#36620,#36621,#23819,.T.);
#46544=EDGE_CURVE('',#36620,#36622,#19526,.T.);
#46545=EDGE_CURVE('',#36623,#36622,#23820,.T.);
#46546=EDGE_CURVE('',#36621,#36623,#19527,.T.);
#46547=EDGE_CURVE('',#36624,#36625,#23821,.T.);
#46548=EDGE_CURVE('',#36624,#36626,#19528,.T.);
#46549=EDGE_CURVE('',#36627,#36626,#23822,.T.);
#46550=EDGE_CURVE('',#36625,#36627,#19529,.T.);
#46551=EDGE_CURVE('',#36628,#36629,#23823,.T.);
#46552=EDGE_CURVE('',#36628,#36630,#19530,.T.);
#46553=EDGE_CURVE('',#36631,#36630,#23824,.T.);
#46554=EDGE_CURVE('',#36629,#36631,#19531,.T.);
#46555=EDGE_CURVE('',#36632,#36633,#23825,.T.);
#46556=EDGE_CURVE('',#36632,#36634,#19532,.T.);
#46557=EDGE_CURVE('',#36635,#36634,#23826,.T.);
#46558=EDGE_CURVE('',#36633,#36635,#19533,.T.);
#46559=EDGE_CURVE('',#36636,#36637,#23827,.T.);
#46560=EDGE_CURVE('',#36636,#36638,#19534,.T.);
#46561=EDGE_CURVE('',#36639,#36638,#23828,.T.);
#46562=EDGE_CURVE('',#36637,#36639,#19535,.T.);
#46563=EDGE_CURVE('',#36640,#36641,#23829,.T.);
#46564=EDGE_CURVE('',#36640,#36642,#19536,.T.);
#46565=EDGE_CURVE('',#36643,#36642,#23830,.T.);
#46566=EDGE_CURVE('',#36641,#36643,#19537,.T.);
#46567=EDGE_CURVE('',#36644,#36645,#23831,.T.);
#46568=EDGE_CURVE('',#36644,#36646,#19538,.T.);
#46569=EDGE_CURVE('',#36647,#36646,#23832,.T.);
#46570=EDGE_CURVE('',#36645,#36647,#19539,.T.);
#46571=EDGE_CURVE('',#36648,#36649,#23833,.T.);
#46572=EDGE_CURVE('',#36648,#36650,#19540,.T.);
#46573=EDGE_CURVE('',#36651,#36650,#23834,.T.);
#46574=EDGE_CURVE('',#36649,#36651,#19541,.T.);
#46575=EDGE_CURVE('',#36652,#36653,#23835,.T.);
#46576=EDGE_CURVE('',#36652,#36654,#19542,.T.);
#46577=EDGE_CURVE('',#36655,#36654,#23836,.T.);
#46578=EDGE_CURVE('',#36653,#36655,#19543,.T.);
#46579=EDGE_CURVE('',#36656,#36657,#23837,.T.);
#46580=EDGE_CURVE('',#36656,#36658,#19544,.T.);
#46581=EDGE_CURVE('',#36659,#36658,#23838,.T.);
#46582=EDGE_CURVE('',#36657,#36659,#19545,.T.);
#46583=EDGE_CURVE('',#36660,#36661,#23839,.T.);
#46584=EDGE_CURVE('',#36660,#36662,#19546,.T.);
#46585=EDGE_CURVE('',#36663,#36662,#23840,.T.);
#46586=EDGE_CURVE('',#36661,#36663,#19547,.T.);
#46587=EDGE_CURVE('',#36664,#36665,#23841,.T.);
#46588=EDGE_CURVE('',#36664,#36666,#19548,.T.);
#46589=EDGE_CURVE('',#36667,#36666,#23842,.T.);
#46590=EDGE_CURVE('',#36665,#36667,#19549,.T.);
#46591=EDGE_CURVE('',#36668,#36669,#23843,.T.);
#46592=EDGE_CURVE('',#36668,#36670,#19550,.T.);
#46593=EDGE_CURVE('',#36671,#36670,#23844,.T.);
#46594=EDGE_CURVE('',#36669,#36671,#19551,.T.);
#46595=EDGE_CURVE('',#36672,#36673,#23845,.T.);
#46596=EDGE_CURVE('',#36672,#36674,#19552,.T.);
#46597=EDGE_CURVE('',#36675,#36674,#23846,.T.);
#46598=EDGE_CURVE('',#36673,#36675,#19553,.T.);
#46599=EDGE_CURVE('',#36676,#36677,#23847,.T.);
#46600=EDGE_CURVE('',#36676,#36678,#19554,.T.);
#46601=EDGE_CURVE('',#36679,#36678,#23848,.T.);
#46602=EDGE_CURVE('',#36677,#36679,#19555,.T.);
#46603=EDGE_CURVE('',#36680,#36681,#23849,.T.);
#46604=EDGE_CURVE('',#36680,#36682,#19556,.T.);
#46605=EDGE_CURVE('',#36683,#36682,#23850,.T.);
#46606=EDGE_CURVE('',#36681,#36683,#19557,.T.);
#46607=EDGE_CURVE('',#36684,#36685,#23851,.T.);
#46608=EDGE_CURVE('',#36684,#36686,#19558,.T.);
#46609=EDGE_CURVE('',#36687,#36686,#23852,.T.);
#46610=EDGE_CURVE('',#36685,#36687,#19559,.T.);
#46611=EDGE_CURVE('',#36688,#36689,#23853,.T.);
#46612=EDGE_CURVE('',#36688,#36690,#19560,.T.);
#46613=EDGE_CURVE('',#36691,#36690,#23854,.T.);
#46614=EDGE_CURVE('',#36689,#36691,#19561,.T.);
#46615=EDGE_CURVE('',#36692,#36693,#23855,.T.);
#46616=EDGE_CURVE('',#36692,#36694,#19562,.T.);
#46617=EDGE_CURVE('',#36695,#36694,#23856,.T.);
#46618=EDGE_CURVE('',#36693,#36695,#19563,.T.);
#46619=EDGE_CURVE('',#36696,#36697,#23857,.T.);
#46620=EDGE_CURVE('',#36696,#36698,#19564,.T.);
#46621=EDGE_CURVE('',#36699,#36698,#23858,.T.);
#46622=EDGE_CURVE('',#36697,#36699,#19565,.T.);
#46623=EDGE_CURVE('',#36700,#36701,#23859,.T.);
#46624=EDGE_CURVE('',#36700,#36702,#19566,.T.);
#46625=EDGE_CURVE('',#36703,#36702,#23860,.T.);
#46626=EDGE_CURVE('',#36701,#36703,#19567,.T.);
#46627=EDGE_CURVE('',#36704,#36705,#23861,.T.);
#46628=EDGE_CURVE('',#36704,#36706,#19568,.T.);
#46629=EDGE_CURVE('',#36707,#36706,#23862,.T.);
#46630=EDGE_CURVE('',#36705,#36707,#19569,.T.);
#46631=EDGE_CURVE('',#36708,#36709,#23863,.T.);
#46632=EDGE_CURVE('',#36708,#36710,#19570,.T.);
#46633=EDGE_CURVE('',#36711,#36710,#23864,.T.);
#46634=EDGE_CURVE('',#36709,#36711,#19571,.T.);
#46635=EDGE_CURVE('',#36712,#36713,#23865,.T.);
#46636=EDGE_CURVE('',#36712,#36714,#19572,.T.);
#46637=EDGE_CURVE('',#36715,#36714,#23866,.T.);
#46638=EDGE_CURVE('',#36713,#36715,#19573,.T.);
#46639=EDGE_CURVE('',#36716,#36717,#23867,.T.);
#46640=EDGE_CURVE('',#36716,#36718,#19574,.T.);
#46641=EDGE_CURVE('',#36719,#36718,#23868,.T.);
#46642=EDGE_CURVE('',#36717,#36719,#19575,.T.);
#46643=EDGE_CURVE('',#36720,#36721,#23869,.T.);
#46644=EDGE_CURVE('',#36720,#36722,#19576,.T.);
#46645=EDGE_CURVE('',#36723,#36722,#23870,.T.);
#46646=EDGE_CURVE('',#36721,#36723,#19577,.T.);
#46647=EDGE_CURVE('',#36724,#36725,#23871,.T.);
#46648=EDGE_CURVE('',#36724,#36726,#19578,.T.);
#46649=EDGE_CURVE('',#36727,#36726,#23872,.T.);
#46650=EDGE_CURVE('',#36725,#36727,#19579,.T.);
#46651=EDGE_CURVE('',#36728,#36729,#23873,.T.);
#46652=EDGE_CURVE('',#36728,#36730,#19580,.T.);
#46653=EDGE_CURVE('',#36731,#36730,#23874,.T.);
#46654=EDGE_CURVE('',#36729,#36731,#19581,.T.);
#46655=EDGE_CURVE('',#36732,#36733,#23875,.T.);
#46656=EDGE_CURVE('',#36732,#36734,#19582,.T.);
#46657=EDGE_CURVE('',#36735,#36734,#23876,.T.);
#46658=EDGE_CURVE('',#36733,#36735,#19583,.T.);
#46659=EDGE_CURVE('',#36736,#36737,#23877,.T.);
#46660=EDGE_CURVE('',#36736,#36738,#19584,.T.);
#46661=EDGE_CURVE('',#36739,#36738,#23878,.T.);
#46662=EDGE_CURVE('',#36737,#36739,#19585,.T.);
#46663=EDGE_CURVE('',#36740,#36741,#23879,.T.);
#46664=EDGE_CURVE('',#36740,#36742,#19586,.T.);
#46665=EDGE_CURVE('',#36743,#36742,#23880,.T.);
#46666=EDGE_CURVE('',#36741,#36743,#19587,.T.);
#46667=EDGE_CURVE('',#36744,#36745,#23881,.T.);
#46668=EDGE_CURVE('',#36744,#36746,#19588,.T.);
#46669=EDGE_CURVE('',#36747,#36746,#23882,.T.);
#46670=EDGE_CURVE('',#36745,#36747,#19589,.T.);
#46671=EDGE_CURVE('',#36748,#36749,#23883,.T.);
#46672=EDGE_CURVE('',#36748,#36750,#19590,.T.);
#46673=EDGE_CURVE('',#36751,#36750,#23884,.T.);
#46674=EDGE_CURVE('',#36749,#36751,#19591,.T.);
#46675=EDGE_CURVE('',#36752,#36753,#23885,.T.);
#46676=EDGE_CURVE('',#36752,#36754,#19592,.T.);
#46677=EDGE_CURVE('',#36755,#36754,#23886,.T.);
#46678=EDGE_CURVE('',#36753,#36755,#19593,.T.);
#46679=EDGE_CURVE('',#36756,#36757,#23887,.T.);
#46680=EDGE_CURVE('',#36756,#36758,#19594,.T.);
#46681=EDGE_CURVE('',#36759,#36758,#23888,.T.);
#46682=EDGE_CURVE('',#36757,#36759,#19595,.T.);
#46683=EDGE_CURVE('',#36760,#36761,#23889,.T.);
#46684=EDGE_CURVE('',#36760,#36762,#19596,.T.);
#46685=EDGE_CURVE('',#36763,#36762,#23890,.T.);
#46686=EDGE_CURVE('',#36761,#36763,#19597,.T.);
#46687=EDGE_CURVE('',#36764,#36765,#23891,.T.);
#46688=EDGE_CURVE('',#36764,#36766,#19598,.T.);
#46689=EDGE_CURVE('',#36767,#36766,#23892,.T.);
#46690=EDGE_CURVE('',#36765,#36767,#19599,.T.);
#46691=EDGE_CURVE('',#36768,#36769,#23893,.T.);
#46692=EDGE_CURVE('',#36768,#36770,#19600,.T.);
#46693=EDGE_CURVE('',#36771,#36770,#23894,.T.);
#46694=EDGE_CURVE('',#36769,#36771,#19601,.T.);
#46695=EDGE_CURVE('',#36772,#36773,#23895,.T.);
#46696=EDGE_CURVE('',#36772,#36774,#19602,.T.);
#46697=EDGE_CURVE('',#36775,#36774,#23896,.T.);
#46698=EDGE_CURVE('',#36773,#36775,#19603,.T.);
#46699=EDGE_CURVE('',#36776,#36777,#19604,.T.);
#46700=EDGE_CURVE('',#36776,#36778,#28290,.T.);
#46701=EDGE_CURVE('',#36778,#36778,#19605,.T.);
#46702=EDGE_CURVE('',#36777,#36776,#19606,.T.);
#46703=EDGE_CURVE('',#36779,#36780,#19607,.T.);
#46704=EDGE_CURVE('',#36779,#36781,#28291,.T.);
#46705=EDGE_CURVE('',#36781,#36781,#19608,.T.);
#46706=EDGE_CURVE('',#36780,#36779,#19609,.T.);
#46707=EDGE_CURVE('',#36782,#36783,#19610,.T.);
#46708=EDGE_CURVE('',#36782,#36784,#28292,.T.);
#46709=EDGE_CURVE('',#36784,#36784,#19611,.T.);
#46710=EDGE_CURVE('',#36783,#36782,#19612,.T.);
#46711=EDGE_CURVE('',#36785,#36786,#19613,.T.);
#46712=EDGE_CURVE('',#36785,#36787,#28293,.T.);
#46713=EDGE_CURVE('',#36787,#36787,#19614,.T.);
#46714=EDGE_CURVE('',#36786,#36785,#19615,.T.);
#46715=EDGE_CURVE('',#36788,#36788,#19616,.T.);
#46716=EDGE_CURVE('',#36788,#36789,#28294,.T.);
#46717=EDGE_CURVE('',#36789,#36789,#19617,.T.);
#46718=EDGE_CURVE('',#36790,#36790,#19618,.T.);
#46719=EDGE_CURVE('',#36790,#36791,#28295,.T.);
#46720=EDGE_CURVE('',#36791,#36791,#19619,.T.);
#46721=EDGE_CURVE('',#36792,#36793,#19620,.T.);
#46722=EDGE_CURVE('',#36792,#36794,#28296,.T.);
#46723=EDGE_CURVE('',#36794,#36794,#19621,.T.);
#46724=EDGE_CURVE('',#36793,#36792,#19622,.T.);
#46725=EDGE_CURVE('',#36795,#36795,#19623,.T.);
#46726=EDGE_CURVE('',#36795,#36796,#28297,.T.);
#46727=EDGE_CURVE('',#36796,#36796,#19624,.T.);
#46728=EDGE_CURVE('',#36780,#36790,#28298,.T.);
#46729=EDGE_CURVE('',#36783,#36788,#28299,.T.);
#46730=EDGE_CURVE('',#36797,#36798,#23897,.T.);
#46731=EDGE_CURVE('',#36774,#36797,#23898,.T.);
#46732=EDGE_CURVE('',#36799,#36772,#23899,.T.);
#46733=EDGE_CURVE('',#36800,#36799,#23900,.F.);
#46734=EDGE_CURVE('',#36770,#36800,#23901,.T.);
#46735=EDGE_CURVE('',#36801,#36768,#23902,.T.);
#46736=EDGE_CURVE('',#36802,#36801,#23903,.F.);
#46737=EDGE_CURVE('',#36766,#36802,#23904,.T.);
#46738=EDGE_CURVE('',#36803,#36764,#23905,.T.);
#46739=EDGE_CURVE('',#36804,#36803,#23906,.F.);
#46740=EDGE_CURVE('',#36762,#36804,#23907,.T.);
#46741=EDGE_CURVE('',#36805,#36760,#23908,.T.);
#46742=EDGE_CURVE('',#36806,#36805,#23909,.F.);
#46743=EDGE_CURVE('',#36758,#36806,#23910,.T.);
#46744=EDGE_CURVE('',#36807,#36756,#23911,.T.);
#46745=EDGE_CURVE('',#36808,#36807,#23912,.F.);
#46746=EDGE_CURVE('',#36754,#36808,#23913,.T.);
#46747=EDGE_CURVE('',#36809,#36752,#23914,.T.);
#46748=EDGE_CURVE('',#36810,#36809,#23915,.F.);
#46749=EDGE_CURVE('',#36750,#36810,#23916,.T.);
#46750=EDGE_CURVE('',#36811,#36748,#23917,.T.);
#46751=EDGE_CURVE('',#36812,#36811,#23918,.F.);
#46752=EDGE_CURVE('',#36746,#36812,#23919,.T.);
#46753=EDGE_CURVE('',#36813,#36744,#23920,.T.);
#46754=EDGE_CURVE('',#36814,#36813,#23921,.F.);
#46755=EDGE_CURVE('',#36742,#36814,#23922,.T.);
#46756=EDGE_CURVE('',#36815,#36740,#23923,.T.);
#46757=EDGE_CURVE('',#36816,#36815,#23924,.F.);
#46758=EDGE_CURVE('',#36738,#36816,#23925,.T.);
#46759=EDGE_CURVE('',#36817,#36736,#23926,.T.);
#46760=EDGE_CURVE('',#36818,#36817,#23927,.F.);
#46761=EDGE_CURVE('',#36734,#36818,#23928,.T.);
#46762=EDGE_CURVE('',#36819,#36732,#23929,.T.);
#46763=EDGE_CURVE('',#36820,#36819,#23930,.F.);
#46764=EDGE_CURVE('',#36730,#36820,#23931,.T.);
#46765=EDGE_CURVE('',#36821,#36728,#23932,.T.);
#46766=EDGE_CURVE('',#36822,#36821,#23933,.F.);
#46767=EDGE_CURVE('',#36726,#36822,#23934,.T.);
#46768=EDGE_CURVE('',#36823,#36724,#23935,.T.);
#46769=EDGE_CURVE('',#36824,#36823,#23936,.F.);
#46770=EDGE_CURVE('',#36722,#36824,#23937,.T.);
#46771=EDGE_CURVE('',#36825,#36720,#23938,.T.);
#46772=EDGE_CURVE('',#36826,#36825,#23939,.F.);
#46773=EDGE_CURVE('',#36718,#36826,#23940,.T.);
#46774=EDGE_CURVE('',#36827,#36716,#23941,.T.);
#46775=EDGE_CURVE('',#36828,#36827,#23942,.F.);
#46776=EDGE_CURVE('',#36714,#36828,#23943,.T.);
#46777=EDGE_CURVE('',#36829,#36712,#23944,.T.);
#46778=EDGE_CURVE('',#36830,#36829,#23945,.F.);
#46779=EDGE_CURVE('',#36710,#36830,#23946,.T.);
#46780=EDGE_CURVE('',#36831,#36708,#23947,.T.);
#46781=EDGE_CURVE('',#36832,#36831,#23948,.F.);
#46782=EDGE_CURVE('',#36706,#36832,#23949,.T.);
#46783=EDGE_CURVE('',#36833,#36704,#23950,.T.);
#46784=EDGE_CURVE('',#36834,#36833,#23951,.F.);
#46785=EDGE_CURVE('',#36702,#36834,#23952,.T.);
#46786=EDGE_CURVE('',#36835,#36700,#23953,.T.);
#46787=EDGE_CURVE('',#36836,#36835,#23954,.F.);
#46788=EDGE_CURVE('',#36698,#36836,#23955,.T.);
#46789=EDGE_CURVE('',#36837,#36696,#23956,.T.);
#46790=EDGE_CURVE('',#36838,#36837,#23957,.F.);
#46791=EDGE_CURVE('',#36694,#36838,#23958,.T.);
#46792=EDGE_CURVE('',#36839,#36692,#23959,.T.);
#46793=EDGE_CURVE('',#36840,#36839,#23960,.F.);
#46794=EDGE_CURVE('',#36690,#36840,#23961,.T.);
#46795=EDGE_CURVE('',#36841,#36688,#23962,.T.);
#46796=EDGE_CURVE('',#36842,#36841,#23963,.F.);
#46797=EDGE_CURVE('',#36686,#36842,#23964,.T.);
#46798=EDGE_CURVE('',#36843,#36684,#23965,.T.);
#46799=EDGE_CURVE('',#36844,#36843,#23966,.F.);
#46800=EDGE_CURVE('',#36682,#36844,#23967,.T.);
#46801=EDGE_CURVE('',#36845,#36680,#23968,.T.);
#46802=EDGE_CURVE('',#36846,#36845,#23969,.F.);
#46803=EDGE_CURVE('',#36678,#36846,#23970,.T.);
#46804=EDGE_CURVE('',#36847,#36676,#23971,.T.);
#46805=EDGE_CURVE('',#36848,#36847,#23972,.F.);
#46806=EDGE_CURVE('',#36674,#36848,#23973,.T.);
#46807=EDGE_CURVE('',#36849,#36672,#23974,.T.);
#46808=EDGE_CURVE('',#36850,#36849,#23975,.F.);
#46809=EDGE_CURVE('',#36670,#36850,#23976,.T.);
#46810=EDGE_CURVE('',#36851,#36668,#23977,.T.);
#46811=EDGE_CURVE('',#36852,#36851,#23978,.F.);
#46812=EDGE_CURVE('',#36666,#36852,#23979,.T.);
#46813=EDGE_CURVE('',#36853,#36664,#23980,.T.);
#46814=EDGE_CURVE('',#36854,#36853,#23981,.F.);
#46815=EDGE_CURVE('',#36662,#36854,#23982,.T.);
#46816=EDGE_CURVE('',#36855,#36660,#23983,.T.);
#46817=EDGE_CURVE('',#36856,#36855,#23984,.F.);
#46818=EDGE_CURVE('',#36658,#36856,#23985,.T.);
#46819=EDGE_CURVE('',#36857,#36656,#23986,.T.);
#46820=EDGE_CURVE('',#36858,#36857,#23987,.F.);
#46821=EDGE_CURVE('',#36654,#36858,#23988,.T.);
#46822=EDGE_CURVE('',#36859,#36652,#23989,.T.);
#46823=EDGE_CURVE('',#36860,#36859,#23990,.F.);
#46824=EDGE_CURVE('',#36650,#36860,#23991,.T.);
#46825=EDGE_CURVE('',#36861,#36648,#23992,.T.);
#46826=EDGE_CURVE('',#36862,#36861,#23993,.F.);
#46827=EDGE_CURVE('',#36646,#36862,#23994,.T.);
#46828=EDGE_CURVE('',#36863,#36644,#23995,.T.);
#46829=EDGE_CURVE('',#36864,#36863,#23996,.F.);
#46830=EDGE_CURVE('',#36642,#36864,#23997,.T.);
#46831=EDGE_CURVE('',#36865,#36640,#23998,.T.);
#46832=EDGE_CURVE('',#36866,#36865,#23999,.F.);
#46833=EDGE_CURVE('',#36638,#36866,#24000,.T.);
#46834=EDGE_CURVE('',#36867,#36636,#24001,.T.);
#46835=EDGE_CURVE('',#36868,#36867,#24002,.F.);
#46836=EDGE_CURVE('',#36868,#36869,#28300,.T.);
#46837=EDGE_CURVE('',#36869,#36869,#19625,.T.);
#46838=EDGE_CURVE('',#36870,#36868,#24003,.F.);
#46839=EDGE_CURVE('',#36634,#36870,#24004,.T.);
#46840=EDGE_CURVE('',#36871,#36632,#24005,.T.);
#46841=EDGE_CURVE('',#36872,#36871,#24006,.F.);
#46842=EDGE_CURVE('',#36630,#36872,#24007,.T.);
#46843=EDGE_CURVE('',#36873,#36628,#24008,.T.);
#46844=EDGE_CURVE('',#36874,#36873,#24009,.F.);
#46845=EDGE_CURVE('',#36626,#36874,#24010,.T.);
#46846=EDGE_CURVE('',#36875,#36624,#24011,.T.);
#46847=EDGE_CURVE('',#36876,#36875,#24012,.F.);
#46848=EDGE_CURVE('',#36622,#36876,#24013,.T.);
#46849=EDGE_CURVE('',#36877,#36620,#24014,.T.);
#46850=EDGE_CURVE('',#36878,#36877,#24015,.F.);
#46851=EDGE_CURVE('',#36618,#36878,#24016,.T.);
#46852=EDGE_CURVE('',#36879,#36616,#24017,.T.);
#46853=EDGE_CURVE('',#36880,#36879,#24018,.F.);
#46854=EDGE_CURVE('',#36614,#36880,#24019,.T.);
#46855=EDGE_CURVE('',#36881,#36612,#24020,.T.);
#46856=EDGE_CURVE('',#36882,#36881,#24021,.F.);
#46857=EDGE_CURVE('',#36610,#36882,#24022,.T.);
#46858=EDGE_CURVE('',#36883,#36608,#24023,.T.);
#46859=EDGE_CURVE('',#36884,#36883,#24024,.F.);
#46860=EDGE_CURVE('',#36606,#36884,#24025,.T.);
#46861=EDGE_CURVE('',#36885,#36604,#24026,.T.);
#46862=EDGE_CURVE('',#36886,#36885,#24027,.F.);
#46863=EDGE_CURVE('',#36602,#36886,#24028,.T.);
#46864=EDGE_CURVE('',#36887,#36600,#24029,.T.);
#46865=EDGE_CURVE('',#36888,#36887,#24030,.F.);
#46866=EDGE_CURVE('',#36598,#36888,#24031,.T.);
#46867=EDGE_CURVE('',#36889,#36596,#24032,.T.);
#46868=EDGE_CURVE('',#36890,#36889,#24033,.F.);
#46869=EDGE_CURVE('',#36594,#36890,#24034,.T.);
#46870=EDGE_CURVE('',#36891,#36592,#24035,.T.);
#46871=EDGE_CURVE('',#36892,#36891,#24036,.F.);
#46872=EDGE_CURVE('',#36590,#36892,#24037,.T.);
#46873=EDGE_CURVE('',#36893,#36588,#24038,.T.);
#46874=EDGE_CURVE('',#36894,#36893,#24039,.F.);
#46875=EDGE_CURVE('',#36586,#36894,#24040,.T.);
#46876=EDGE_CURVE('',#36895,#36584,#24041,.T.);
#46877=EDGE_CURVE('',#36896,#36895,#24042,.F.);
#46878=EDGE_CURVE('',#36582,#36896,#24043,.T.);
#46879=EDGE_CURVE('',#36897,#36580,#24044,.T.);
#46880=EDGE_CURVE('',#36898,#36897,#24045,.F.);
#46881=EDGE_CURVE('',#36578,#36898,#24046,.T.);
#46882=EDGE_CURVE('',#36899,#36576,#24047,.T.);
#46883=EDGE_CURVE('',#36900,#36899,#24048,.F.);
#46884=EDGE_CURVE('',#36574,#36900,#24049,.T.);
#46885=EDGE_CURVE('',#36901,#36572,#24050,.T.);
#46886=EDGE_CURVE('',#36902,#36901,#24051,.F.);
#46887=EDGE_CURVE('',#36570,#36902,#24052,.T.);
#46888=EDGE_CURVE('',#36903,#36568,#24053,.T.);
#46889=EDGE_CURVE('',#36904,#36903,#24054,.F.);
#46890=EDGE_CURVE('',#36566,#36904,#24055,.T.);
#46891=EDGE_CURVE('',#36905,#36564,#24056,.T.);
#46892=EDGE_CURVE('',#36906,#36905,#24057,.F.);
#46893=EDGE_CURVE('',#36562,#36906,#24058,.T.);
#46894=EDGE_CURVE('',#36907,#36560,#24059,.T.);
#46895=EDGE_CURVE('',#36908,#36907,#24060,.F.);
#46896=EDGE_CURVE('',#36558,#36908,#24061,.T.);
#46897=EDGE_CURVE('',#36909,#36556,#24062,.T.);
#46898=EDGE_CURVE('',#36910,#36909,#24063,.F.);
#46899=EDGE_CURVE('',#36554,#36910,#24064,.T.);
#46900=EDGE_CURVE('',#36911,#36552,#24065,.T.);
#46901=EDGE_CURVE('',#36912,#36911,#24066,.F.);
#46902=EDGE_CURVE('',#36550,#36912,#24067,.T.);
#46903=EDGE_CURVE('',#36913,#36548,#24068,.T.);
#46904=EDGE_CURVE('',#36914,#36913,#24069,.F.);
#46905=EDGE_CURVE('',#36546,#36914,#24070,.T.);
#46906=EDGE_CURVE('',#36915,#36544,#24071,.T.);
#46907=EDGE_CURVE('',#36916,#36915,#24072,.F.);
#46908=EDGE_CURVE('',#36542,#36916,#24073,.T.);
#46909=EDGE_CURVE('',#36917,#36540,#24074,.T.);
#46910=EDGE_CURVE('',#36918,#36917,#24075,.F.);
#46911=EDGE_CURVE('',#36538,#36918,#24076,.T.);
#46912=EDGE_CURVE('',#36919,#36536,#24077,.T.);
#46913=EDGE_CURVE('',#36920,#36919,#24078,.F.);
#46914=EDGE_CURVE('',#36534,#36920,#24079,.T.);
#46915=EDGE_CURVE('',#36921,#36532,#24080,.T.);
#46916=EDGE_CURVE('',#36922,#36921,#24081,.F.);
#46917=EDGE_CURVE('',#36530,#36922,#24082,.T.);
#46918=EDGE_CURVE('',#36923,#36528,#24083,.T.);
#46919=EDGE_CURVE('',#36924,#36923,#24084,.F.);
#46920=EDGE_CURVE('',#36526,#36924,#24085,.T.);
#46921=EDGE_CURVE('',#36925,#36524,#24086,.T.);
#46922=EDGE_CURVE('',#36926,#36925,#24087,.F.);
#46923=EDGE_CURVE('',#36522,#36926,#24088,.T.);
#46924=EDGE_CURVE('',#36927,#36520,#24089,.T.);
#46925=EDGE_CURVE('',#36928,#36927,#24090,.F.);
#46926=EDGE_CURVE('',#36518,#36928,#24091,.T.);
#46927=EDGE_CURVE('',#36929,#36516,#24092,.T.);
#46928=EDGE_CURVE('',#36930,#36929,#24093,.F.);
#46929=EDGE_CURVE('',#36514,#36930,#24094,.T.);
#46930=EDGE_CURVE('',#36931,#36512,#24095,.T.);
#46931=EDGE_CURVE('',#36932,#36931,#24096,.F.);
#46932=EDGE_CURVE('',#36510,#36932,#24097,.T.);
#46933=EDGE_CURVE('',#36933,#36508,#24098,.T.);
#46934=EDGE_CURVE('',#36934,#36933,#24099,.F.);
#46935=EDGE_CURVE('',#36506,#36934,#24100,.T.);
#46936=EDGE_CURVE('',#36935,#36504,#24101,.T.);
#46937=EDGE_CURVE('',#36936,#36935,#24102,.F.);
#46938=EDGE_CURVE('',#36502,#36936,#24103,.T.);
#46939=EDGE_CURVE('',#36937,#36500,#24104,.T.);
#46940=EDGE_CURVE('',#36938,#36937,#24105,.F.);
#46941=EDGE_CURVE('',#36498,#36938,#24106,.T.);
#46942=EDGE_CURVE('',#36798,#36496,#24107,.T.);
#46943=EDGE_CURVE('',#36786,#36939,#28301,.T.);
#46944=EDGE_CURVE('',#36940,#36939,#24108,.F.);
#46945=EDGE_CURVE('',#36637,#36940,#24109,.T.);
#46946=EDGE_CURVE('',#36941,#36639,#24110,.T.);
#46947=EDGE_CURVE('',#36942,#36941,#24111,.F.);
#46948=EDGE_CURVE('',#36641,#36942,#24112,.T.);
#46949=EDGE_CURVE('',#36943,#36643,#24113,.T.);
#46950=EDGE_CURVE('',#36944,#36943,#24114,.F.);
#46951=EDGE_CURVE('',#36645,#36944,#24115,.T.);
#46952=EDGE_CURVE('',#36945,#36647,#24116,.T.);
#46953=EDGE_CURVE('',#36946,#36945,#24117,.F.);
#46954=EDGE_CURVE('',#36649,#36946,#24118,.T.);
#46955=EDGE_CURVE('',#36947,#36651,#24119,.T.);
#46956=EDGE_CURVE('',#36948,#36947,#24120,.F.);
#46957=EDGE_CURVE('',#36653,#36948,#24121,.T.);
#46958=EDGE_CURVE('',#36949,#36655,#24122,.T.);
#46959=EDGE_CURVE('',#36950,#36949,#24123,.F.);
#46960=EDGE_CURVE('',#36657,#36950,#24124,.T.);
#46961=EDGE_CURVE('',#36951,#36659,#24125,.T.);
#46962=EDGE_CURVE('',#36952,#36951,#24126,.F.);
#46963=EDGE_CURVE('',#36661,#36952,#24127,.T.);
#46964=EDGE_CURVE('',#36953,#36663,#24128,.T.);
#46965=EDGE_CURVE('',#36954,#36953,#24129,.F.);
#46966=EDGE_CURVE('',#36665,#36954,#24130,.T.);
#46967=EDGE_CURVE('',#36955,#36667,#24131,.T.);
#46968=EDGE_CURVE('',#36956,#36955,#24132,.F.);
#46969=EDGE_CURVE('',#36669,#36956,#24133,.T.);
#46970=EDGE_CURVE('',#36957,#36671,#24134,.T.);
#46971=EDGE_CURVE('',#36958,#36957,#24135,.F.);
#46972=EDGE_CURVE('',#36673,#36958,#24136,.T.);
#46973=EDGE_CURVE('',#36959,#36675,#24137,.T.);
#46974=EDGE_CURVE('',#36960,#36959,#24138,.F.);
#46975=EDGE_CURVE('',#36677,#36960,#24139,.T.);
#46976=EDGE_CURVE('',#36961,#36679,#24140,.T.);
#46977=EDGE_CURVE('',#36962,#36961,#24141,.F.);
#46978=EDGE_CURVE('',#36681,#36962,#24142,.T.);
#46979=EDGE_CURVE('',#36963,#36683,#24143,.T.);
#46980=EDGE_CURVE('',#36964,#36963,#24144,.F.);
#46981=EDGE_CURVE('',#36685,#36964,#24145,.T.);
#46982=EDGE_CURVE('',#36965,#36687,#24146,.T.);
#46983=EDGE_CURVE('',#36966,#36965,#24147,.F.);
#46984=EDGE_CURVE('',#36689,#36966,#24148,.T.);
#46985=EDGE_CURVE('',#36967,#36691,#24149,.T.);
#46986=EDGE_CURVE('',#36968,#36967,#24150,.F.);
#46987=EDGE_CURVE('',#36693,#36968,#24151,.T.);
#46988=EDGE_CURVE('',#36969,#36695,#24152,.T.);
#46989=EDGE_CURVE('',#36970,#36969,#24153,.F.);
#46990=EDGE_CURVE('',#36697,#36970,#24154,.T.);
#46991=EDGE_CURVE('',#36971,#36699,#24155,.T.);
#46992=EDGE_CURVE('',#36972,#36971,#24156,.F.);
#46993=EDGE_CURVE('',#36701,#36972,#24157,.T.);
#46994=EDGE_CURVE('',#36973,#36703,#24158,.T.);
#46995=EDGE_CURVE('',#36974,#36973,#24159,.F.);
#46996=EDGE_CURVE('',#36705,#36974,#24160,.T.);
#46997=EDGE_CURVE('',#36975,#36707,#24161,.T.);
#46998=EDGE_CURVE('',#36976,#36975,#24162,.F.);
#46999=EDGE_CURVE('',#36709,#36976,#24163,.T.);
#47000=EDGE_CURVE('',#36977,#36711,#24164,.T.);
#47001=EDGE_CURVE('',#36978,#36977,#24165,.F.);
#47002=EDGE_CURVE('',#36713,#36978,#24166,.T.);
#47003=EDGE_CURVE('',#36979,#36715,#24167,.T.);
#47004=EDGE_CURVE('',#36980,#36979,#24168,.F.);
#47005=EDGE_CURVE('',#36717,#36980,#24169,.T.);
#47006=EDGE_CURVE('',#36981,#36719,#24170,.T.);
#47007=EDGE_CURVE('',#36982,#36981,#24171,.F.);
#47008=EDGE_CURVE('',#36721,#36982,#24172,.T.);
#47009=EDGE_CURVE('',#36983,#36723,#24173,.T.);
#47010=EDGE_CURVE('',#36984,#36983,#24174,.F.);
#47011=EDGE_CURVE('',#36725,#36984,#24175,.T.);
#47012=EDGE_CURVE('',#36985,#36727,#24176,.T.);
#47013=EDGE_CURVE('',#36986,#36985,#24177,.F.);
#47014=EDGE_CURVE('',#36729,#36986,#24178,.T.);
#47015=EDGE_CURVE('',#36987,#36731,#24179,.T.);
#47016=EDGE_CURVE('',#36988,#36987,#24180,.F.);
#47017=EDGE_CURVE('',#36733,#36988,#24181,.T.);
#47018=EDGE_CURVE('',#36989,#36735,#24182,.T.);
#47019=EDGE_CURVE('',#36990,#36989,#24183,.F.);
#47020=EDGE_CURVE('',#36737,#36990,#24184,.T.);
#47021=EDGE_CURVE('',#36991,#36739,#24185,.T.);
#47022=EDGE_CURVE('',#36992,#36991,#24186,.F.);
#47023=EDGE_CURVE('',#36741,#36992,#24187,.T.);
#47024=EDGE_CURVE('',#36993,#36743,#24188,.T.);
#47025=EDGE_CURVE('',#36994,#36993,#24189,.F.);
#47026=EDGE_CURVE('',#36745,#36994,#24190,.T.);
#47027=EDGE_CURVE('',#36995,#36747,#24191,.T.);
#47028=EDGE_CURVE('',#36996,#36995,#24192,.F.);
#47029=EDGE_CURVE('',#36749,#36996,#24193,.T.);
#47030=EDGE_CURVE('',#36997,#36751,#24194,.T.);
#47031=EDGE_CURVE('',#36998,#36997,#24195,.F.);
#47032=EDGE_CURVE('',#36753,#36998,#24196,.T.);
#47033=EDGE_CURVE('',#36999,#36755,#24197,.T.);
#47034=EDGE_CURVE('',#37000,#36999,#24198,.F.);
#47035=EDGE_CURVE('',#36757,#37000,#24199,.T.);
#47036=EDGE_CURVE('',#37001,#36759,#24200,.T.);
#47037=EDGE_CURVE('',#37002,#37001,#24201,.F.);
#47038=EDGE_CURVE('',#36761,#37002,#24202,.T.);
#47039=EDGE_CURVE('',#37003,#36763,#24203,.T.);
#47040=EDGE_CURVE('',#37004,#37003,#24204,.F.);
#47041=EDGE_CURVE('',#36765,#37004,#24205,.T.);
#47042=EDGE_CURVE('',#37005,#36767,#24206,.T.);
#47043=EDGE_CURVE('',#37006,#37005,#24207,.F.);
#47044=EDGE_CURVE('',#36769,#37006,#24208,.T.);
#47045=EDGE_CURVE('',#37007,#36771,#24209,.T.);
#47046=EDGE_CURVE('',#37008,#37007,#24210,.F.);
#47047=EDGE_CURVE('',#36773,#37008,#24211,.T.);
#47048=EDGE_CURVE('',#37009,#36775,#24212,.T.);
#47049=EDGE_CURVE('',#37010,#37009,#24213,.T.);
#47050=EDGE_CURVE('',#36497,#37010,#24214,.T.);
#47051=EDGE_CURVE('',#37011,#36499,#24215,.T.);
#47052=EDGE_CURVE('',#37012,#37011,#24216,.F.);
#47053=EDGE_CURVE('',#36501,#37012,#24217,.T.);
#47054=EDGE_CURVE('',#37013,#36503,#24218,.T.);
#47055=EDGE_CURVE('',#37014,#37013,#24219,.F.);
#47056=EDGE_CURVE('',#36505,#37014,#24220,.T.);
#47057=EDGE_CURVE('',#37015,#36507,#24221,.T.);
#47058=EDGE_CURVE('',#37016,#37015,#24222,.F.);
#47059=EDGE_CURVE('',#36509,#37016,#24223,.T.);
#47060=EDGE_CURVE('',#37017,#36511,#24224,.T.);
#47061=EDGE_CURVE('',#37018,#37017,#24225,.F.);
#47062=EDGE_CURVE('',#36513,#37018,#24226,.T.);
#47063=EDGE_CURVE('',#37019,#36515,#24227,.T.);
#47064=EDGE_CURVE('',#37020,#37019,#24228,.F.);
#47065=EDGE_CURVE('',#36517,#37020,#24229,.T.);
#47066=EDGE_CURVE('',#37021,#36519,#24230,.T.);
#47067=EDGE_CURVE('',#37022,#37021,#24231,.F.);
#47068=EDGE_CURVE('',#36521,#37022,#24232,.T.);
#47069=EDGE_CURVE('',#37023,#36523,#24233,.T.);
#47070=EDGE_CURVE('',#37024,#37023,#24234,.F.);
#47071=EDGE_CURVE('',#36525,#37024,#24235,.T.);
#47072=EDGE_CURVE('',#37025,#36527,#24236,.T.);
#47073=EDGE_CURVE('',#37026,#37025,#24237,.F.);
#47074=EDGE_CURVE('',#36529,#37026,#24238,.T.);
#47075=EDGE_CURVE('',#37027,#36531,#24239,.T.);
#47076=EDGE_CURVE('',#37028,#37027,#24240,.F.);
#47077=EDGE_CURVE('',#36533,#37028,#24241,.T.);
#47078=EDGE_CURVE('',#37029,#36535,#24242,.T.);
#47079=EDGE_CURVE('',#37030,#37029,#24243,.F.);
#47080=EDGE_CURVE('',#36537,#37030,#24244,.T.);
#47081=EDGE_CURVE('',#37031,#36539,#24245,.T.);
#47082=EDGE_CURVE('',#37032,#37031,#24246,.F.);
#47083=EDGE_CURVE('',#36541,#37032,#24247,.T.);
#47084=EDGE_CURVE('',#37033,#36543,#24248,.T.);
#47085=EDGE_CURVE('',#37034,#37033,#24249,.F.);
#47086=EDGE_CURVE('',#36545,#37034,#24250,.T.);
#47087=EDGE_CURVE('',#37035,#36547,#24251,.T.);
#47088=EDGE_CURVE('',#37036,#37035,#24252,.F.);
#47089=EDGE_CURVE('',#36549,#37036,#24253,.T.);
#47090=EDGE_CURVE('',#37037,#36551,#24254,.T.);
#47091=EDGE_CURVE('',#37038,#37037,#24255,.F.);
#47092=EDGE_CURVE('',#36553,#37038,#24256,.T.);
#47093=EDGE_CURVE('',#37039,#36555,#24257,.T.);
#47094=EDGE_CURVE('',#37040,#37039,#24258,.F.);
#47095=EDGE_CURVE('',#36557,#37040,#24259,.T.);
#47096=EDGE_CURVE('',#37041,#36559,#24260,.T.);
#47097=EDGE_CURVE('',#37042,#37041,#24261,.F.);
#47098=EDGE_CURVE('',#36561,#37042,#24262,.T.);
#47099=EDGE_CURVE('',#37043,#36563,#24263,.T.);
#47100=EDGE_CURVE('',#37044,#37043,#24264,.F.);
#47101=EDGE_CURVE('',#36565,#37044,#24265,.T.);
#47102=EDGE_CURVE('',#37045,#36567,#24266,.T.);
#47103=EDGE_CURVE('',#37046,#37045,#24267,.F.);
#47104=EDGE_CURVE('',#36569,#37046,#24268,.T.);
#47105=EDGE_CURVE('',#37047,#36571,#24269,.T.);
#47106=EDGE_CURVE('',#37048,#37047,#24270,.F.);
#47107=EDGE_CURVE('',#36573,#37048,#24271,.T.);
#47108=EDGE_CURVE('',#37049,#36575,#24272,.T.);
#47109=EDGE_CURVE('',#37050,#37049,#24273,.F.);
#47110=EDGE_CURVE('',#36577,#37050,#24274,.T.);
#47111=EDGE_CURVE('',#37051,#36579,#24275,.T.);
#47112=EDGE_CURVE('',#37052,#37051,#24276,.F.);
#47113=EDGE_CURVE('',#36581,#37052,#24277,.T.);
#47114=EDGE_CURVE('',#37053,#36583,#24278,.T.);
#47115=EDGE_CURVE('',#37054,#37053,#24279,.F.);
#47116=EDGE_CURVE('',#36585,#37054,#24280,.T.);
#47117=EDGE_CURVE('',#37055,#36587,#24281,.T.);
#47118=EDGE_CURVE('',#37056,#37055,#24282,.F.);
#47119=EDGE_CURVE('',#36589,#37056,#24283,.T.);
#47120=EDGE_CURVE('',#37057,#36591,#24284,.T.);
#47121=EDGE_CURVE('',#37058,#37057,#24285,.F.);
#47122=EDGE_CURVE('',#36593,#37058,#24286,.T.);
#47123=EDGE_CURVE('',#37059,#36595,#24287,.T.);
#47124=EDGE_CURVE('',#37060,#37059,#24288,.F.);
#47125=EDGE_CURVE('',#36597,#37060,#24289,.T.);
#47126=EDGE_CURVE('',#37061,#36599,#24290,.T.);
#47127=EDGE_CURVE('',#37062,#37061,#24291,.F.);
#47128=EDGE_CURVE('',#36601,#37062,#24292,.T.);
#47129=EDGE_CURVE('',#37063,#36603,#24293,.T.);
#47130=EDGE_CURVE('',#37064,#37063,#24294,.F.);
#47131=EDGE_CURVE('',#36605,#37064,#24295,.T.);
#47132=EDGE_CURVE('',#37065,#36607,#24296,.T.);
#47133=EDGE_CURVE('',#37066,#37065,#24297,.F.);
#47134=EDGE_CURVE('',#36609,#37066,#24298,.T.);
#47135=EDGE_CURVE('',#37067,#36611,#24299,.T.);
#47136=EDGE_CURVE('',#37068,#37067,#24300,.F.);
#47137=EDGE_CURVE('',#36613,#37068,#24301,.T.);
#47138=EDGE_CURVE('',#37069,#36615,#24302,.T.);
#47139=EDGE_CURVE('',#37070,#37069,#24303,.F.);
#47140=EDGE_CURVE('',#36617,#37070,#24304,.T.);
#47141=EDGE_CURVE('',#37071,#36619,#24305,.T.);
#47142=EDGE_CURVE('',#37072,#37071,#24306,.F.);
#47143=EDGE_CURVE('',#36621,#37072,#24307,.T.);
#47144=EDGE_CURVE('',#37073,#36623,#24308,.T.);
#47145=EDGE_CURVE('',#37074,#37073,#24309,.F.);
#47146=EDGE_CURVE('',#36625,#37074,#24310,.T.);
#47147=EDGE_CURVE('',#37075,#36627,#24311,.T.);
#47148=EDGE_CURVE('',#37076,#37075,#24312,.F.);
#47149=EDGE_CURVE('',#36629,#37076,#24313,.T.);
#47150=EDGE_CURVE('',#37077,#36631,#24314,.T.);
#47151=EDGE_CURVE('',#37078,#37077,#24315,.F.);
#47152=EDGE_CURVE('',#36633,#37078,#24316,.T.);
#47153=EDGE_CURVE('',#37079,#36635,#24317,.T.);
#47154=EDGE_CURVE('',#36939,#37079,#24318,.F.);
#47155=EDGE_CURVE('',#36793,#37080,#28302,.T.);
#47156=EDGE_CURVE('',#37080,#37080,#19626,.T.);
#47157=EDGE_CURVE('',#36777,#36795,#28303,.T.);
#47158=EDGE_CURVE('',#36797,#37009,#19627,.T.);
#47159=EDGE_CURVE('',#36798,#37010,#19628,.T.);
#47160=EDGE_CURVE('',#36938,#37011,#19629,.T.);
#47161=EDGE_CURVE('',#36937,#37012,#19630,.T.);
#47162=EDGE_CURVE('',#36936,#37013,#19631,.T.);
#47163=EDGE_CURVE('',#36935,#37014,#19632,.T.);
#47164=EDGE_CURVE('',#36934,#37015,#19633,.T.);
#47165=EDGE_CURVE('',#36933,#37016,#19634,.T.);
#47166=EDGE_CURVE('',#36932,#37017,#19635,.T.);
#47167=EDGE_CURVE('',#36931,#37018,#19636,.T.);
#47168=EDGE_CURVE('',#36930,#37019,#19637,.T.);
#47169=EDGE_CURVE('',#36929,#37020,#19638,.T.);
#47170=EDGE_CURVE('',#36928,#37021,#19639,.T.);
#47171=EDGE_CURVE('',#36927,#37022,#19640,.T.);
#47172=EDGE_CURVE('',#36926,#37023,#19641,.T.);
#47173=EDGE_CURVE('',#36925,#37024,#19642,.T.);
#47174=EDGE_CURVE('',#36924,#37025,#19643,.T.);
#47175=EDGE_CURVE('',#36923,#37026,#19644,.T.);
#47176=EDGE_CURVE('',#36922,#37027,#19645,.T.);
#47177=EDGE_CURVE('',#36921,#37028,#19646,.T.);
#47178=EDGE_CURVE('',#36920,#37029,#19647,.T.);
#47179=EDGE_CURVE('',#36919,#37030,#19648,.T.);
#47180=EDGE_CURVE('',#36918,#37031,#19649,.T.);
#47181=EDGE_CURVE('',#36917,#37032,#19650,.T.);
#47182=EDGE_CURVE('',#36916,#37033,#19651,.T.);
#47183=EDGE_CURVE('',#36915,#37034,#19652,.T.);
#47184=EDGE_CURVE('',#36914,#37035,#19653,.T.);
#47185=EDGE_CURVE('',#36913,#37036,#19654,.T.);
#47186=EDGE_CURVE('',#36912,#37037,#19655,.T.);
#47187=EDGE_CURVE('',#36911,#37038,#19656,.T.);
#47188=EDGE_CURVE('',#36910,#37039,#19657,.T.);
#47189=EDGE_CURVE('',#36909,#37040,#19658,.T.);
#47190=EDGE_CURVE('',#36908,#37041,#19659,.T.);
#47191=EDGE_CURVE('',#36907,#37042,#19660,.T.);
#47192=EDGE_CURVE('',#36906,#37043,#19661,.T.);
#47193=EDGE_CURVE('',#36905,#37044,#19662,.T.);
#47194=EDGE_CURVE('',#36904,#37045,#19663,.T.);
#47195=EDGE_CURVE('',#36903,#37046,#19664,.T.);
#47196=EDGE_CURVE('',#36902,#37047,#19665,.T.);
#47197=EDGE_CURVE('',#36901,#37048,#19666,.T.);
#47198=EDGE_CURVE('',#36900,#37049,#19667,.T.);
#47199=EDGE_CURVE('',#36899,#37050,#19668,.T.);
#47200=EDGE_CURVE('',#36898,#37051,#19669,.T.);
#47201=EDGE_CURVE('',#36897,#37052,#19670,.T.);
#47202=EDGE_CURVE('',#36896,#37053,#19671,.T.);
#47203=EDGE_CURVE('',#36895,#37054,#19672,.T.);
#47204=EDGE_CURVE('',#36894,#37055,#19673,.T.);
#47205=EDGE_CURVE('',#36893,#37056,#19674,.T.);
#47206=EDGE_CURVE('',#36892,#37057,#19675,.T.);
#47207=EDGE_CURVE('',#36891,#37058,#19676,.T.);
#47208=EDGE_CURVE('',#36890,#37059,#19677,.T.);
#47209=EDGE_CURVE('',#36889,#37060,#19678,.T.);
#47210=EDGE_CURVE('',#36888,#37061,#19679,.T.);
#47211=EDGE_CURVE('',#36887,#37062,#19680,.T.);
#47212=EDGE_CURVE('',#36886,#37063,#19681,.T.);
#47213=EDGE_CURVE('',#36885,#37064,#19682,.T.);
#47214=EDGE_CURVE('',#36884,#37065,#19683,.T.);
#47215=EDGE_CURVE('',#36883,#37066,#19684,.T.);
#47216=EDGE_CURVE('',#36882,#37067,#19685,.T.);
#47217=EDGE_CURVE('',#36881,#37068,#19686,.T.);
#47218=EDGE_CURVE('',#36880,#37069,#19687,.T.);
#47219=EDGE_CURVE('',#36879,#37070,#19688,.T.);
#47220=EDGE_CURVE('',#36878,#37071,#19689,.T.);
#47221=EDGE_CURVE('',#36877,#37072,#19690,.T.);
#47222=EDGE_CURVE('',#36876,#37073,#19691,.T.);
#47223=EDGE_CURVE('',#36875,#37074,#19692,.T.);
#47224=EDGE_CURVE('',#36874,#37075,#19693,.T.);
#47225=EDGE_CURVE('',#36873,#37076,#19694,.T.);
#47226=EDGE_CURVE('',#36872,#37077,#19695,.T.);
#47227=EDGE_CURVE('',#36871,#37078,#19696,.T.);
#47228=EDGE_CURVE('',#36870,#37079,#19697,.T.);
#47229=EDGE_CURVE('',#36867,#36940,#19698,.T.);
#47230=EDGE_CURVE('',#36866,#36941,#19699,.T.);
#47231=EDGE_CURVE('',#36865,#36942,#19700,.T.);
#47232=EDGE_CURVE('',#36864,#36943,#19701,.T.);
#47233=EDGE_CURVE('',#36863,#36944,#19702,.T.);
#47234=EDGE_CURVE('',#36862,#36945,#19703,.T.);
#47235=EDGE_CURVE('',#36861,#36946,#19704,.T.);
#47236=EDGE_CURVE('',#36860,#36947,#19705,.T.);
#47237=EDGE_CURVE('',#36859,#36948,#19706,.T.);
#47238=EDGE_CURVE('',#36858,#36949,#19707,.T.);
#47239=EDGE_CURVE('',#36857,#36950,#19708,.T.);
#47240=EDGE_CURVE('',#36856,#36951,#19709,.T.);
#47241=EDGE_CURVE('',#36855,#36952,#19710,.T.);
#47242=EDGE_CURVE('',#36854,#36953,#19711,.T.);
#47243=EDGE_CURVE('',#36853,#36954,#19712,.T.);
#47244=EDGE_CURVE('',#36852,#36955,#19713,.T.);
#47245=EDGE_CURVE('',#36851,#36956,#19714,.T.);
#47246=EDGE_CURVE('',#36850,#36957,#19715,.T.);
#47247=EDGE_CURVE('',#36849,#36958,#19716,.T.);
#47248=EDGE_CURVE('',#36848,#36959,#19717,.T.);
#47249=EDGE_CURVE('',#36847,#36960,#19718,.T.);
#47250=EDGE_CURVE('',#36846,#36961,#19719,.T.);
#47251=EDGE_CURVE('',#36845,#36962,#19720,.T.);
#47252=EDGE_CURVE('',#36844,#36963,#19721,.T.);
#47253=EDGE_CURVE('',#36843,#36964,#19722,.T.);
#47254=EDGE_CURVE('',#36842,#36965,#19723,.T.);
#47255=EDGE_CURVE('',#36841,#36966,#19724,.T.);
#47256=EDGE_CURVE('',#36840,#36967,#19725,.T.);
#47257=EDGE_CURVE('',#36839,#36968,#19726,.T.);
#47258=EDGE_CURVE('',#36838,#36969,#19727,.T.);
#47259=EDGE_CURVE('',#36837,#36970,#19728,.T.);
#47260=EDGE_CURVE('',#36836,#36971,#19729,.T.);
#47261=EDGE_CURVE('',#36835,#36972,#19730,.T.);
#47262=EDGE_CURVE('',#36834,#36973,#19731,.T.);
#47263=EDGE_CURVE('',#36833,#36974,#19732,.T.);
#47264=EDGE_CURVE('',#36832,#36975,#19733,.T.);
#47265=EDGE_CURVE('',#36831,#36976,#19734,.T.);
#47266=EDGE_CURVE('',#36830,#36977,#19735,.T.);
#47267=EDGE_CURVE('',#36829,#36978,#19736,.T.);
#47268=EDGE_CURVE('',#36828,#36979,#19737,.T.);
#47269=EDGE_CURVE('',#36827,#36980,#19738,.T.);
#47270=EDGE_CURVE('',#36826,#36981,#19739,.T.);
#47271=EDGE_CURVE('',#36825,#36982,#19740,.T.);
#47272=EDGE_CURVE('',#36824,#36983,#19741,.T.);
#47273=EDGE_CURVE('',#36823,#36984,#19742,.T.);
#47274=EDGE_CURVE('',#36822,#36985,#19743,.T.);
#47275=EDGE_CURVE('',#36821,#36986,#19744,.T.);
#47276=EDGE_CURVE('',#36820,#36987,#19745,.T.);
#47277=EDGE_CURVE('',#36819,#36988,#19746,.T.);
#47278=EDGE_CURVE('',#36818,#36989,#19747,.T.);
#47279=EDGE_CURVE('',#36817,#36990,#19748,.T.);
#47280=EDGE_CURVE('',#36816,#36991,#19749,.T.);
#47281=EDGE_CURVE('',#36815,#36992,#19750,.T.);
#47282=EDGE_CURVE('',#36814,#36993,#19751,.T.);
#47283=EDGE_CURVE('',#36813,#36994,#19752,.T.);
#47284=EDGE_CURVE('',#36812,#36995,#19753,.T.);
#47285=EDGE_CURVE('',#36811,#36996,#19754,.T.);
#47286=EDGE_CURVE('',#36810,#36997,#19755,.T.);
#47287=EDGE_CURVE('',#36809,#36998,#19756,.T.);
#47288=EDGE_CURVE('',#36808,#36999,#19757,.T.);
#47289=EDGE_CURVE('',#36807,#37000,#19758,.T.);
#47290=EDGE_CURVE('',#36806,#37001,#19759,.T.);
#47291=EDGE_CURVE('',#36805,#37002,#19760,.T.);
#47292=EDGE_CURVE('',#36804,#37003,#19761,.T.);
#47293=EDGE_CURVE('',#36803,#37004,#19762,.T.);
#47294=EDGE_CURVE('',#36802,#37005,#19763,.T.);
#47295=EDGE_CURVE('',#36801,#37006,#19764,.T.);
#47296=EDGE_CURVE('',#36800,#37007,#19765,.T.);
#47297=EDGE_CURVE('',#36799,#37008,#19766,.T.);
#47298=EDGE_CURVE('',#37081,#37081,#19767,.T.);
#47299=EDGE_CURVE('',#37081,#37082,#28304,.T.);
#47300=EDGE_CURVE('',#37082,#37082,#19768,.T.);
#47301=EDGE_CURVE('',#37083,#37083,#19769,.T.);
#47302=EDGE_CURVE('',#37083,#37084,#28305,.T.);
#47303=EDGE_CURVE('',#37084,#37084,#19770,.T.);
#47304=EDGE_CURVE('',#37085,#37085,#19771,.T.);
#47305=EDGE_CURVE('',#37085,#37086,#19772,.T.);
#47306=EDGE_CURVE('',#37086,#37086,#19773,.T.);
#47307=EDGE_CURVE('',#37087,#37087,#19774,.T.);
#47308=EDGE_CURVE('',#37087,#37088,#19775,.T.);
#47309=EDGE_CURVE('',#37088,#37088,#19776,.T.);
#47310=EDGE_CURVE('',#37089,#37090,#19777,.T.);
#47311=EDGE_CURVE('',#37089,#37091,#19778,.T.);
#47312=EDGE_CURVE('',#37091,#37091,#19779,.T.);
#47313=EDGE_CURVE('',#37090,#37089,#19780,.T.);
#47314=EDGE_CURVE('',#37092,#37092,#19781,.T.);
#47315=EDGE_CURVE('',#37092,#37093,#19782,.T.);
#47316=EDGE_CURVE('',#37093,#37093,#19783,.T.);
#47317=EDGE_CURVE('',#37094,#37094,#19784,.T.);
#47318=EDGE_CURVE('',#37094,#37095,#19785,.T.);
#47319=EDGE_CURVE('',#37096,#37095,#19786,.T.);
#47320=EDGE_CURVE('',#37095,#37096,#19787,.T.);
#47321=EDGE_CURVE('',#37097,#37098,#19788,.T.);
#47322=EDGE_CURVE('',#37097,#37099,#19789,.T.);
#47323=EDGE_CURVE('',#37100,#37099,#19790,.T.);
#47324=EDGE_CURVE('',#37098,#37100,#19791,.T.);
#47325=EDGE_CURVE('',#37101,#37102,#19792,.T.);
#47326=EDGE_CURVE('',#37101,#37103,#19793,.T.);
#47327=EDGE_CURVE('',#37104,#37103,#19794,.T.);
#47328=EDGE_CURVE('',#37102,#37104,#19795,.T.);
#47329=EDGE_CURVE('',#37105,#37105,#19796,.T.);
#47330=EDGE_CURVE('',#37105,#37106,#19797,.T.);
#47331=EDGE_CURVE('',#37107,#37106,#19798,.T.);
#47332=EDGE_CURVE('',#37106,#37107,#19799,.T.);
#47333=EDGE_CURVE('',#37108,#37108,#19800,.T.);
#47334=EDGE_CURVE('',#37108,#37109,#19801,.T.);
#47335=EDGE_CURVE('',#37110,#37109,#19802,.T.);
#47336=EDGE_CURVE('',#37109,#37110,#19803,.T.);
#47337=EDGE_CURVE('',#37111,#37111,#19804,.T.);
#47338=EDGE_CURVE('',#37111,#37112,#19805,.T.);
#47339=EDGE_CURVE('',#37113,#37112,#19806,.T.);
#47340=EDGE_CURVE('',#37112,#37113,#19807,.T.);
#47341=EDGE_CURVE('',#37114,#37115,#19808,.T.);
#47342=EDGE_CURVE('',#37116,#37115,#28306,.T.);
#47343=EDGE_CURVE('',#37116,#37117,#19809,.T.);
#47344=EDGE_CURVE('',#37117,#37114,#28307,.T.);
#47345=EDGE_CURVE('',#37118,#37119,#19810,.T.);
#47346=EDGE_CURVE('',#37120,#37119,#28308,.T.);
#47347=EDGE_CURVE('',#37120,#37121,#19811,.T.);
#47348=EDGE_CURVE('',#37121,#37118,#28309,.T.);
#47349=EDGE_CURVE('',#37122,#37122,#19812,.T.);
#47350=EDGE_CURVE('',#37122,#37107,#28310,.T.);
#47351=EDGE_CURVE('',#37086,#37110,#28311,.T.);
#47352=EDGE_CURVE('',#37088,#37113,#28312,.T.);
#47353=EDGE_CURVE('',#37123,#37123,#19813,.T.);
#47354=EDGE_CURVE('',#37123,#37096,#28313,.T.);
#47355=EDGE_CURVE('',#37124,#37125,#19814,.T.);
#47356=EDGE_CURVE('',#37125,#37126,#28314,.T.);
#47357=EDGE_CURVE('',#37127,#37126,#19815,.T.);
#47358=EDGE_CURVE('',#37124,#37127,#28315,.T.);
#47359=EDGE_CURVE('',#37128,#37129,#19816,.T.);
#47360=EDGE_CURVE('',#37129,#37130,#28316,.T.);
#47361=EDGE_CURVE('',#37131,#37130,#19817,.T.);
#47362=EDGE_CURVE('',#37128,#37131,#28317,.T.);
#47363=EDGE_CURVE('',#37132,#37133,#19818,.T.);
#47364=EDGE_CURVE('',#37133,#37134,#28318,.T.);
#47365=EDGE_CURVE('',#37134,#37135,#19819,.T.);
#47366=EDGE_CURVE('',#37135,#37132,#28319,.T.);
#47367=EDGE_CURVE('',#37136,#37137,#19820,.T.);
#47368=EDGE_CURVE('',#37137,#37138,#28320,.T.);
#47369=EDGE_CURVE('',#37138,#37139,#19821,.T.);
#47370=EDGE_CURVE('',#37139,#37136,#28321,.T.);
#47371=EDGE_CURVE('',#37090,#37092,#28322,.T.);
#47372=EDGE_CURVE('',#37140,#37141,#19822,.T.);
#47373=EDGE_CURVE('',#37142,#37140,#19823,.T.);
#47374=EDGE_CURVE('',#37143,#37142,#19824,.T.);
#47375=EDGE_CURVE('',#37144,#37143,#19825,.T.);
#47376=EDGE_CURVE('',#37145,#37144,#19826,.T.);
#47377=EDGE_CURVE('',#37146,#37145,#19827,.T.);
#47378=EDGE_CURVE('',#37147,#37146,#19828,.T.);
#47379=EDGE_CURVE('',#37148,#37147,#19829,.T.);
#47380=EDGE_CURVE('',#37149,#37148,#19830,.T.);
#47381=EDGE_CURVE('',#37150,#37149,#19831,.T.);
#47382=EDGE_CURVE('',#37151,#37150,#19832,.T.);
#47383=EDGE_CURVE('',#37152,#37151,#19833,.T.);
#47384=EDGE_CURVE('',#37153,#37152,#19834,.T.);
#47385=EDGE_CURVE('',#37154,#37153,#19835,.T.);
#47386=EDGE_CURVE('',#37155,#37154,#19836,.T.);
#47387=EDGE_CURVE('',#37156,#37155,#19837,.T.);
#47388=EDGE_CURVE('',#37157,#37156,#19838,.T.);
#47389=EDGE_CURVE('',#37158,#37157,#19839,.T.);
#47390=EDGE_CURVE('',#37159,#37158,#19840,.T.);
#47391=EDGE_CURVE('',#37160,#37159,#19841,.T.);
#47392=EDGE_CURVE('',#37161,#37160,#19842,.T.);
#47393=EDGE_CURVE('',#37162,#37161,#19843,.T.);
#47394=EDGE_CURVE('',#37163,#37162,#19844,.T.);
#47395=EDGE_CURVE('',#37164,#37163,#19845,.T.);
#47396=EDGE_CURVE('',#37165,#37164,#19846,.T.);
#47397=EDGE_CURVE('',#37166,#37165,#19847,.T.);
#47398=EDGE_CURVE('',#37167,#37166,#19848,.T.);
#47399=EDGE_CURVE('',#37168,#37167,#19849,.T.);
#47400=EDGE_CURVE('',#37169,#37168,#19850,.T.);
#47401=EDGE_CURVE('',#37133,#37169,#19851,.T.);
#47402=EDGE_CURVE('',#37170,#37132,#19852,.T.);
#47403=EDGE_CURVE('',#37171,#37170,#19853,.T.);
#47404=EDGE_CURVE('',#37137,#37171,#19854,.T.);
#47405=EDGE_CURVE('',#37172,#37136,#19855,.T.);
#47406=EDGE_CURVE('',#37173,#37172,#19856,.T.);
#47407=EDGE_CURVE('',#37174,#37173,#19857,.T.);
#47408=EDGE_CURVE('',#37175,#37174,#19858,.T.);
#47409=EDGE_CURVE('',#37176,#37175,#19859,.T.);
#47410=EDGE_CURVE('',#37177,#37176,#19860,.T.);
#47411=EDGE_CURVE('',#37178,#37177,#19861,.T.);
#47412=EDGE_CURVE('',#37179,#37178,#19862,.T.);
#47413=EDGE_CURVE('',#37180,#37179,#19863,.T.);
#47414=EDGE_CURVE('',#37181,#37180,#19864,.T.);
#47415=EDGE_CURVE('',#37182,#37181,#19865,.T.);
#47416=EDGE_CURVE('',#37183,#37182,#19866,.T.);
#47417=EDGE_CURVE('',#37184,#37183,#19867,.T.);
#47418=EDGE_CURVE('',#37185,#37184,#19868,.T.);
#47419=EDGE_CURVE('',#37186,#37185,#19869,.T.);
#47420=EDGE_CURVE('',#37187,#37186,#19870,.T.);
#47421=EDGE_CURVE('',#37188,#37187,#19871,.T.);
#47422=EDGE_CURVE('',#37189,#37188,#19872,.T.);
#47423=EDGE_CURVE('',#37190,#37189,#19873,.T.);
#47424=EDGE_CURVE('',#37191,#37190,#19874,.T.);
#47425=EDGE_CURVE('',#37192,#37191,#19875,.T.);
#47426=EDGE_CURVE('',#37193,#37192,#19876,.T.);
#47427=EDGE_CURVE('',#37194,#37193,#19877,.T.);
#47428=EDGE_CURVE('',#37195,#37194,#19878,.T.);
#47429=EDGE_CURVE('',#37196,#37195,#19879,.T.);
#47430=EDGE_CURVE('',#37197,#37196,#19880,.T.);
#47431=EDGE_CURVE('',#37198,#37197,#19881,.T.);
#47432=EDGE_CURVE('',#37199,#37198,#19882,.T.);
#47433=EDGE_CURVE('',#37200,#37199,#19883,.T.);
#47434=EDGE_CURVE('',#37201,#37200,#19884,.T.);
#47435=EDGE_CURVE('',#37202,#37201,#19885,.T.);
#47436=EDGE_CURVE('',#37203,#37202,#19886,.T.);
#47437=EDGE_CURVE('',#37204,#37203,#19887,.T.);
#47438=EDGE_CURVE('',#37205,#37204,#19888,.T.);
#47439=EDGE_CURVE('',#37206,#37205,#19889,.T.);
#47440=EDGE_CURVE('',#37207,#37206,#19890,.T.);
#47441=EDGE_CURVE('',#37208,#37207,#19891,.T.);
#47442=EDGE_CURVE('',#37209,#37208,#19892,.T.);
#47443=EDGE_CURVE('',#37210,#37209,#19893,.T.);
#47444=EDGE_CURVE('',#37211,#37210,#19894,.T.);
#47445=EDGE_CURVE('',#37212,#37211,#19895,.T.);
#47446=EDGE_CURVE('',#37213,#37212,#19896,.T.);
#47447=EDGE_CURVE('',#37214,#37213,#19897,.T.);
#47448=EDGE_CURVE('',#37215,#37214,#19898,.T.);
#47449=EDGE_CURVE('',#37216,#37215,#19899,.T.);
#47450=EDGE_CURVE('',#37217,#37216,#19900,.T.);
#47451=EDGE_CURVE('',#37218,#37217,#19901,.T.);
#47452=EDGE_CURVE('',#37219,#37218,#19902,.T.);
#47453=EDGE_CURVE('',#37220,#37219,#19903,.T.);
#47454=EDGE_CURVE('',#37221,#37220,#19904,.T.);
#47455=EDGE_CURVE('',#37222,#37221,#19905,.T.);
#47456=EDGE_CURVE('',#37223,#37222,#19906,.T.);
#47457=EDGE_CURVE('',#37224,#37223,#19907,.T.);
#47458=EDGE_CURVE('',#37225,#37224,#19908,.T.);
#47459=EDGE_CURVE('',#37226,#37225,#19909,.T.);
#47460=EDGE_CURVE('',#37227,#37226,#19910,.T.);
#47461=EDGE_CURVE('',#37228,#37227,#19911,.T.);
#47462=EDGE_CURVE('',#37229,#37228,#19912,.T.);
#47463=EDGE_CURVE('',#37230,#37229,#19913,.T.);
#47464=EDGE_CURVE('',#37231,#37230,#19914,.T.);
#47465=EDGE_CURVE('',#37232,#37231,#19915,.T.);
#47466=EDGE_CURVE('',#37233,#37232,#19916,.T.);
#47467=EDGE_CURVE('',#37234,#37233,#19917,.T.);
#47468=EDGE_CURVE('',#37235,#37234,#19918,.T.);
#47469=EDGE_CURVE('',#37236,#37235,#19919,.T.);
#47470=EDGE_CURVE('',#37237,#37236,#19920,.T.);
#47471=EDGE_CURVE('',#37238,#37237,#19921,.T.);
#47472=EDGE_CURVE('',#37239,#37238,#19922,.T.);
#47473=EDGE_CURVE('',#37240,#37239,#19923,.T.);
#47474=EDGE_CURVE('',#37241,#37240,#19924,.T.);
#47475=EDGE_CURVE('',#37242,#37241,#19925,.T.);
#47476=EDGE_CURVE('',#37243,#37242,#19926,.T.);
#47477=EDGE_CURVE('',#37244,#37243,#19927,.T.);
#47478=EDGE_CURVE('',#37245,#37244,#19928,.T.);
#47479=EDGE_CURVE('',#37246,#37245,#19929,.T.);
#47480=EDGE_CURVE('',#37247,#37246,#19930,.T.);
#47481=EDGE_CURVE('',#37248,#37247,#19931,.T.);
#47482=EDGE_CURVE('',#37249,#37248,#19932,.T.);
#47483=EDGE_CURVE('',#37250,#37249,#19933,.T.);
#47484=EDGE_CURVE('',#37251,#37250,#19934,.T.);
#47485=EDGE_CURVE('',#37252,#37251,#19935,.T.);
#47486=EDGE_CURVE('',#37253,#37252,#19936,.T.);
#47487=EDGE_CURVE('',#37254,#37253,#19937,.T.);
#47488=EDGE_CURVE('',#37255,#37254,#19938,.T.);
#47489=EDGE_CURVE('',#37125,#37255,#19939,.T.);
#47490=EDGE_CURVE('',#37256,#37124,#19940,.T.);
#47491=EDGE_CURVE('',#37257,#37256,#19941,.T.);
#47492=EDGE_CURVE('',#37129,#37257,#19942,.T.);
#47493=EDGE_CURVE('',#37258,#37128,#19943,.T.);
#47494=EDGE_CURVE('',#37259,#37258,#19944,.T.);
#47495=EDGE_CURVE('',#37260,#37259,#19945,.T.);
#47496=EDGE_CURVE('',#37261,#37260,#19946,.T.);
#47497=EDGE_CURVE('',#37262,#37261,#19947,.T.);
#47498=EDGE_CURVE('',#37263,#37262,#19948,.T.);
#47499=EDGE_CURVE('',#37264,#37263,#19949,.T.);
#47500=EDGE_CURVE('',#37265,#37264,#19950,.T.);
#47501=EDGE_CURVE('',#37266,#37265,#19951,.T.);
#47502=EDGE_CURVE('',#37267,#37266,#19952,.T.);
#47503=EDGE_CURVE('',#37268,#37267,#19953,.T.);
#47504=EDGE_CURVE('',#37269,#37268,#19954,.T.);
#47505=EDGE_CURVE('',#37270,#37269,#19955,.T.);
#47506=EDGE_CURVE('',#37271,#37270,#19956,.T.);
#47507=EDGE_CURVE('',#37272,#37271,#19957,.T.);
#47508=EDGE_CURVE('',#37273,#37272,#19958,.T.);
#47509=EDGE_CURVE('',#37274,#37273,#19959,.T.);
#47510=EDGE_CURVE('',#37275,#37274,#19960,.T.);
#47511=EDGE_CURVE('',#37276,#37275,#19961,.T.);
#47512=EDGE_CURVE('',#37277,#37276,#19962,.T.);
#47513=EDGE_CURVE('',#37278,#37277,#19963,.T.);
#47514=EDGE_CURVE('',#37279,#37278,#19964,.T.);
#47515=EDGE_CURVE('',#37141,#37279,#19965,.T.);
#47516=EDGE_CURVE('',#37280,#37281,#19966,.T.);
#47517=EDGE_CURVE('',#37281,#37282,#19967,.T.);
#47518=EDGE_CURVE('',#37282,#37104,#28323,.T.);
#47519=EDGE_CURVE('',#37103,#37283,#19968,.T.);
#47520=EDGE_CURVE('',#37283,#37284,#19969,.T.);
#47521=EDGE_CURVE('',#37284,#37285,#28324,.T.);
#47522=EDGE_CURVE('',#37285,#37280,#19970,.T.);
#47523=EDGE_CURVE('',#37286,#37287,#28325,.T.);
#47524=EDGE_CURVE('',#37287,#37288,#19971,.T.);
#47525=EDGE_CURVE('',#37288,#37100,#19972,.T.);
#47526=EDGE_CURVE('',#37099,#37289,#28326,.T.);
#47527=EDGE_CURVE('',#37289,#37290,#19973,.T.);
#47528=EDGE_CURVE('',#37290,#37291,#19974,.T.);
#47529=EDGE_CURVE('',#37291,#37286,#19975,.T.);
#47530=EDGE_CURVE('',#37141,#37292,#28327,.T.);
#47531=EDGE_CURVE('',#37293,#37279,#28328,.T.);
#47532=EDGE_CURVE('',#37292,#37293,#19976,.T.);
#47533=EDGE_CURVE('',#37294,#37143,#28329,.T.);
#47534=EDGE_CURVE('',#37295,#37294,#19977,.T.);
#47535=EDGE_CURVE('',#37144,#37295,#28330,.T.);
#47536=EDGE_CURVE('',#37276,#37296,#28331,.T.);
#47537=EDGE_CURVE('',#37297,#37275,#28332,.T.);
#47538=EDGE_CURVE('',#37296,#37297,#19978,.T.);
#47539=EDGE_CURVE('',#37272,#37298,#28333,.T.);
#47540=EDGE_CURVE('',#37299,#37271,#28334,.T.);
#47541=EDGE_CURVE('',#37298,#37299,#19979,.T.);
#47542=EDGE_CURVE('',#37268,#37300,#28335,.T.);
#47543=EDGE_CURVE('',#37301,#37267,#28336,.T.);
#47544=EDGE_CURVE('',#37300,#37301,#19980,.T.);
#47545=EDGE_CURVE('',#37302,#37255,#28337,.T.);
#47546=EDGE_CURVE('',#37126,#37302,#19981,.T.);
#47547=EDGE_CURVE('',#37303,#37257,#28338,.T.);
#47548=EDGE_CURVE('',#37130,#37303,#19982,.T.);
#47549=EDGE_CURVE('',#37304,#37259,#28339,.T.);
#47550=EDGE_CURVE('',#37305,#37304,#19983,.T.);
#47551=EDGE_CURVE('',#37260,#37305,#28340,.T.);
#47552=EDGE_CURVE('',#37264,#37306,#28341,.T.);
#47553=EDGE_CURVE('',#37307,#37263,#28342,.T.);
#47554=EDGE_CURVE('',#37306,#37307,#19984,.T.);
#47555=EDGE_CURVE('',#37164,#37308,#28343,.T.);
#47556=EDGE_CURVE('',#37309,#37163,#28344,.T.);
#47557=EDGE_CURVE('',#37308,#37309,#19985,.T.);
#47558=EDGE_CURVE('',#37310,#37167,#28345,.T.);
#47559=EDGE_CURVE('',#37311,#37310,#19986,.T.);
#47560=EDGE_CURVE('',#37168,#37311,#28346,.T.);
#47561=EDGE_CURVE('',#37160,#37312,#28347,.T.);
#47562=EDGE_CURVE('',#37313,#37159,#28348,.T.);
#47563=EDGE_CURVE('',#37312,#37313,#19987,.T.);
#47564=EDGE_CURVE('',#37314,#37135,#19988,.T.);
#47565=EDGE_CURVE('',#37170,#37314,#28349,.T.);
#47566=EDGE_CURVE('',#37315,#37139,#19989,.T.);
#47567=EDGE_CURVE('',#37172,#37315,#28350,.T.);
#47568=EDGE_CURVE('',#37316,#37175,#28351,.T.);
#47569=EDGE_CURVE('',#37317,#37316,#19990,.T.);
#47570=EDGE_CURVE('',#37176,#37317,#28352,.T.);
#47571=EDGE_CURVE('',#37152,#37318,#28353,.T.);
#47572=EDGE_CURVE('',#37319,#37151,#28354,.T.);
#47573=EDGE_CURVE('',#37318,#37319,#19991,.T.);
#47574=EDGE_CURVE('',#37320,#37155,#28355,.T.);
#47575=EDGE_CURVE('',#37321,#37320,#19992,.T.);
#47576=EDGE_CURVE('',#37156,#37321,#28356,.T.);
#47577=EDGE_CURVE('',#37148,#37322,#28357,.T.);
#47578=EDGE_CURVE('',#37323,#37147,#28358,.T.);
#47579=EDGE_CURVE('',#37322,#37323,#19993,.T.);
#47580=EDGE_CURVE('',#37196,#37324,#28359,.T.);
#47581=EDGE_CURVE('',#37325,#37195,#28360,.T.);
#47582=EDGE_CURVE('',#37324,#37325,#19994,.T.);
#47583=EDGE_CURVE('',#37326,#37199,#28361,.T.);
#47584=EDGE_CURVE('',#37327,#37326,#19995,.T.);
#47585=EDGE_CURVE('',#37200,#37327,#28362,.T.);
#47586=EDGE_CURVE('',#37192,#37328,#28363,.T.);
#47587=EDGE_CURVE('',#37329,#37191,#28364,.T.);
#47588=EDGE_CURVE('',#37328,#37329,#19996,.T.);
#47589=EDGE_CURVE('',#37330,#37203,#28365,.T.);
#47590=EDGE_CURVE('',#37331,#37330,#19997,.T.);
#47591=EDGE_CURVE('',#37204,#37331,#28366,.T.);
#47592=EDGE_CURVE('',#37332,#37207,#28367,.T.);
#47593=EDGE_CURVE('',#37333,#37332,#19998,.T.);
#47594=EDGE_CURVE('',#37208,#37333,#28368,.T.);
#47595=EDGE_CURVE('',#37334,#37211,#28369,.T.);
#47596=EDGE_CURVE('',#37335,#37334,#19999,.T.);
#47597=EDGE_CURVE('',#37212,#37335,#28370,.T.);
#47598=EDGE_CURVE('',#37184,#37336,#28371,.T.);
#47599=EDGE_CURVE('',#37337,#37183,#28372,.T.);
#47600=EDGE_CURVE('',#37336,#37337,#20000,.T.);
#47601=EDGE_CURVE('',#37338,#37187,#28373,.T.);
#47602=EDGE_CURVE('',#37339,#37338,#20001,.T.);
#47603=EDGE_CURVE('',#37188,#37339,#28374,.T.);
#47604=EDGE_CURVE('',#37180,#37340,#28375,.T.);
#47605=EDGE_CURVE('',#37341,#37179,#28376,.T.);
#47606=EDGE_CURVE('',#37340,#37341,#20002,.T.);
#47607=EDGE_CURVE('',#37232,#37342,#28377,.T.);
#47608=EDGE_CURVE('',#37343,#37231,#28378,.T.);
#47609=EDGE_CURVE('',#37342,#37343,#20003,.T.);
#47610=EDGE_CURVE('',#37344,#37235,#28379,.T.);
#47611=EDGE_CURVE('',#37345,#37344,#20004,.T.);
#47612=EDGE_CURVE('',#37236,#37345,#28380,.T.);
#47613=EDGE_CURVE('',#37228,#37346,#28381,.T.);
#47614=EDGE_CURVE('',#37347,#37227,#28382,.T.);
#47615=EDGE_CURVE('',#37346,#37347,#20005,.T.);
#47616=EDGE_CURVE('',#37348,#37239,#28383,.T.);
#47617=EDGE_CURVE('',#37349,#37348,#20006,.T.);
#47618=EDGE_CURVE('',#37240,#37349,#28384,.T.);
#47619=EDGE_CURVE('',#37350,#37243,#28385,.T.);
#47620=EDGE_CURVE('',#37351,#37350,#20007,.T.);
#47621=EDGE_CURVE('',#37244,#37351,#28386,.T.);
#47622=EDGE_CURVE('',#37352,#37247,#28387,.T.);
#47623=EDGE_CURVE('',#37353,#37352,#20008,.T.);
#47624=EDGE_CURVE('',#37248,#37353,#28388,.T.);
#47625=EDGE_CURVE('',#37224,#37354,#28389,.T.);
#47626=EDGE_CURVE('',#37355,#37223,#28390,.T.);
#47627=EDGE_CURVE('',#37354,#37355,#20009,.T.);
#47628=EDGE_CURVE('',#37220,#37356,#28391,.T.);
#47629=EDGE_CURVE('',#37357,#37219,#28392,.T.);
#47630=EDGE_CURVE('',#37356,#37357,#20010,.T.);
#47631=EDGE_CURVE('',#37216,#37358,#28393,.T.);
#47632=EDGE_CURVE('',#37359,#37215,#28394,.T.);
#47633=EDGE_CURVE('',#37358,#37359,#20011,.T.);
#47634=EDGE_CURVE('',#37360,#37292,#20012,.T.);
#47635=EDGE_CURVE('',#37361,#37293,#20013,.T.);
#47636=EDGE_CURVE('',#37361,#37362,#20014,.T.);
#47637=EDGE_CURVE('',#37362,#37296,#20015,.T.);
#47638=EDGE_CURVE('',#37363,#37297,#20016,.T.);
#47639=EDGE_CURVE('',#37363,#37364,#20017,.T.);
#47640=EDGE_CURVE('',#37364,#37298,#20018,.T.);
#47641=EDGE_CURVE('',#37365,#37299,#20019,.T.);
#47642=EDGE_CURVE('',#37365,#37366,#20020,.T.);
#47643=EDGE_CURVE('',#37366,#37300,#20021,.T.);
#47644=EDGE_CURVE('',#37367,#37301,#20022,.T.);
#47645=EDGE_CURVE('',#37367,#37368,#20023,.T.);
#47646=EDGE_CURVE('',#37368,#37306,#20024,.T.);
#47647=EDGE_CURVE('',#37369,#37307,#20025,.T.);
#47648=EDGE_CURVE('',#37369,#37370,#20026,.T.);
#47649=EDGE_CURVE('',#37370,#37305,#20027,.T.);
#47650=EDGE_CURVE('',#37371,#37304,#20028,.T.);
#47651=EDGE_CURVE('',#37371,#37131,#20029,.T.);
#47652=EDGE_CURVE('',#37372,#37303,#20030,.T.);
#47653=EDGE_CURVE('',#37372,#37127,#20031,.T.);
#47654=EDGE_CURVE('',#37373,#37302,#20032,.T.);
#47655=EDGE_CURVE('',#37373,#37374,#20033,.T.);
#47656=EDGE_CURVE('',#37374,#37375,#20034,.T.);
#47657=EDGE_CURVE('',#37375,#37376,#20035,.T.);
#47658=EDGE_CURVE('',#37377,#37376,#20036,.T.);
#47659=EDGE_CURVE('',#37377,#37378,#20037,.T.);
#47660=EDGE_CURVE('',#37378,#37353,#20038,.T.);
#47661=EDGE_CURVE('',#37379,#37352,#20039,.T.);
#47662=EDGE_CURVE('',#37379,#37380,#20040,.T.);
#47663=EDGE_CURVE('',#37380,#37351,#20041,.T.);
#47664=EDGE_CURVE('',#37381,#37350,#20042,.T.);
#47665=EDGE_CURVE('',#37381,#37382,#20043,.T.);
#47666=EDGE_CURVE('',#37382,#37349,#20044,.T.);
#47667=EDGE_CURVE('',#37383,#37348,#20045,.T.);
#47668=EDGE_CURVE('',#37383,#37384,#20046,.T.);
#47669=EDGE_CURVE('',#37384,#37345,#20047,.T.);
#47670=EDGE_CURVE('',#37385,#37344,#20048,.T.);
#47671=EDGE_CURVE('',#37385,#37386,#20049,.T.);
#47672=EDGE_CURVE('',#37386,#37342,#20050,.T.);
#47673=EDGE_CURVE('',#37387,#37343,#20051,.T.);
#47674=EDGE_CURVE('',#37387,#37388,#20052,.T.);
#47675=EDGE_CURVE('',#37388,#37346,#20053,.T.);
#47676=EDGE_CURVE('',#37389,#37347,#20054,.T.);
#47677=EDGE_CURVE('',#37389,#37390,#20055,.T.);
#47678=EDGE_CURVE('',#37390,#37354,#20056,.T.);
#47679=EDGE_CURVE('',#37391,#37355,#20057,.T.);
#47680=EDGE_CURVE('',#37391,#37392,#20058,.T.);
#47681=EDGE_CURVE('',#37392,#37356,#20059,.T.);
#47682=EDGE_CURVE('',#37393,#37357,#20060,.T.);
#47683=EDGE_CURVE('',#37393,#37394,#20061,.T.);
#47684=EDGE_CURVE('',#37394,#37358,#20062,.T.);
#47685=EDGE_CURVE('',#37395,#37359,#20063,.T.);
#47686=EDGE_CURVE('',#37395,#37396,#20064,.T.);
#47687=EDGE_CURVE('',#37396,#37335,#20065,.T.);
#47688=EDGE_CURVE('',#37397,#37334,#20066,.T.);
#47689=EDGE_CURVE('',#37397,#37398,#20067,.T.);
#47690=EDGE_CURVE('',#37398,#37333,#20068,.T.);
#47691=EDGE_CURVE('',#37399,#37332,#20069,.T.);
#47692=EDGE_CURVE('',#37399,#37400,#20070,.T.);
#47693=EDGE_CURVE('',#37400,#37331,#20071,.T.);
#47694=EDGE_CURVE('',#37401,#37330,#20072,.T.);
#47695=EDGE_CURVE('',#37401,#37402,#20073,.T.);
#47696=EDGE_CURVE('',#37402,#37327,#20074,.T.);
#47697=EDGE_CURVE('',#37403,#37326,#20075,.T.);
#47698=EDGE_CURVE('',#37403,#37404,#20076,.T.);
#47699=EDGE_CURVE('',#37404,#37324,#20077,.T.);
#47700=EDGE_CURVE('',#37405,#37325,#20078,.T.);
#47701=EDGE_CURVE('',#37405,#37406,#20079,.T.);
#47702=EDGE_CURVE('',#37406,#37328,#20080,.T.);
#47703=EDGE_CURVE('',#37407,#37329,#20081,.T.);
#47704=EDGE_CURVE('',#37407,#37408,#20082,.T.);
#47705=EDGE_CURVE('',#37408,#37339,#20083,.T.);
#47706=EDGE_CURVE('',#37409,#37338,#20084,.T.);
#47707=EDGE_CURVE('',#37409,#37410,#20085,.T.);
#47708=EDGE_CURVE('',#37410,#37336,#20086,.T.);
#47709=EDGE_CURVE('',#37411,#37337,#20087,.T.);
#47710=EDGE_CURVE('',#37411,#37412,#20088,.T.);
#47711=EDGE_CURVE('',#37412,#37340,#20089,.T.);
#47712=EDGE_CURVE('',#37413,#37341,#20090,.T.);
#47713=EDGE_CURVE('',#37413,#37414,#20091,.T.);
#47714=EDGE_CURVE('',#37414,#37317,#20092,.T.);
#47715=EDGE_CURVE('',#37415,#37316,#20093,.T.);
#47716=EDGE_CURVE('',#37415,#37416,#20094,.T.);
#47717=EDGE_CURVE('',#37416,#37315,#20095,.T.);
#47718=EDGE_CURVE('',#37138,#37417,#20096,.T.);
#47719=EDGE_CURVE('',#37417,#37314,#20097,.T.);
#47720=EDGE_CURVE('',#37134,#37418,#20098,.T.);
#47721=EDGE_CURVE('',#37418,#37311,#20099,.T.);
#47722=EDGE_CURVE('',#37419,#37310,#20100,.T.);
#47723=EDGE_CURVE('',#37419,#37420,#20101,.T.);
#47724=EDGE_CURVE('',#37420,#37308,#20102,.T.);
#47725=EDGE_CURVE('',#37421,#37309,#20103,.T.);
#47726=EDGE_CURVE('',#37421,#37422,#20104,.T.);
#47727=EDGE_CURVE('',#37422,#37312,#20105,.T.);
#47728=EDGE_CURVE('',#37423,#37313,#20106,.T.);
#47729=EDGE_CURVE('',#37423,#37424,#20107,.T.);
#47730=EDGE_CURVE('',#37424,#37321,#20108,.T.);
#47731=EDGE_CURVE('',#37425,#37320,#20109,.T.);
#47732=EDGE_CURVE('',#37425,#37426,#20110,.T.);
#47733=EDGE_CURVE('',#37426,#37318,#20111,.T.);
#47734=EDGE_CURVE('',#37427,#37319,#20112,.T.);
#47735=EDGE_CURVE('',#37427,#37428,#20113,.T.);
#47736=EDGE_CURVE('',#37428,#37322,#20114,.T.);
#47737=EDGE_CURVE('',#37429,#37323,#20115,.T.);
#47738=EDGE_CURVE('',#37429,#37430,#20116,.T.);
#47739=EDGE_CURVE('',#37430,#37295,#20117,.T.);
#47740=EDGE_CURVE('',#37431,#37294,#20118,.T.);
#47741=EDGE_CURVE('',#37431,#37360,#20119,.T.);
#47742=EDGE_CURVE('',#37252,#37375,#28395,.T.);
#47743=EDGE_CURVE('',#37376,#37251,#28396,.T.);
#47744=EDGE_CURVE('',#37249,#37378,#28397,.T.);
#47745=EDGE_CURVE('',#37250,#37377,#28398,.T.);
#47746=EDGE_CURVE('',#37253,#37374,#28399,.T.);
#47747=EDGE_CURVE('',#37254,#37373,#28400,.T.);
#47748=EDGE_CURVE('',#37213,#37396,#28401,.T.);
#47749=EDGE_CURVE('',#37214,#37395,#28402,.T.);
#47750=EDGE_CURVE('',#37217,#37394,#28403,.T.);
#47751=EDGE_CURVE('',#37218,#37393,#28404,.T.);
#47752=EDGE_CURVE('',#37221,#37392,#28405,.T.);
#47753=EDGE_CURVE('',#37222,#37391,#28406,.T.);
#47754=EDGE_CURVE('',#37225,#37390,#28407,.T.);
#47755=EDGE_CURVE('',#37226,#37389,#28408,.T.);
#47756=EDGE_CURVE('',#37245,#37380,#28409,.T.);
#47757=EDGE_CURVE('',#37246,#37379,#28410,.T.);
#47758=EDGE_CURVE('',#37241,#37382,#28411,.T.);
#47759=EDGE_CURVE('',#37242,#37381,#28412,.T.);
#47760=EDGE_CURVE('',#37237,#37384,#28413,.T.);
#47761=EDGE_CURVE('',#37238,#37383,#28414,.T.);
#47762=EDGE_CURVE('',#37229,#37388,#28415,.T.);
#47763=EDGE_CURVE('',#37230,#37387,#28416,.T.);
#47764=EDGE_CURVE('',#37233,#37386,#28417,.T.);
#47765=EDGE_CURVE('',#37234,#37385,#28418,.T.);
#47766=EDGE_CURVE('',#37177,#37414,#28419,.T.);
#47767=EDGE_CURVE('',#37178,#37413,#28420,.T.);
#47768=EDGE_CURVE('',#37181,#37412,#28421,.T.);
#47769=EDGE_CURVE('',#37182,#37411,#28422,.T.);
#47770=EDGE_CURVE('',#37189,#37408,#28423,.T.);
#47771=EDGE_CURVE('',#37190,#37407,#28424,.T.);
#47772=EDGE_CURVE('',#37185,#37410,#28425,.T.);
#47773=EDGE_CURVE('',#37186,#37409,#28426,.T.);
#47774=EDGE_CURVE('',#37209,#37398,#28427,.T.);
#47775=EDGE_CURVE('',#37210,#37397,#28428,.T.);
#47776=EDGE_CURVE('',#37205,#37400,#28429,.T.);
#47777=EDGE_CURVE('',#37206,#37399,#28430,.T.);
#47778=EDGE_CURVE('',#37201,#37402,#28431,.T.);
#47779=EDGE_CURVE('',#37202,#37401,#28432,.T.);
#47780=EDGE_CURVE('',#37193,#37406,#28433,.T.);
#47781=EDGE_CURVE('',#37194,#37405,#28434,.T.);
#47782=EDGE_CURVE('',#37197,#37404,#28435,.T.);
#47783=EDGE_CURVE('',#37198,#37403,#28436,.T.);
#47784=EDGE_CURVE('',#37145,#37430,#28437,.T.);
#47785=EDGE_CURVE('',#37146,#37429,#28438,.T.);
#47786=EDGE_CURVE('',#37149,#37428,#28439,.T.);
#47787=EDGE_CURVE('',#37150,#37427,#28440,.T.);
#47788=EDGE_CURVE('',#37157,#37424,#28441,.T.);
#47789=EDGE_CURVE('',#37158,#37423,#28442,.T.);
#47790=EDGE_CURVE('',#37153,#37426,#28443,.T.);
#47791=EDGE_CURVE('',#37154,#37425,#28444,.T.);
#47792=EDGE_CURVE('',#37173,#37416,#28445,.T.);
#47793=EDGE_CURVE('',#37174,#37415,#28446,.T.);
#47794=EDGE_CURVE('',#37171,#37417,#28447,.T.);
#47795=EDGE_CURVE('',#37169,#37418,#28448,.T.);
#47796=EDGE_CURVE('',#37161,#37422,#28449,.T.);
#47797=EDGE_CURVE('',#37162,#37421,#28450,.T.);
#47798=EDGE_CURVE('',#37165,#37420,#28451,.T.);
#47799=EDGE_CURVE('',#37166,#37419,#28452,.T.);
#47800=EDGE_CURVE('',#37261,#37370,#28453,.T.);
#47801=EDGE_CURVE('',#37262,#37369,#28454,.T.);
#47802=EDGE_CURVE('',#37265,#37368,#28455,.T.);
#47803=EDGE_CURVE('',#37266,#37367,#28456,.T.);
#47804=EDGE_CURVE('',#37258,#37371,#28457,.T.);
#47805=EDGE_CURVE('',#37256,#37372,#28458,.T.);
#47806=EDGE_CURVE('',#37269,#37366,#28459,.T.);
#47807=EDGE_CURVE('',#37270,#37365,#28460,.T.);
#47808=EDGE_CURVE('',#37273,#37364,#28461,.T.);
#47809=EDGE_CURVE('',#37274,#37363,#28462,.T.);
#47810=EDGE_CURVE('',#37277,#37362,#28463,.T.);
#47811=EDGE_CURVE('',#37278,#37361,#28464,.T.);
#47812=EDGE_CURVE('',#37140,#37360,#28465,.T.);
#47813=EDGE_CURVE('',#37142,#37431,#28466,.T.);
#47814=EDGE_CURVE('',#37432,#37433,#28467,.T.);
#47815=EDGE_CURVE('',#37433,#37118,#28468,.T.);
#47816=EDGE_CURVE('',#37121,#37432,#28469,.T.);
#47817=EDGE_CURVE('',#37434,#37435,#28470,.T.);
#47818=EDGE_CURVE('',#37435,#37433,#20120,.T.);
#47819=EDGE_CURVE('',#37432,#37434,#20121,.T.);
#47820=EDGE_CURVE('',#37436,#37437,#28471,.T.);
#47821=EDGE_CURVE('',#37437,#37435,#20122,.T.);
#47822=EDGE_CURVE('',#37434,#37436,#20123,.T.);
#47823=EDGE_CURVE('',#37438,#37439,#28472,.T.);
#47824=EDGE_CURVE('',#37439,#37437,#20124,.T.);
#47825=EDGE_CURVE('',#37436,#37438,#20125,.T.);
#47826=EDGE_CURVE('',#37440,#37102,#28473,.T.);
#47827=EDGE_CURVE('',#37102,#37439,#28474,.T.);
#47828=EDGE_CURVE('',#37438,#37440,#28475,.T.);
#47829=EDGE_CURVE('',#37441,#37101,#28476,.T.);
#47830=EDGE_CURVE('',#37440,#37441,#20126,.T.);
#47831=EDGE_CURVE('',#37119,#37101,#20127,.T.);
#47832=EDGE_CURVE('',#37441,#37120,#20128,.T.);
#47833=EDGE_CURVE('',#37442,#37443,#28477,.T.);
#47834=EDGE_CURVE('',#37443,#37444,#20129,.T.);
#47835=EDGE_CURVE('',#37445,#37444,#28478,.T.);
#47836=EDGE_CURVE('',#37445,#37442,#20130,.T.);
#47837=EDGE_CURVE('',#37115,#37443,#28479,.T.);
#47838=EDGE_CURVE('',#37442,#37116,#28480,.T.);
#47839=EDGE_CURVE('',#37446,#37098,#28481,.T.);
#47840=EDGE_CURVE('',#37098,#37114,#20131,.T.);
#47841=EDGE_CURVE('',#37117,#37446,#20132,.T.);
#47842=EDGE_CURVE('',#37447,#37097,#28482,.T.);
#47843=EDGE_CURVE('',#37446,#37447,#20133,.T.);
#47844=EDGE_CURVE('',#37448,#37449,#28483,.T.);
#47845=EDGE_CURVE('',#37449,#37097,#28484,.T.);
#47846=EDGE_CURVE('',#37447,#37448,#28485,.T.);
#47847=EDGE_CURVE('',#37450,#37451,#28486,.T.);
#47848=EDGE_CURVE('',#37451,#37449,#20134,.T.);
#47849=EDGE_CURVE('',#37448,#37450,#20135,.T.);
#47850=EDGE_CURVE('',#37444,#37451,#20136,.T.);
#47851=EDGE_CURVE('',#37450,#37445,#20137,.T.);
#47852=EDGE_CURVE('',#37119,#37283,#20138,.T.);
#47853=EDGE_CURVE('',#37284,#37118,#20139,.T.);
#47854=EDGE_CURVE('',#37285,#37433,#20140,.T.);
#47855=EDGE_CURVE('',#37280,#37435,#20141,.T.);
#47856=EDGE_CURVE('',#37281,#37437,#20142,.T.);
#47857=EDGE_CURVE('',#37439,#37282,#20143,.T.);
#47858=EDGE_CURVE('',#37449,#37289,#20144,.T.);
#47859=EDGE_CURVE('',#37290,#37451,#20145,.T.);
#47860=EDGE_CURVE('',#37291,#37444,#20146,.T.);
#47861=EDGE_CURVE('',#37286,#37443,#20147,.T.);
#47862=EDGE_CURVE('',#37287,#37115,#20148,.T.);
#47863=EDGE_CURVE('',#37114,#37288,#20149,.T.);
#63834=ORIENTED_EDGE('',*,*,#46419,.F.);
#63835=ORIENTED_EDGE('',*,*,#46420,.T.);
#63836=ORIENTED_EDGE('',*,*,#46421,.F.);
#63837=ORIENTED_EDGE('',*,*,#46422,.F.);
#63838=ORIENTED_EDGE('',*,*,#46423,.F.);
#63839=ORIENTED_EDGE('',*,*,#46424,.T.);
#63840=ORIENTED_EDGE('',*,*,#46425,.F.);
#63841=ORIENTED_EDGE('',*,*,#46426,.F.);
#63842=ORIENTED_EDGE('',*,*,#46427,.F.);
#63843=ORIENTED_EDGE('',*,*,#46428,.T.);
#63844=ORIENTED_EDGE('',*,*,#46429,.F.);
#63845=ORIENTED_EDGE('',*,*,#46430,.F.);
#63846=ORIENTED_EDGE('',*,*,#46431,.F.);
#63847=ORIENTED_EDGE('',*,*,#46432,.T.);
#63848=ORIENTED_EDGE('',*,*,#46433,.F.);
#63849=ORIENTED_EDGE('',*,*,#46434,.F.);
#63850=ORIENTED_EDGE('',*,*,#46435,.F.);
#63851=ORIENTED_EDGE('',*,*,#46436,.T.);
#63852=ORIENTED_EDGE('',*,*,#46437,.F.);
#63853=ORIENTED_EDGE('',*,*,#46438,.F.);
#63854=ORIENTED_EDGE('',*,*,#46439,.F.);
#63855=ORIENTED_EDGE('',*,*,#46440,.T.);
#63856=ORIENTED_EDGE('',*,*,#46441,.F.);
#63857=ORIENTED_EDGE('',*,*,#46442,.F.);
#63858=ORIENTED_EDGE('',*,*,#46443,.F.);
#63859=ORIENTED_EDGE('',*,*,#46444,.T.);
#63860=ORIENTED_EDGE('',*,*,#46445,.F.);
#63861=ORIENTED_EDGE('',*,*,#46446,.F.);
#63862=ORIENTED_EDGE('',*,*,#46447,.F.);
#63863=ORIENTED_EDGE('',*,*,#46448,.T.);
#63864=ORIENTED_EDGE('',*,*,#46449,.F.);
#63865=ORIENTED_EDGE('',*,*,#46450,.F.);
#63866=ORIENTED_EDGE('',*,*,#46451,.F.);
#63867=ORIENTED_EDGE('',*,*,#46452,.T.);
#63868=ORIENTED_EDGE('',*,*,#46453,.F.);
#63869=ORIENTED_EDGE('',*,*,#46454,.F.);
#63870=ORIENTED_EDGE('',*,*,#46455,.F.);
#63871=ORIENTED_EDGE('',*,*,#46456,.T.);
#63872=ORIENTED_EDGE('',*,*,#46457,.F.);
#63873=ORIENTED_EDGE('',*,*,#46458,.F.);
#63874=ORIENTED_EDGE('',*,*,#46459,.F.);
#63875=ORIENTED_EDGE('',*,*,#46460,.T.);
#63876=ORIENTED_EDGE('',*,*,#46461,.F.);
#63877=ORIENTED_EDGE('',*,*,#46462,.F.);
#63878=ORIENTED_EDGE('',*,*,#46463,.F.);
#63879=ORIENTED_EDGE('',*,*,#46464,.T.);
#63880=ORIENTED_EDGE('',*,*,#46465,.F.);
#63881=ORIENTED_EDGE('',*,*,#46466,.F.);
#63882=ORIENTED_EDGE('',*,*,#46467,.F.);
#63883=ORIENTED_EDGE('',*,*,#46468,.T.);
#63884=ORIENTED_EDGE('',*,*,#46469,.F.);
#63885=ORIENTED_EDGE('',*,*,#46470,.F.);
#63886=ORIENTED_EDGE('',*,*,#46471,.F.);
#63887=ORIENTED_EDGE('',*,*,#46472,.T.);
#63888=ORIENTED_EDGE('',*,*,#46473,.F.);
#63889=ORIENTED_EDGE('',*,*,#46474,.F.);
#63890=ORIENTED_EDGE('',*,*,#46475,.F.);
#63891=ORIENTED_EDGE('',*,*,#46476,.T.);
#63892=ORIENTED_EDGE('',*,*,#46477,.F.);
#63893=ORIENTED_EDGE('',*,*,#46478,.F.);
#63894=ORIENTED_EDGE('',*,*,#46479,.F.);
#63895=ORIENTED_EDGE('',*,*,#46480,.T.);
#63896=ORIENTED_EDGE('',*,*,#46481,.F.);
#63897=ORIENTED_EDGE('',*,*,#46482,.F.);
#63898=ORIENTED_EDGE('',*,*,#46483,.F.);
#63899=ORIENTED_EDGE('',*,*,#46484,.T.);
#63900=ORIENTED_EDGE('',*,*,#46485,.F.);
#63901=ORIENTED_EDGE('',*,*,#46486,.F.);
#63902=ORIENTED_EDGE('',*,*,#46487,.F.);
#63903=ORIENTED_EDGE('',*,*,#46488,.T.);
#63904=ORIENTED_EDGE('',*,*,#46489,.F.);
#63905=ORIENTED_EDGE('',*,*,#46490,.F.);
#63906=ORIENTED_EDGE('',*,*,#46491,.F.);
#63907=ORIENTED_EDGE('',*,*,#46492,.T.);
#63908=ORIENTED_EDGE('',*,*,#46493,.F.);
#63909=ORIENTED_EDGE('',*,*,#46494,.F.);
#63910=ORIENTED_EDGE('',*,*,#46495,.F.);
#63911=ORIENTED_EDGE('',*,*,#46496,.T.);
#63912=ORIENTED_EDGE('',*,*,#46497,.F.);
#63913=ORIENTED_EDGE('',*,*,#46498,.F.);
#63914=ORIENTED_EDGE('',*,*,#46499,.F.);
#63915=ORIENTED_EDGE('',*,*,#46500,.T.);
#63916=ORIENTED_EDGE('',*,*,#46501,.F.);
#63917=ORIENTED_EDGE('',*,*,#46502,.F.);
#63918=ORIENTED_EDGE('',*,*,#46503,.F.);
#63919=ORIENTED_EDGE('',*,*,#46504,.T.);
#63920=ORIENTED_EDGE('',*,*,#46505,.F.);
#63921=ORIENTED_EDGE('',*,*,#46506,.F.);
#63922=ORIENTED_EDGE('',*,*,#46507,.F.);
#63923=ORIENTED_EDGE('',*,*,#46508,.T.);
#63924=ORIENTED_EDGE('',*,*,#46509,.F.);
#63925=ORIENTED_EDGE('',*,*,#46510,.F.);
#63926=ORIENTED_EDGE('',*,*,#46511,.F.);
#63927=ORIENTED_EDGE('',*,*,#46512,.T.);
#63928=ORIENTED_EDGE('',*,*,#46513,.F.);
#63929=ORIENTED_EDGE('',*,*,#46514,.F.);
#63930=ORIENTED_EDGE('',*,*,#46515,.F.);
#63931=ORIENTED_EDGE('',*,*,#46516,.T.);
#63932=ORIENTED_EDGE('',*,*,#46517,.F.);
#63933=ORIENTED_EDGE('',*,*,#46518,.F.);
#63934=ORIENTED_EDGE('',*,*,#46519,.F.);
#63935=ORIENTED_EDGE('',*,*,#46520,.T.);
#63936=ORIENTED_EDGE('',*,*,#46521,.F.);
#63937=ORIENTED_EDGE('',*,*,#46522,.F.);
#63938=ORIENTED_EDGE('',*,*,#46523,.F.);
#63939=ORIENTED_EDGE('',*,*,#46524,.T.);
#63940=ORIENTED_EDGE('',*,*,#46525,.F.);
#63941=ORIENTED_EDGE('',*,*,#46526,.F.);
#63942=ORIENTED_EDGE('',*,*,#46527,.F.);
#63943=ORIENTED_EDGE('',*,*,#46528,.T.);
#63944=ORIENTED_EDGE('',*,*,#46529,.F.);
#63945=ORIENTED_EDGE('',*,*,#46530,.F.);
#63946=ORIENTED_EDGE('',*,*,#46531,.F.);
#63947=ORIENTED_EDGE('',*,*,#46532,.T.);
#63948=ORIENTED_EDGE('',*,*,#46533,.F.);
#63949=ORIENTED_EDGE('',*,*,#46534,.F.);
#63950=ORIENTED_EDGE('',*,*,#46535,.F.);
#63951=ORIENTED_EDGE('',*,*,#46536,.T.);
#63952=ORIENTED_EDGE('',*,*,#46537,.F.);
#63953=ORIENTED_EDGE('',*,*,#46538,.F.);
#63954=ORIENTED_EDGE('',*,*,#46539,.F.);
#63955=ORIENTED_EDGE('',*,*,#46540,.T.);
#63956=ORIENTED_EDGE('',*,*,#46541,.F.);
#63957=ORIENTED_EDGE('',*,*,#46542,.F.);
#63958=ORIENTED_EDGE('',*,*,#46543,.F.);
#63959=ORIENTED_EDGE('',*,*,#46544,.T.);
#63960=ORIENTED_EDGE('',*,*,#46545,.F.);
#63961=ORIENTED_EDGE('',*,*,#46546,.F.);
#63962=ORIENTED_EDGE('',*,*,#46547,.F.);
#63963=ORIENTED_EDGE('',*,*,#46548,.T.);
#63964=ORIENTED_EDGE('',*,*,#46549,.F.);
#63965=ORIENTED_EDGE('',*,*,#46550,.F.);
#63966=ORIENTED_EDGE('',*,*,#46551,.F.);
#63967=ORIENTED_EDGE('',*,*,#46552,.T.);
#63968=ORIENTED_EDGE('',*,*,#46553,.F.);
#63969=ORIENTED_EDGE('',*,*,#46554,.F.);
#63970=ORIENTED_EDGE('',*,*,#46555,.F.);
#63971=ORIENTED_EDGE('',*,*,#46556,.T.);
#63972=ORIENTED_EDGE('',*,*,#46557,.F.);
#63973=ORIENTED_EDGE('',*,*,#46558,.F.);
#63974=ORIENTED_EDGE('',*,*,#46559,.F.);
#63975=ORIENTED_EDGE('',*,*,#46560,.T.);
#63976=ORIENTED_EDGE('',*,*,#46561,.F.);
#63977=ORIENTED_EDGE('',*,*,#46562,.F.);
#63978=ORIENTED_EDGE('',*,*,#46563,.F.);
#63979=ORIENTED_EDGE('',*,*,#46564,.T.);
#63980=ORIENTED_EDGE('',*,*,#46565,.F.);
#63981=ORIENTED_EDGE('',*,*,#46566,.F.);
#63982=ORIENTED_EDGE('',*,*,#46567,.F.);
#63983=ORIENTED_EDGE('',*,*,#46568,.T.);
#63984=ORIENTED_EDGE('',*,*,#46569,.F.);
#63985=ORIENTED_EDGE('',*,*,#46570,.F.);
#63986=ORIENTED_EDGE('',*,*,#46571,.F.);
#63987=ORIENTED_EDGE('',*,*,#46572,.T.);
#63988=ORIENTED_EDGE('',*,*,#46573,.F.);
#63989=ORIENTED_EDGE('',*,*,#46574,.F.);
#63990=ORIENTED_EDGE('',*,*,#46575,.F.);
#63991=ORIENTED_EDGE('',*,*,#46576,.T.);
#63992=ORIENTED_EDGE('',*,*,#46577,.F.);
#63993=ORIENTED_EDGE('',*,*,#46578,.F.);
#63994=ORIENTED_EDGE('',*,*,#46579,.F.);
#63995=ORIENTED_EDGE('',*,*,#46580,.T.);
#63996=ORIENTED_EDGE('',*,*,#46581,.F.);
#63997=ORIENTED_EDGE('',*,*,#46582,.F.);
#63998=ORIENTED_EDGE('',*,*,#46583,.F.);
#63999=ORIENTED_EDGE('',*,*,#46584,.T.);
#64000=ORIENTED_EDGE('',*,*,#46585,.F.);
#64001=ORIENTED_EDGE('',*,*,#46586,.F.);
#64002=ORIENTED_EDGE('',*,*,#46587,.F.);
#64003=ORIENTED_EDGE('',*,*,#46588,.T.);
#64004=ORIENTED_EDGE('',*,*,#46589,.F.);
#64005=ORIENTED_EDGE('',*,*,#46590,.F.);
#64006=ORIENTED_EDGE('',*,*,#46591,.F.);
#64007=ORIENTED_EDGE('',*,*,#46592,.T.);
#64008=ORIENTED_EDGE('',*,*,#46593,.F.);
#64009=ORIENTED_EDGE('',*,*,#46594,.F.);
#64010=ORIENTED_EDGE('',*,*,#46595,.F.);
#64011=ORIENTED_EDGE('',*,*,#46596,.T.);
#64012=ORIENTED_EDGE('',*,*,#46597,.F.);
#64013=ORIENTED_EDGE('',*,*,#46598,.F.);
#64014=ORIENTED_EDGE('',*,*,#46599,.F.);
#64015=ORIENTED_EDGE('',*,*,#46600,.T.);
#64016=ORIENTED_EDGE('',*,*,#46601,.F.);
#64017=ORIENTED_EDGE('',*,*,#46602,.F.);
#64018=ORIENTED_EDGE('',*,*,#46603,.F.);
#64019=ORIENTED_EDGE('',*,*,#46604,.T.);
#64020=ORIENTED_EDGE('',*,*,#46605,.F.);
#64021=ORIENTED_EDGE('',*,*,#46606,.F.);
#64022=ORIENTED_EDGE('',*,*,#46607,.F.);
#64023=ORIENTED_EDGE('',*,*,#46608,.T.);
#64024=ORIENTED_EDGE('',*,*,#46609,.F.);
#64025=ORIENTED_EDGE('',*,*,#46610,.F.);
#64026=ORIENTED_EDGE('',*,*,#46611,.F.);
#64027=ORIENTED_EDGE('',*,*,#46612,.T.);
#64028=ORIENTED_EDGE('',*,*,#46613,.F.);
#64029=ORIENTED_EDGE('',*,*,#46614,.F.);
#64030=ORIENTED_EDGE('',*,*,#46615,.F.);
#64031=ORIENTED_EDGE('',*,*,#46616,.T.);
#64032=ORIENTED_EDGE('',*,*,#46617,.F.);
#64033=ORIENTED_EDGE('',*,*,#46618,.F.);
#64034=ORIENTED_EDGE('',*,*,#46619,.F.);
#64035=ORIENTED_EDGE('',*,*,#46620,.T.);
#64036=ORIENTED_EDGE('',*,*,#46621,.F.);
#64037=ORIENTED_EDGE('',*,*,#46622,.F.);
#64038=ORIENTED_EDGE('',*,*,#46623,.F.);
#64039=ORIENTED_EDGE('',*,*,#46624,.T.);
#64040=ORIENTED_EDGE('',*,*,#46625,.F.);
#64041=ORIENTED_EDGE('',*,*,#46626,.F.);
#64042=ORIENTED_EDGE('',*,*,#46627,.F.);
#64043=ORIENTED_EDGE('',*,*,#46628,.T.);
#64044=ORIENTED_EDGE('',*,*,#46629,.F.);
#64045=ORIENTED_EDGE('',*,*,#46630,.F.);
#64046=ORIENTED_EDGE('',*,*,#46631,.F.);
#64047=ORIENTED_EDGE('',*,*,#46632,.T.);
#64048=ORIENTED_EDGE('',*,*,#46633,.F.);
#64049=ORIENTED_EDGE('',*,*,#46634,.F.);
#64050=ORIENTED_EDGE('',*,*,#46635,.F.);
#64051=ORIENTED_EDGE('',*,*,#46636,.T.);
#64052=ORIENTED_EDGE('',*,*,#46637,.F.);
#64053=ORIENTED_EDGE('',*,*,#46638,.F.);
#64054=ORIENTED_EDGE('',*,*,#46639,.F.);
#64055=ORIENTED_EDGE('',*,*,#46640,.T.);
#64056=ORIENTED_EDGE('',*,*,#46641,.F.);
#64057=ORIENTED_EDGE('',*,*,#46642,.F.);
#64058=ORIENTED_EDGE('',*,*,#46643,.F.);
#64059=ORIENTED_EDGE('',*,*,#46644,.T.);
#64060=ORIENTED_EDGE('',*,*,#46645,.F.);
#64061=ORIENTED_EDGE('',*,*,#46646,.F.);
#64062=ORIENTED_EDGE('',*,*,#46647,.F.);
#64063=ORIENTED_EDGE('',*,*,#46648,.T.);
#64064=ORIENTED_EDGE('',*,*,#46649,.F.);
#64065=ORIENTED_EDGE('',*,*,#46650,.F.);
#64066=ORIENTED_EDGE('',*,*,#46651,.F.);
#64067=ORIENTED_EDGE('',*,*,#46652,.T.);
#64068=ORIENTED_EDGE('',*,*,#46653,.F.);
#64069=ORIENTED_EDGE('',*,*,#46654,.F.);
#64070=ORIENTED_EDGE('',*,*,#46655,.F.);
#64071=ORIENTED_EDGE('',*,*,#46656,.T.);
#64072=ORIENTED_EDGE('',*,*,#46657,.F.);
#64073=ORIENTED_EDGE('',*,*,#46658,.F.);
#64074=ORIENTED_EDGE('',*,*,#46659,.F.);
#64075=ORIENTED_EDGE('',*,*,#46660,.T.);
#64076=ORIENTED_EDGE('',*,*,#46661,.F.);
#64077=ORIENTED_EDGE('',*,*,#46662,.F.);
#64078=ORIENTED_EDGE('',*,*,#46663,.F.);
#64079=ORIENTED_EDGE('',*,*,#46664,.T.);
#64080=ORIENTED_EDGE('',*,*,#46665,.F.);
#64081=ORIENTED_EDGE('',*,*,#46666,.F.);
#64082=ORIENTED_EDGE('',*,*,#46667,.F.);
#64083=ORIENTED_EDGE('',*,*,#46668,.T.);
#64084=ORIENTED_EDGE('',*,*,#46669,.F.);
#64085=ORIENTED_EDGE('',*,*,#46670,.F.);
#64086=ORIENTED_EDGE('',*,*,#46671,.F.);
#64087=ORIENTED_EDGE('',*,*,#46672,.T.);
#64088=ORIENTED_EDGE('',*,*,#46673,.F.);
#64089=ORIENTED_EDGE('',*,*,#46674,.F.);
#64090=ORIENTED_EDGE('',*,*,#46675,.F.);
#64091=ORIENTED_EDGE('',*,*,#46676,.T.);
#64092=ORIENTED_EDGE('',*,*,#46677,.F.);
#64093=ORIENTED_EDGE('',*,*,#46678,.F.);
#64094=ORIENTED_EDGE('',*,*,#46679,.F.);
#64095=ORIENTED_EDGE('',*,*,#46680,.T.);
#64096=ORIENTED_EDGE('',*,*,#46681,.F.);
#64097=ORIENTED_EDGE('',*,*,#46682,.F.);
#64098=ORIENTED_EDGE('',*,*,#46683,.F.);
#64099=ORIENTED_EDGE('',*,*,#46684,.T.);
#64100=ORIENTED_EDGE('',*,*,#46685,.F.);
#64101=ORIENTED_EDGE('',*,*,#46686,.F.);
#64102=ORIENTED_EDGE('',*,*,#46687,.F.);
#64103=ORIENTED_EDGE('',*,*,#46688,.T.);
#64104=ORIENTED_EDGE('',*,*,#46689,.F.);
#64105=ORIENTED_EDGE('',*,*,#46690,.F.);
#64106=ORIENTED_EDGE('',*,*,#46691,.F.);
#64107=ORIENTED_EDGE('',*,*,#46692,.T.);
#64108=ORIENTED_EDGE('',*,*,#46693,.F.);
#64109=ORIENTED_EDGE('',*,*,#46694,.F.);
#64110=ORIENTED_EDGE('',*,*,#46695,.F.);
#64111=ORIENTED_EDGE('',*,*,#46696,.T.);
#64112=ORIENTED_EDGE('',*,*,#46697,.F.);
#64113=ORIENTED_EDGE('',*,*,#46698,.F.);
#64114=ORIENTED_EDGE('',*,*,#46699,.F.);
#64115=ORIENTED_EDGE('',*,*,#46700,.T.);
#64116=ORIENTED_EDGE('',*,*,#46701,.F.);
#64117=ORIENTED_EDGE('',*,*,#46700,.F.);
#64118=ORIENTED_EDGE('',*,*,#46702,.F.);
#64119=ORIENTED_EDGE('',*,*,#46703,.F.);
#64120=ORIENTED_EDGE('',*,*,#46704,.T.);
#64121=ORIENTED_EDGE('',*,*,#46705,.F.);
#64122=ORIENTED_EDGE('',*,*,#46704,.F.);
#64123=ORIENTED_EDGE('',*,*,#46706,.F.);
#64124=ORIENTED_EDGE('',*,*,#46707,.F.);
#64125=ORIENTED_EDGE('',*,*,#46708,.T.);
#64126=ORIENTED_EDGE('',*,*,#46709,.F.);
#64127=ORIENTED_EDGE('',*,*,#46708,.F.);
#64128=ORIENTED_EDGE('',*,*,#46710,.F.);
#64129=ORIENTED_EDGE('',*,*,#46711,.F.);
#64130=ORIENTED_EDGE('',*,*,#46712,.T.);
#64131=ORIENTED_EDGE('',*,*,#46713,.F.);
#64132=ORIENTED_EDGE('',*,*,#46712,.F.);
#64133=ORIENTED_EDGE('',*,*,#46714,.F.);
#64134=ORIENTED_EDGE('',*,*,#46715,.F.);
#64135=ORIENTED_EDGE('',*,*,#46716,.T.);
#64136=ORIENTED_EDGE('',*,*,#46717,.F.);
#64137=ORIENTED_EDGE('',*,*,#46716,.F.);
#64138=ORIENTED_EDGE('',*,*,#46718,.F.);
#64139=ORIENTED_EDGE('',*,*,#46719,.T.);
#64140=ORIENTED_EDGE('',*,*,#46720,.F.);
#64141=ORIENTED_EDGE('',*,*,#46719,.F.);
#64142=ORIENTED_EDGE('',*,*,#46721,.F.);
#64143=ORIENTED_EDGE('',*,*,#46722,.T.);
#64144=ORIENTED_EDGE('',*,*,#46723,.F.);
#64145=ORIENTED_EDGE('',*,*,#46722,.F.);
#64146=ORIENTED_EDGE('',*,*,#46724,.F.);
#64147=ORIENTED_EDGE('',*,*,#46725,.F.);
#64148=ORIENTED_EDGE('',*,*,#46726,.T.);
#64149=ORIENTED_EDGE('',*,*,#46727,.F.);
#64150=ORIENTED_EDGE('',*,*,#46726,.F.);
#64151=ORIENTED_EDGE('',*,*,#46703,.T.);
#64152=ORIENTED_EDGE('',*,*,#46728,.T.);
#64153=ORIENTED_EDGE('',*,*,#46718,.T.);
#64154=ORIENTED_EDGE('',*,*,#46728,.F.);
#64155=ORIENTED_EDGE('',*,*,#46706,.T.);
#64156=ORIENTED_EDGE('',*,*,#46707,.T.);
#64157=ORIENTED_EDGE('',*,*,#46729,.T.);
#64158=ORIENTED_EDGE('',*,*,#46715,.T.);
#64159=ORIENTED_EDGE('',*,*,#46729,.F.);
#64160=ORIENTED_EDGE('',*,*,#46710,.T.);
#64161=ORIENTED_EDGE('',*,*,#46730,.F.);
#64162=ORIENTED_EDGE('',*,*,#46731,.F.);
#64163=ORIENTED_EDGE('',*,*,#46696,.F.);
#64164=ORIENTED_EDGE('',*,*,#46732,.F.);
#64165=ORIENTED_EDGE('',*,*,#46733,.F.);
#64166=ORIENTED_EDGE('',*,*,#46734,.F.);
#64167=ORIENTED_EDGE('',*,*,#46692,.F.);
#64168=ORIENTED_EDGE('',*,*,#46735,.F.);
#64169=ORIENTED_EDGE('',*,*,#46736,.F.);
#64170=ORIENTED_EDGE('',*,*,#46737,.F.);
#64171=ORIENTED_EDGE('',*,*,#46688,.F.);
#64172=ORIENTED_EDGE('',*,*,#46738,.F.);
#64173=ORIENTED_EDGE('',*,*,#46739,.F.);
#64174=ORIENTED_EDGE('',*,*,#46740,.F.);
#64175=ORIENTED_EDGE('',*,*,#46684,.F.);
#64176=ORIENTED_EDGE('',*,*,#46741,.F.);
#64177=ORIENTED_EDGE('',*,*,#46742,.F.);
#64178=ORIENTED_EDGE('',*,*,#46743,.F.);
#64179=ORIENTED_EDGE('',*,*,#46680,.F.);
#64180=ORIENTED_EDGE('',*,*,#46744,.F.);
#64181=ORIENTED_EDGE('',*,*,#46745,.F.);
#64182=ORIENTED_EDGE('',*,*,#46746,.F.);
#64183=ORIENTED_EDGE('',*,*,#46676,.F.);
#64184=ORIENTED_EDGE('',*,*,#46747,.F.);
#64185=ORIENTED_EDGE('',*,*,#46748,.F.);
#64186=ORIENTED_EDGE('',*,*,#46749,.F.);
#64187=ORIENTED_EDGE('',*,*,#46672,.F.);
#64188=ORIENTED_EDGE('',*,*,#46750,.F.);
#64189=ORIENTED_EDGE('',*,*,#46751,.F.);
#64190=ORIENTED_EDGE('',*,*,#46752,.F.);
#64191=ORIENTED_EDGE('',*,*,#46668,.F.);
#64192=ORIENTED_EDGE('',*,*,#46753,.F.);
#64193=ORIENTED_EDGE('',*,*,#46754,.F.);
#64194=ORIENTED_EDGE('',*,*,#46755,.F.);
#64195=ORIENTED_EDGE('',*,*,#46664,.F.);
#64196=ORIENTED_EDGE('',*,*,#46756,.F.);
#64197=ORIENTED_EDGE('',*,*,#46757,.F.);
#64198=ORIENTED_EDGE('',*,*,#46758,.F.);
#64199=ORIENTED_EDGE('',*,*,#46660,.F.);
#64200=ORIENTED_EDGE('',*,*,#46759,.F.);
#64201=ORIENTED_EDGE('',*,*,#46760,.F.);
#64202=ORIENTED_EDGE('',*,*,#46761,.F.);
#64203=ORIENTED_EDGE('',*,*,#46656,.F.);
#64204=ORIENTED_EDGE('',*,*,#46762,.F.);
#64205=ORIENTED_EDGE('',*,*,#46763,.F.);
#64206=ORIENTED_EDGE('',*,*,#46764,.F.);
#64207=ORIENTED_EDGE('',*,*,#46652,.F.);
#64208=ORIENTED_EDGE('',*,*,#46765,.F.);
#64209=ORIENTED_EDGE('',*,*,#46766,.F.);
#64210=ORIENTED_EDGE('',*,*,#46767,.F.);
#64211=ORIENTED_EDGE('',*,*,#46648,.F.);
#64212=ORIENTED_EDGE('',*,*,#46768,.F.);
#64213=ORIENTED_EDGE('',*,*,#46769,.F.);
#64214=ORIENTED_EDGE('',*,*,#46770,.F.);
#64215=ORIENTED_EDGE('',*,*,#46644,.F.);
#64216=ORIENTED_EDGE('',*,*,#46771,.F.);
#64217=ORIENTED_EDGE('',*,*,#46772,.F.);
#64218=ORIENTED_EDGE('',*,*,#46773,.F.);
#64219=ORIENTED_EDGE('',*,*,#46640,.F.);
#64220=ORIENTED_EDGE('',*,*,#46774,.F.);
#64221=ORIENTED_EDGE('',*,*,#46775,.F.);
#64222=ORIENTED_EDGE('',*,*,#46776,.F.);
#64223=ORIENTED_EDGE('',*,*,#46636,.F.);
#64224=ORIENTED_EDGE('',*,*,#46777,.F.);
#64225=ORIENTED_EDGE('',*,*,#46778,.F.);
#64226=ORIENTED_EDGE('',*,*,#46779,.F.);
#64227=ORIENTED_EDGE('',*,*,#46632,.F.);
#64228=ORIENTED_EDGE('',*,*,#46780,.F.);
#64229=ORIENTED_EDGE('',*,*,#46781,.F.);
#64230=ORIENTED_EDGE('',*,*,#46782,.F.);
#64231=ORIENTED_EDGE('',*,*,#46628,.F.);
#64232=ORIENTED_EDGE('',*,*,#46783,.F.);
#64233=ORIENTED_EDGE('',*,*,#46784,.F.);
#64234=ORIENTED_EDGE('',*,*,#46785,.F.);
#64235=ORIENTED_EDGE('',*,*,#46624,.F.);
#64236=ORIENTED_EDGE('',*,*,#46786,.F.);
#64237=ORIENTED_EDGE('',*,*,#46787,.F.);
#64238=ORIENTED_EDGE('',*,*,#46788,.F.);
#64239=ORIENTED_EDGE('',*,*,#46620,.F.);
#64240=ORIENTED_EDGE('',*,*,#46789,.F.);
#64241=ORIENTED_EDGE('',*,*,#46790,.F.);
#64242=ORIENTED_EDGE('',*,*,#46791,.F.);
#64243=ORIENTED_EDGE('',*,*,#46616,.F.);
#64244=ORIENTED_EDGE('',*,*,#46792,.F.);
#64245=ORIENTED_EDGE('',*,*,#46793,.F.);
#64246=ORIENTED_EDGE('',*,*,#46794,.F.);
#64247=ORIENTED_EDGE('',*,*,#46612,.F.);
#64248=ORIENTED_EDGE('',*,*,#46795,.F.);
#64249=ORIENTED_EDGE('',*,*,#46796,.F.);
#64250=ORIENTED_EDGE('',*,*,#46797,.F.);
#64251=ORIENTED_EDGE('',*,*,#46608,.F.);
#64252=ORIENTED_EDGE('',*,*,#46798,.F.);
#64253=ORIENTED_EDGE('',*,*,#46799,.F.);
#64254=ORIENTED_EDGE('',*,*,#46800,.F.);
#64255=ORIENTED_EDGE('',*,*,#46604,.F.);
#64256=ORIENTED_EDGE('',*,*,#46801,.F.);
#64257=ORIENTED_EDGE('',*,*,#46802,.F.);
#64258=ORIENTED_EDGE('',*,*,#46803,.F.);
#64259=ORIENTED_EDGE('',*,*,#46600,.F.);
#64260=ORIENTED_EDGE('',*,*,#46804,.F.);
#64261=ORIENTED_EDGE('',*,*,#46805,.F.);
#64262=ORIENTED_EDGE('',*,*,#46806,.F.);
#64263=ORIENTED_EDGE('',*,*,#46596,.F.);
#64264=ORIENTED_EDGE('',*,*,#46807,.F.);
#64265=ORIENTED_EDGE('',*,*,#46808,.F.);
#64266=ORIENTED_EDGE('',*,*,#46809,.F.);
#64267=ORIENTED_EDGE('',*,*,#46592,.F.);
#64268=ORIENTED_EDGE('',*,*,#46810,.F.);
#64269=ORIENTED_EDGE('',*,*,#46811,.F.);
#64270=ORIENTED_EDGE('',*,*,#46812,.F.);
#64271=ORIENTED_EDGE('',*,*,#46588,.F.);
#64272=ORIENTED_EDGE('',*,*,#46813,.F.);
#64273=ORIENTED_EDGE('',*,*,#46814,.F.);
#64274=ORIENTED_EDGE('',*,*,#46815,.F.);
#64275=ORIENTED_EDGE('',*,*,#46584,.F.);
#64276=ORIENTED_EDGE('',*,*,#46816,.F.);
#64277=ORIENTED_EDGE('',*,*,#46817,.F.);
#64278=ORIENTED_EDGE('',*,*,#46818,.F.);
#64279=ORIENTED_EDGE('',*,*,#46580,.F.);
#64280=ORIENTED_EDGE('',*,*,#46819,.F.);
#64281=ORIENTED_EDGE('',*,*,#46820,.F.);
#64282=ORIENTED_EDGE('',*,*,#46821,.F.);
#64283=ORIENTED_EDGE('',*,*,#46576,.F.);
#64284=ORIENTED_EDGE('',*,*,#46822,.F.);
#64285=ORIENTED_EDGE('',*,*,#46823,.F.);
#64286=ORIENTED_EDGE('',*,*,#46824,.F.);
#64287=ORIENTED_EDGE('',*,*,#46572,.F.);
#64288=ORIENTED_EDGE('',*,*,#46825,.F.);
#64289=ORIENTED_EDGE('',*,*,#46826,.F.);
#64290=ORIENTED_EDGE('',*,*,#46827,.F.);
#64291=ORIENTED_EDGE('',*,*,#46568,.F.);
#64292=ORIENTED_EDGE('',*,*,#46828,.F.);
#64293=ORIENTED_EDGE('',*,*,#46829,.F.);
#64294=ORIENTED_EDGE('',*,*,#46830,.F.);
#64295=ORIENTED_EDGE('',*,*,#46564,.F.);
#64296=ORIENTED_EDGE('',*,*,#46831,.F.);
#64297=ORIENTED_EDGE('',*,*,#46832,.F.);
#64298=ORIENTED_EDGE('',*,*,#46833,.F.);
#64299=ORIENTED_EDGE('',*,*,#46560,.F.);
#64300=ORIENTED_EDGE('',*,*,#46834,.F.);
#64301=ORIENTED_EDGE('',*,*,#46835,.F.);
#64302=ORIENTED_EDGE('',*,*,#46836,.T.);
#64303=ORIENTED_EDGE('',*,*,#46837,.T.);
#64304=ORIENTED_EDGE('',*,*,#46836,.F.);
#64305=ORIENTED_EDGE('',*,*,#46838,.F.);
#64306=ORIENTED_EDGE('',*,*,#46839,.F.);
#64307=ORIENTED_EDGE('',*,*,#46556,.F.);
#64308=ORIENTED_EDGE('',*,*,#46840,.F.);
#64309=ORIENTED_EDGE('',*,*,#46841,.F.);
#64310=ORIENTED_EDGE('',*,*,#46842,.F.);
#64311=ORIENTED_EDGE('',*,*,#46552,.F.);
#64312=ORIENTED_EDGE('',*,*,#46843,.F.);
#64313=ORIENTED_EDGE('',*,*,#46844,.F.);
#64314=ORIENTED_EDGE('',*,*,#46845,.F.);
#64315=ORIENTED_EDGE('',*,*,#46548,.F.);
#64316=ORIENTED_EDGE('',*,*,#46846,.F.);
#64317=ORIENTED_EDGE('',*,*,#46847,.F.);
#64318=ORIENTED_EDGE('',*,*,#46848,.F.);
#64319=ORIENTED_EDGE('',*,*,#46544,.F.);
#64320=ORIENTED_EDGE('',*,*,#46849,.F.);
#64321=ORIENTED_EDGE('',*,*,#46850,.F.);
#64322=ORIENTED_EDGE('',*,*,#46851,.F.);
#64323=ORIENTED_EDGE('',*,*,#46540,.F.);
#64324=ORIENTED_EDGE('',*,*,#46852,.F.);
#64325=ORIENTED_EDGE('',*,*,#46853,.F.);
#64326=ORIENTED_EDGE('',*,*,#46854,.F.);
#64327=ORIENTED_EDGE('',*,*,#46536,.F.);
#64328=ORIENTED_EDGE('',*,*,#46855,.F.);
#64329=ORIENTED_EDGE('',*,*,#46856,.F.);
#64330=ORIENTED_EDGE('',*,*,#46857,.F.);
#64331=ORIENTED_EDGE('',*,*,#46532,.F.);
#64332=ORIENTED_EDGE('',*,*,#46858,.F.);
#64333=ORIENTED_EDGE('',*,*,#46859,.F.);
#64334=ORIENTED_EDGE('',*,*,#46860,.F.);
#64335=ORIENTED_EDGE('',*,*,#46528,.F.);
#64336=ORIENTED_EDGE('',*,*,#46861,.F.);
#64337=ORIENTED_EDGE('',*,*,#46862,.F.);
#64338=ORIENTED_EDGE('',*,*,#46863,.F.);
#64339=ORIENTED_EDGE('',*,*,#46524,.F.);
#64340=ORIENTED_EDGE('',*,*,#46864,.F.);
#64341=ORIENTED_EDGE('',*,*,#46865,.F.);
#64342=ORIENTED_EDGE('',*,*,#46866,.F.);
#64343=ORIENTED_EDGE('',*,*,#46520,.F.);
#64344=ORIENTED_EDGE('',*,*,#46867,.F.);
#64345=ORIENTED_EDGE('',*,*,#46868,.F.);
#64346=ORIENTED_EDGE('',*,*,#46869,.F.);
#64347=ORIENTED_EDGE('',*,*,#46516,.F.);
#64348=ORIENTED_EDGE('',*,*,#46870,.F.);
#64349=ORIENTED_EDGE('',*,*,#46871,.F.);
#64350=ORIENTED_EDGE('',*,*,#46872,.F.);
#64351=ORIENTED_EDGE('',*,*,#46512,.F.);
#64352=ORIENTED_EDGE('',*,*,#46873,.F.);
#64353=ORIENTED_EDGE('',*,*,#46874,.F.);
#64354=ORIENTED_EDGE('',*,*,#46875,.F.);
#64355=ORIENTED_EDGE('',*,*,#46508,.F.);
#64356=ORIENTED_EDGE('',*,*,#46876,.F.);
#64357=ORIENTED_EDGE('',*,*,#46877,.F.);
#64358=ORIENTED_EDGE('',*,*,#46878,.F.);
#64359=ORIENTED_EDGE('',*,*,#46504,.F.);
#64360=ORIENTED_EDGE('',*,*,#46879,.F.);
#64361=ORIENTED_EDGE('',*,*,#46880,.F.);
#64362=ORIENTED_EDGE('',*,*,#46881,.F.);
#64363=ORIENTED_EDGE('',*,*,#46500,.F.);
#64364=ORIENTED_EDGE('',*,*,#46882,.F.);
#64365=ORIENTED_EDGE('',*,*,#46883,.F.);
#64366=ORIENTED_EDGE('',*,*,#46884,.F.);
#64367=ORIENTED_EDGE('',*,*,#46496,.F.);
#64368=ORIENTED_EDGE('',*,*,#46885,.F.);
#64369=ORIENTED_EDGE('',*,*,#46886,.F.);
#64370=ORIENTED_EDGE('',*,*,#46887,.F.);
#64371=ORIENTED_EDGE('',*,*,#46492,.F.);
#64372=ORIENTED_EDGE('',*,*,#46888,.F.);
#64373=ORIENTED_EDGE('',*,*,#46889,.F.);
#64374=ORIENTED_EDGE('',*,*,#46890,.F.);
#64375=ORIENTED_EDGE('',*,*,#46488,.F.);
#64376=ORIENTED_EDGE('',*,*,#46891,.F.);
#64377=ORIENTED_EDGE('',*,*,#46892,.F.);
#64378=ORIENTED_EDGE('',*,*,#46893,.F.);
#64379=ORIENTED_EDGE('',*,*,#46484,.F.);
#64380=ORIENTED_EDGE('',*,*,#46894,.F.);
#64381=ORIENTED_EDGE('',*,*,#46895,.F.);
#64382=ORIENTED_EDGE('',*,*,#46896,.F.);
#64383=ORIENTED_EDGE('',*,*,#46480,.F.);
#64384=ORIENTED_EDGE('',*,*,#46897,.F.);
#64385=ORIENTED_EDGE('',*,*,#46898,.F.);
#64386=ORIENTED_EDGE('',*,*,#46899,.F.);
#64387=ORIENTED_EDGE('',*,*,#46476,.F.);
#64388=ORIENTED_EDGE('',*,*,#46900,.F.);
#64389=ORIENTED_EDGE('',*,*,#46901,.F.);
#64390=ORIENTED_EDGE('',*,*,#46902,.F.);
#64391=ORIENTED_EDGE('',*,*,#46472,.F.);
#64392=ORIENTED_EDGE('',*,*,#46903,.F.);
#64393=ORIENTED_EDGE('',*,*,#46904,.F.);
#64394=ORIENTED_EDGE('',*,*,#46905,.F.);
#64395=ORIENTED_EDGE('',*,*,#46468,.F.);
#64396=ORIENTED_EDGE('',*,*,#46906,.F.);
#64397=ORIENTED_EDGE('',*,*,#46907,.F.);
#64398=ORIENTED_EDGE('',*,*,#46908,.F.);
#64399=ORIENTED_EDGE('',*,*,#46464,.F.);
#64400=ORIENTED_EDGE('',*,*,#46909,.F.);
#64401=ORIENTED_EDGE('',*,*,#46910,.F.);
#64402=ORIENTED_EDGE('',*,*,#46911,.F.);
#64403=ORIENTED_EDGE('',*,*,#46460,.F.);
#64404=ORIENTED_EDGE('',*,*,#46912,.F.);
#64405=ORIENTED_EDGE('',*,*,#46913,.F.);
#64406=ORIENTED_EDGE('',*,*,#46914,.F.);
#64407=ORIENTED_EDGE('',*,*,#46456,.F.);
#64408=ORIENTED_EDGE('',*,*,#46915,.F.);
#64409=ORIENTED_EDGE('',*,*,#46916,.F.);
#64410=ORIENTED_EDGE('',*,*,#46917,.F.);
#64411=ORIENTED_EDGE('',*,*,#46452,.F.);
#64412=ORIENTED_EDGE('',*,*,#46918,.F.);
#64413=ORIENTED_EDGE('',*,*,#46919,.F.);
#64414=ORIENTED_EDGE('',*,*,#46920,.F.);
#64415=ORIENTED_EDGE('',*,*,#46448,.F.);
#64416=ORIENTED_EDGE('',*,*,#46921,.F.);
#64417=ORIENTED_EDGE('',*,*,#46922,.F.);
#64418=ORIENTED_EDGE('',*,*,#46923,.F.);
#64419=ORIENTED_EDGE('',*,*,#46444,.F.);
#64420=ORIENTED_EDGE('',*,*,#46924,.F.);
#64421=ORIENTED_EDGE('',*,*,#46925,.F.);
#64422=ORIENTED_EDGE('',*,*,#46926,.F.);
#64423=ORIENTED_EDGE('',*,*,#46440,.F.);
#64424=ORIENTED_EDGE('',*,*,#46927,.F.);
#64425=ORIENTED_EDGE('',*,*,#46928,.F.);
#64426=ORIENTED_EDGE('',*,*,#46929,.F.);
#64427=ORIENTED_EDGE('',*,*,#46436,.F.);
#64428=ORIENTED_EDGE('',*,*,#46930,.F.);
#64429=ORIENTED_EDGE('',*,*,#46931,.F.);
#64430=ORIENTED_EDGE('',*,*,#46932,.F.);
#64431=ORIENTED_EDGE('',*,*,#46432,.F.);
#64432=ORIENTED_EDGE('',*,*,#46933,.F.);
#64433=ORIENTED_EDGE('',*,*,#46934,.F.);
#64434=ORIENTED_EDGE('',*,*,#46935,.F.);
#64435=ORIENTED_EDGE('',*,*,#46428,.F.);
#64436=ORIENTED_EDGE('',*,*,#46936,.F.);
#64437=ORIENTED_EDGE('',*,*,#46937,.F.);
#64438=ORIENTED_EDGE('',*,*,#46938,.F.);
#64439=ORIENTED_EDGE('',*,*,#46424,.F.);
#64440=ORIENTED_EDGE('',*,*,#46939,.F.);
#64441=ORIENTED_EDGE('',*,*,#46940,.F.);
#64442=ORIENTED_EDGE('',*,*,#46941,.F.);
#64443=ORIENTED_EDGE('',*,*,#46420,.F.);
#64444=ORIENTED_EDGE('',*,*,#46942,.F.);
#64445=ORIENTED_EDGE('',*,*,#46711,.T.);
#64446=ORIENTED_EDGE('',*,*,#46943,.T.);
#64447=ORIENTED_EDGE('',*,*,#46944,.F.);
#64448=ORIENTED_EDGE('',*,*,#46945,.F.);
#64449=ORIENTED_EDGE('',*,*,#46562,.T.);
#64450=ORIENTED_EDGE('',*,*,#46946,.F.);
#64451=ORIENTED_EDGE('',*,*,#46947,.F.);
#64452=ORIENTED_EDGE('',*,*,#46948,.F.);
#64453=ORIENTED_EDGE('',*,*,#46566,.T.);
#64454=ORIENTED_EDGE('',*,*,#46949,.F.);
#64455=ORIENTED_EDGE('',*,*,#46950,.F.);
#64456=ORIENTED_EDGE('',*,*,#46951,.F.);
#64457=ORIENTED_EDGE('',*,*,#46570,.T.);
#64458=ORIENTED_EDGE('',*,*,#46952,.F.);
#64459=ORIENTED_EDGE('',*,*,#46953,.F.);
#64460=ORIENTED_EDGE('',*,*,#46954,.F.);
#64461=ORIENTED_EDGE('',*,*,#46574,.T.);
#64462=ORIENTED_EDGE('',*,*,#46955,.F.);
#64463=ORIENTED_EDGE('',*,*,#46956,.F.);
#64464=ORIENTED_EDGE('',*,*,#46957,.F.);
#64465=ORIENTED_EDGE('',*,*,#46578,.T.);
#64466=ORIENTED_EDGE('',*,*,#46958,.F.);
#64467=ORIENTED_EDGE('',*,*,#46959,.F.);
#64468=ORIENTED_EDGE('',*,*,#46960,.F.);
#64469=ORIENTED_EDGE('',*,*,#46582,.T.);
#64470=ORIENTED_EDGE('',*,*,#46961,.F.);
#64471=ORIENTED_EDGE('',*,*,#46962,.F.);
#64472=ORIENTED_EDGE('',*,*,#46963,.F.);
#64473=ORIENTED_EDGE('',*,*,#46586,.T.);
#64474=ORIENTED_EDGE('',*,*,#46964,.F.);
#64475=ORIENTED_EDGE('',*,*,#46965,.F.);
#64476=ORIENTED_EDGE('',*,*,#46966,.F.);
#64477=ORIENTED_EDGE('',*,*,#46590,.T.);
#64478=ORIENTED_EDGE('',*,*,#46967,.F.);
#64479=ORIENTED_EDGE('',*,*,#46968,.F.);
#64480=ORIENTED_EDGE('',*,*,#46969,.F.);
#64481=ORIENTED_EDGE('',*,*,#46594,.T.);
#64482=ORIENTED_EDGE('',*,*,#46970,.F.);
#64483=ORIENTED_EDGE('',*,*,#46971,.F.);
#64484=ORIENTED_EDGE('',*,*,#46972,.F.);
#64485=ORIENTED_EDGE('',*,*,#46598,.T.);
#64486=ORIENTED_EDGE('',*,*,#46973,.F.);
#64487=ORIENTED_EDGE('',*,*,#46974,.F.);
#64488=ORIENTED_EDGE('',*,*,#46975,.F.);
#64489=ORIENTED_EDGE('',*,*,#46602,.T.);
#64490=ORIENTED_EDGE('',*,*,#46976,.F.);
#64491=ORIENTED_EDGE('',*,*,#46977,.F.);
#64492=ORIENTED_EDGE('',*,*,#46978,.F.);
#64493=ORIENTED_EDGE('',*,*,#46606,.T.);
#64494=ORIENTED_EDGE('',*,*,#46979,.F.);
#64495=ORIENTED_EDGE('',*,*,#46980,.F.);
#64496=ORIENTED_EDGE('',*,*,#46981,.F.);
#64497=ORIENTED_EDGE('',*,*,#46610,.T.);
#64498=ORIENTED_EDGE('',*,*,#46982,.F.);
#64499=ORIENTED_EDGE('',*,*,#46983,.F.);
#64500=ORIENTED_EDGE('',*,*,#46984,.F.);
#64501=ORIENTED_EDGE('',*,*,#46614,.T.);
#64502=ORIENTED_EDGE('',*,*,#46985,.F.);
#64503=ORIENTED_EDGE('',*,*,#46986,.F.);
#64504=ORIENTED_EDGE('',*,*,#46987,.F.);
#64505=ORIENTED_EDGE('',*,*,#46618,.T.);
#64506=ORIENTED_EDGE('',*,*,#46988,.F.);
#64507=ORIENTED_EDGE('',*,*,#46989,.F.);
#64508=ORIENTED_EDGE('',*,*,#46990,.F.);
#64509=ORIENTED_EDGE('',*,*,#46622,.T.);
#64510=ORIENTED_EDGE('',*,*,#46991,.F.);
#64511=ORIENTED_EDGE('',*,*,#46992,.F.);
#64512=ORIENTED_EDGE('',*,*,#46993,.F.);
#64513=ORIENTED_EDGE('',*,*,#46626,.T.);
#64514=ORIENTED_EDGE('',*,*,#46994,.F.);
#64515=ORIENTED_EDGE('',*,*,#46995,.F.);
#64516=ORIENTED_EDGE('',*,*,#46996,.F.);
#64517=ORIENTED_EDGE('',*,*,#46630,.T.);
#64518=ORIENTED_EDGE('',*,*,#46997,.F.);
#64519=ORIENTED_EDGE('',*,*,#46998,.F.);
#64520=ORIENTED_EDGE('',*,*,#46999,.F.);
#64521=ORIENTED_EDGE('',*,*,#46634,.T.);
#64522=ORIENTED_EDGE('',*,*,#47000,.F.);
#64523=ORIENTED_EDGE('',*,*,#47001,.F.);
#64524=ORIENTED_EDGE('',*,*,#47002,.F.);
#64525=ORIENTED_EDGE('',*,*,#46638,.T.);
#64526=ORIENTED_EDGE('',*,*,#47003,.F.);
#64527=ORIENTED_EDGE('',*,*,#47004,.F.);
#64528=ORIENTED_EDGE('',*,*,#47005,.F.);
#64529=ORIENTED_EDGE('',*,*,#46642,.T.);
#64530=ORIENTED_EDGE('',*,*,#47006,.F.);
#64531=ORIENTED_EDGE('',*,*,#47007,.F.);
#64532=ORIENTED_EDGE('',*,*,#47008,.F.);
#64533=ORIENTED_EDGE('',*,*,#46646,.T.);
#64534=ORIENTED_EDGE('',*,*,#47009,.F.);
#64535=ORIENTED_EDGE('',*,*,#47010,.F.);
#64536=ORIENTED_EDGE('',*,*,#47011,.F.);
#64537=ORIENTED_EDGE('',*,*,#46650,.T.);
#64538=ORIENTED_EDGE('',*,*,#47012,.F.);
#64539=ORIENTED_EDGE('',*,*,#47013,.F.);
#64540=ORIENTED_EDGE('',*,*,#47014,.F.);
#64541=ORIENTED_EDGE('',*,*,#46654,.T.);
#64542=ORIENTED_EDGE('',*,*,#47015,.F.);
#64543=ORIENTED_EDGE('',*,*,#47016,.F.);
#64544=ORIENTED_EDGE('',*,*,#47017,.F.);
#64545=ORIENTED_EDGE('',*,*,#46658,.T.);
#64546=ORIENTED_EDGE('',*,*,#47018,.F.);
#64547=ORIENTED_EDGE('',*,*,#47019,.F.);
#64548=ORIENTED_EDGE('',*,*,#47020,.F.);
#64549=ORIENTED_EDGE('',*,*,#46662,.T.);
#64550=ORIENTED_EDGE('',*,*,#47021,.F.);
#64551=ORIENTED_EDGE('',*,*,#47022,.F.);
#64552=ORIENTED_EDGE('',*,*,#47023,.F.);
#64553=ORIENTED_EDGE('',*,*,#46666,.T.);
#64554=ORIENTED_EDGE('',*,*,#47024,.F.);
#64555=ORIENTED_EDGE('',*,*,#47025,.F.);
#64556=ORIENTED_EDGE('',*,*,#47026,.F.);
#64557=ORIENTED_EDGE('',*,*,#46670,.T.);
#64558=ORIENTED_EDGE('',*,*,#47027,.F.);
#64559=ORIENTED_EDGE('',*,*,#47028,.F.);
#64560=ORIENTED_EDGE('',*,*,#47029,.F.);
#64561=ORIENTED_EDGE('',*,*,#46674,.T.);
#64562=ORIENTED_EDGE('',*,*,#47030,.F.);
#64563=ORIENTED_EDGE('',*,*,#47031,.F.);
#64564=ORIENTED_EDGE('',*,*,#47032,.F.);
#64565=ORIENTED_EDGE('',*,*,#46678,.T.);
#64566=ORIENTED_EDGE('',*,*,#47033,.F.);
#64567=ORIENTED_EDGE('',*,*,#47034,.F.);
#64568=ORIENTED_EDGE('',*,*,#47035,.F.);
#64569=ORIENTED_EDGE('',*,*,#46682,.T.);
#64570=ORIENTED_EDGE('',*,*,#47036,.F.);
#64571=ORIENTED_EDGE('',*,*,#47037,.F.);
#64572=ORIENTED_EDGE('',*,*,#47038,.F.);
#64573=ORIENTED_EDGE('',*,*,#46686,.T.);
#64574=ORIENTED_EDGE('',*,*,#47039,.F.);
#64575=ORIENTED_EDGE('',*,*,#47040,.F.);
#64576=ORIENTED_EDGE('',*,*,#47041,.F.);
#64577=ORIENTED_EDGE('',*,*,#46690,.T.);
#64578=ORIENTED_EDGE('',*,*,#47042,.F.);
#64579=ORIENTED_EDGE('',*,*,#47043,.F.);
#64580=ORIENTED_EDGE('',*,*,#47044,.F.);
#64581=ORIENTED_EDGE('',*,*,#46694,.T.);
#64582=ORIENTED_EDGE('',*,*,#47045,.F.);
#64583=ORIENTED_EDGE('',*,*,#47046,.F.);
#64584=ORIENTED_EDGE('',*,*,#47047,.F.);
#64585=ORIENTED_EDGE('',*,*,#46698,.T.);
#64586=ORIENTED_EDGE('',*,*,#47048,.F.);
#64587=ORIENTED_EDGE('',*,*,#47049,.F.);
#64588=ORIENTED_EDGE('',*,*,#47050,.F.);
#64589=ORIENTED_EDGE('',*,*,#46422,.T.);
#64590=ORIENTED_EDGE('',*,*,#47051,.F.);
#64591=ORIENTED_EDGE('',*,*,#47052,.F.);
#64592=ORIENTED_EDGE('',*,*,#47053,.F.);
#64593=ORIENTED_EDGE('',*,*,#46426,.T.);
#64594=ORIENTED_EDGE('',*,*,#47054,.F.);
#64595=ORIENTED_EDGE('',*,*,#47055,.F.);
#64596=ORIENTED_EDGE('',*,*,#47056,.F.);
#64597=ORIENTED_EDGE('',*,*,#46430,.T.);
#64598=ORIENTED_EDGE('',*,*,#47057,.F.);
#64599=ORIENTED_EDGE('',*,*,#47058,.F.);
#64600=ORIENTED_EDGE('',*,*,#47059,.F.);
#64601=ORIENTED_EDGE('',*,*,#46434,.T.);
#64602=ORIENTED_EDGE('',*,*,#47060,.F.);
#64603=ORIENTED_EDGE('',*,*,#47061,.F.);
#64604=ORIENTED_EDGE('',*,*,#47062,.F.);
#64605=ORIENTED_EDGE('',*,*,#46438,.T.);
#64606=ORIENTED_EDGE('',*,*,#47063,.F.);
#64607=ORIENTED_EDGE('',*,*,#47064,.F.);
#64608=ORIENTED_EDGE('',*,*,#47065,.F.);
#64609=ORIENTED_EDGE('',*,*,#46442,.T.);
#64610=ORIENTED_EDGE('',*,*,#47066,.F.);
#64611=ORIENTED_EDGE('',*,*,#47067,.F.);
#64612=ORIENTED_EDGE('',*,*,#47068,.F.);
#64613=ORIENTED_EDGE('',*,*,#46446,.T.);
#64614=ORIENTED_EDGE('',*,*,#47069,.F.);
#64615=ORIENTED_EDGE('',*,*,#47070,.F.);
#64616=ORIENTED_EDGE('',*,*,#47071,.F.);
#64617=ORIENTED_EDGE('',*,*,#46450,.T.);
#64618=ORIENTED_EDGE('',*,*,#47072,.F.);
#64619=ORIENTED_EDGE('',*,*,#47073,.F.);
#64620=ORIENTED_EDGE('',*,*,#47074,.F.);
#64621=ORIENTED_EDGE('',*,*,#46454,.T.);
#64622=ORIENTED_EDGE('',*,*,#47075,.F.);
#64623=ORIENTED_EDGE('',*,*,#47076,.F.);
#64624=ORIENTED_EDGE('',*,*,#47077,.F.);
#64625=ORIENTED_EDGE('',*,*,#46458,.T.);
#64626=ORIENTED_EDGE('',*,*,#47078,.F.);
#64627=ORIENTED_EDGE('',*,*,#47079,.F.);
#64628=ORIENTED_EDGE('',*,*,#47080,.F.);
#64629=ORIENTED_EDGE('',*,*,#46462,.T.);
#64630=ORIENTED_EDGE('',*,*,#47081,.F.);
#64631=ORIENTED_EDGE('',*,*,#47082,.F.);
#64632=ORIENTED_EDGE('',*,*,#47083,.F.);
#64633=ORIENTED_EDGE('',*,*,#46466,.T.);
#64634=ORIENTED_EDGE('',*,*,#47084,.F.);
#64635=ORIENTED_EDGE('',*,*,#47085,.F.);
#64636=ORIENTED_EDGE('',*,*,#47086,.F.);
#64637=ORIENTED_EDGE('',*,*,#46470,.T.);
#64638=ORIENTED_EDGE('',*,*,#47087,.F.);
#64639=ORIENTED_EDGE('',*,*,#47088,.F.);
#64640=ORIENTED_EDGE('',*,*,#47089,.F.);
#64641=ORIENTED_EDGE('',*,*,#46474,.T.);
#64642=ORIENTED_EDGE('',*,*,#47090,.F.);
#64643=ORIENTED_EDGE('',*,*,#47091,.F.);
#64644=ORIENTED_EDGE('',*,*,#47092,.F.);
#64645=ORIENTED_EDGE('',*,*,#46478,.T.);
#64646=ORIENTED_EDGE('',*,*,#47093,.F.);
#64647=ORIENTED_EDGE('',*,*,#47094,.F.);
#64648=ORIENTED_EDGE('',*,*,#47095,.F.);
#64649=ORIENTED_EDGE('',*,*,#46482,.T.);
#64650=ORIENTED_EDGE('',*,*,#47096,.F.);
#64651=ORIENTED_EDGE('',*,*,#47097,.F.);
#64652=ORIENTED_EDGE('',*,*,#47098,.F.);
#64653=ORIENTED_EDGE('',*,*,#46486,.T.);
#64654=ORIENTED_EDGE('',*,*,#47099,.F.);
#64655=ORIENTED_EDGE('',*,*,#47100,.F.);
#64656=ORIENTED_EDGE('',*,*,#47101,.F.);
#64657=ORIENTED_EDGE('',*,*,#46490,.T.);
#64658=ORIENTED_EDGE('',*,*,#47102,.F.);
#64659=ORIENTED_EDGE('',*,*,#47103,.F.);
#64660=ORIENTED_EDGE('',*,*,#47104,.F.);
#64661=ORIENTED_EDGE('',*,*,#46494,.T.);
#64662=ORIENTED_EDGE('',*,*,#47105,.F.);
#64663=ORIENTED_EDGE('',*,*,#47106,.F.);
#64664=ORIENTED_EDGE('',*,*,#47107,.F.);
#64665=ORIENTED_EDGE('',*,*,#46498,.T.);
#64666=ORIENTED_EDGE('',*,*,#47108,.F.);
#64667=ORIENTED_EDGE('',*,*,#47109,.F.);
#64668=ORIENTED_EDGE('',*,*,#47110,.F.);
#64669=ORIENTED_EDGE('',*,*,#46502,.T.);
#64670=ORIENTED_EDGE('',*,*,#47111,.F.);
#64671=ORIENTED_EDGE('',*,*,#47112,.F.);
#64672=ORIENTED_EDGE('',*,*,#47113,.F.);
#64673=ORIENTED_EDGE('',*,*,#46506,.T.);
#64674=ORIENTED_EDGE('',*,*,#47114,.F.);
#64675=ORIENTED_EDGE('',*,*,#47115,.F.);
#64676=ORIENTED_EDGE('',*,*,#47116,.F.);
#64677=ORIENTED_EDGE('',*,*,#46510,.T.);
#64678=ORIENTED_EDGE('',*,*,#47117,.F.);
#64679=ORIENTED_EDGE('',*,*,#47118,.F.);
#64680=ORIENTED_EDGE('',*,*,#47119,.F.);
#64681=ORIENTED_EDGE('',*,*,#46514,.T.);
#64682=ORIENTED_EDGE('',*,*,#47120,.F.);
#64683=ORIENTED_EDGE('',*,*,#47121,.F.);
#64684=ORIENTED_EDGE('',*,*,#47122,.F.);
#64685=ORIENTED_EDGE('',*,*,#46518,.T.);
#64686=ORIENTED_EDGE('',*,*,#47123,.F.);
#64687=ORIENTED_EDGE('',*,*,#47124,.F.);
#64688=ORIENTED_EDGE('',*,*,#47125,.F.);
#64689=ORIENTED_EDGE('',*,*,#46522,.T.);
#64690=ORIENTED_EDGE('',*,*,#47126,.F.);
#64691=ORIENTED_EDGE('',*,*,#47127,.F.);
#64692=ORIENTED_EDGE('',*,*,#47128,.F.);
#64693=ORIENTED_EDGE('',*,*,#46526,.T.);
#64694=ORIENTED_EDGE('',*,*,#47129,.F.);
#64695=ORIENTED_EDGE('',*,*,#47130,.F.);
#64696=ORIENTED_EDGE('',*,*,#47131,.F.);
#64697=ORIENTED_EDGE('',*,*,#46530,.T.);
#64698=ORIENTED_EDGE('',*,*,#47132,.F.);
#64699=ORIENTED_EDGE('',*,*,#47133,.F.);
#64700=ORIENTED_EDGE('',*,*,#47134,.F.);
#64701=ORIENTED_EDGE('',*,*,#46534,.T.);
#64702=ORIENTED_EDGE('',*,*,#47135,.F.);
#64703=ORIENTED_EDGE('',*,*,#47136,.F.);
#64704=ORIENTED_EDGE('',*,*,#47137,.F.);
#64705=ORIENTED_EDGE('',*,*,#46538,.T.);
#64706=ORIENTED_EDGE('',*,*,#47138,.F.);
#64707=ORIENTED_EDGE('',*,*,#47139,.F.);
#64708=ORIENTED_EDGE('',*,*,#47140,.F.);
#64709=ORIENTED_EDGE('',*,*,#46542,.T.);
#64710=ORIENTED_EDGE('',*,*,#47141,.F.);
#64711=ORIENTED_EDGE('',*,*,#47142,.F.);
#64712=ORIENTED_EDGE('',*,*,#47143,.F.);
#64713=ORIENTED_EDGE('',*,*,#46546,.T.);
#64714=ORIENTED_EDGE('',*,*,#47144,.F.);
#64715=ORIENTED_EDGE('',*,*,#47145,.F.);
#64716=ORIENTED_EDGE('',*,*,#47146,.F.);
#64717=ORIENTED_EDGE('',*,*,#46550,.T.);
#64718=ORIENTED_EDGE('',*,*,#47147,.F.);
#64719=ORIENTED_EDGE('',*,*,#47148,.F.);
#64720=ORIENTED_EDGE('',*,*,#47149,.F.);
#64721=ORIENTED_EDGE('',*,*,#46554,.T.);
#64722=ORIENTED_EDGE('',*,*,#47150,.F.);
#64723=ORIENTED_EDGE('',*,*,#47151,.F.);
#64724=ORIENTED_EDGE('',*,*,#47152,.F.);
#64725=ORIENTED_EDGE('',*,*,#46558,.T.);
#64726=ORIENTED_EDGE('',*,*,#47153,.F.);
#64727=ORIENTED_EDGE('',*,*,#47154,.F.);
#64728=ORIENTED_EDGE('',*,*,#46943,.F.);
#64729=ORIENTED_EDGE('',*,*,#46714,.T.);
#64730=ORIENTED_EDGE('',*,*,#46721,.T.);
#64731=ORIENTED_EDGE('',*,*,#47155,.T.);
#64732=ORIENTED_EDGE('',*,*,#47156,.T.);
#64733=ORIENTED_EDGE('',*,*,#47155,.F.);
#64734=ORIENTED_EDGE('',*,*,#46724,.T.);
#64735=ORIENTED_EDGE('',*,*,#46699,.T.);
#64736=ORIENTED_EDGE('',*,*,#47157,.T.);
#64737=ORIENTED_EDGE('',*,*,#46725,.T.);
#64738=ORIENTED_EDGE('',*,*,#47157,.F.);
#64739=ORIENTED_EDGE('',*,*,#46702,.T.);
#64740=ORIENTED_EDGE('',*,*,#46723,.T.);
#64741=ORIENTED_EDGE('',*,*,#46727,.T.);
#64742=ORIENTED_EDGE('',*,*,#46713,.T.);
#64743=ORIENTED_EDGE('',*,*,#47156,.F.);
#64744=ORIENTED_EDGE('',*,*,#46720,.T.);
#64745=ORIENTED_EDGE('',*,*,#46717,.T.);
#64746=ORIENTED_EDGE('',*,*,#46837,.F.);
#64747=ORIENTED_EDGE('',*,*,#46701,.T.);
#64748=ORIENTED_EDGE('',*,*,#46709,.T.);
#64749=ORIENTED_EDGE('',*,*,#46705,.T.);
#64750=ORIENTED_EDGE('',*,*,#47048,.T.);
#64751=ORIENTED_EDGE('',*,*,#46697,.T.);
#64752=ORIENTED_EDGE('',*,*,#46731,.T.);
#64753=ORIENTED_EDGE('',*,*,#47158,.T.);
#64754=ORIENTED_EDGE('',*,*,#47049,.T.);
#64755=ORIENTED_EDGE('',*,*,#47158,.F.);
#64756=ORIENTED_EDGE('',*,*,#46730,.T.);
#64757=ORIENTED_EDGE('',*,*,#47159,.T.);
#64758=ORIENTED_EDGE('',*,*,#47050,.T.);
#64759=ORIENTED_EDGE('',*,*,#47159,.F.);
#64760=ORIENTED_EDGE('',*,*,#46942,.T.);
#64761=ORIENTED_EDGE('',*,*,#46419,.T.);
#64762=ORIENTED_EDGE('',*,*,#47051,.T.);
#64763=ORIENTED_EDGE('',*,*,#46421,.T.);
#64764=ORIENTED_EDGE('',*,*,#46941,.T.);
#64765=ORIENTED_EDGE('',*,*,#47160,.T.);
#64766=ORIENTED_EDGE('',*,*,#47052,.T.);
#64767=ORIENTED_EDGE('',*,*,#47160,.F.);
#64768=ORIENTED_EDGE('',*,*,#46940,.T.);
#64769=ORIENTED_EDGE('',*,*,#47161,.T.);
#64770=ORIENTED_EDGE('',*,*,#47053,.T.);
#64771=ORIENTED_EDGE('',*,*,#47161,.F.);
#64772=ORIENTED_EDGE('',*,*,#46939,.T.);
#64773=ORIENTED_EDGE('',*,*,#46423,.T.);
#64774=ORIENTED_EDGE('',*,*,#47054,.T.);
#64775=ORIENTED_EDGE('',*,*,#46425,.T.);
#64776=ORIENTED_EDGE('',*,*,#46938,.T.);
#64777=ORIENTED_EDGE('',*,*,#47162,.T.);
#64778=ORIENTED_EDGE('',*,*,#47055,.T.);
#64779=ORIENTED_EDGE('',*,*,#47162,.F.);
#64780=ORIENTED_EDGE('',*,*,#46937,.T.);
#64781=ORIENTED_EDGE('',*,*,#47163,.T.);
#64782=ORIENTED_EDGE('',*,*,#47056,.T.);
#64783=ORIENTED_EDGE('',*,*,#47163,.F.);
#64784=ORIENTED_EDGE('',*,*,#46936,.T.);
#64785=ORIENTED_EDGE('',*,*,#46427,.T.);
#64786=ORIENTED_EDGE('',*,*,#47057,.T.);
#64787=ORIENTED_EDGE('',*,*,#46429,.T.);
#64788=ORIENTED_EDGE('',*,*,#46935,.T.);
#64789=ORIENTED_EDGE('',*,*,#47164,.T.);
#64790=ORIENTED_EDGE('',*,*,#47058,.T.);
#64791=ORIENTED_EDGE('',*,*,#47164,.F.);
#64792=ORIENTED_EDGE('',*,*,#46934,.T.);
#64793=ORIENTED_EDGE('',*,*,#47165,.T.);
#64794=ORIENTED_EDGE('',*,*,#47059,.T.);
#64795=ORIENTED_EDGE('',*,*,#47165,.F.);
#64796=ORIENTED_EDGE('',*,*,#46933,.T.);
#64797=ORIENTED_EDGE('',*,*,#46431,.T.);
#64798=ORIENTED_EDGE('',*,*,#47060,.T.);
#64799=ORIENTED_EDGE('',*,*,#46433,.T.);
#64800=ORIENTED_EDGE('',*,*,#46932,.T.);
#64801=ORIENTED_EDGE('',*,*,#47166,.T.);
#64802=ORIENTED_EDGE('',*,*,#47061,.T.);
#64803=ORIENTED_EDGE('',*,*,#47166,.F.);
#64804=ORIENTED_EDGE('',*,*,#46931,.T.);
#64805=ORIENTED_EDGE('',*,*,#47167,.T.);
#64806=ORIENTED_EDGE('',*,*,#47062,.T.);
#64807=ORIENTED_EDGE('',*,*,#47167,.F.);
#64808=ORIENTED_EDGE('',*,*,#46930,.T.);
#64809=ORIENTED_EDGE('',*,*,#46435,.T.);
#64810=ORIENTED_EDGE('',*,*,#47063,.T.);
#64811=ORIENTED_EDGE('',*,*,#46437,.T.);
#64812=ORIENTED_EDGE('',*,*,#46929,.T.);
#64813=ORIENTED_EDGE('',*,*,#47168,.T.);
#64814=ORIENTED_EDGE('',*,*,#47064,.T.);
#64815=ORIENTED_EDGE('',*,*,#47168,.F.);
#64816=ORIENTED_EDGE('',*,*,#46928,.T.);
#64817=ORIENTED_EDGE('',*,*,#47169,.T.);
#64818=ORIENTED_EDGE('',*,*,#47065,.T.);
#64819=ORIENTED_EDGE('',*,*,#47169,.F.);
#64820=ORIENTED_EDGE('',*,*,#46927,.T.);
#64821=ORIENTED_EDGE('',*,*,#46439,.T.);
#64822=ORIENTED_EDGE('',*,*,#47066,.T.);
#64823=ORIENTED_EDGE('',*,*,#46441,.T.);
#64824=ORIENTED_EDGE('',*,*,#46926,.T.);
#64825=ORIENTED_EDGE('',*,*,#47170,.T.);
#64826=ORIENTED_EDGE('',*,*,#47067,.T.);
#64827=ORIENTED_EDGE('',*,*,#47170,.F.);
#64828=ORIENTED_EDGE('',*,*,#46925,.T.);
#64829=ORIENTED_EDGE('',*,*,#47171,.T.);
#64830=ORIENTED_EDGE('',*,*,#47068,.T.);
#64831=ORIENTED_EDGE('',*,*,#47171,.F.);
#64832=ORIENTED_EDGE('',*,*,#46924,.T.);
#64833=ORIENTED_EDGE('',*,*,#46443,.T.);
#64834=ORIENTED_EDGE('',*,*,#47069,.T.);
#64835=ORIENTED_EDGE('',*,*,#46445,.T.);
#64836=ORIENTED_EDGE('',*,*,#46923,.T.);
#64837=ORIENTED_EDGE('',*,*,#47172,.T.);
#64838=ORIENTED_EDGE('',*,*,#47070,.T.);
#64839=ORIENTED_EDGE('',*,*,#47172,.F.);
#64840=ORIENTED_EDGE('',*,*,#46922,.T.);
#64841=ORIENTED_EDGE('',*,*,#47173,.T.);
#64842=ORIENTED_EDGE('',*,*,#47071,.T.);
#64843=ORIENTED_EDGE('',*,*,#47173,.F.);
#64844=ORIENTED_EDGE('',*,*,#46921,.T.);
#64845=ORIENTED_EDGE('',*,*,#46447,.T.);
#64846=ORIENTED_EDGE('',*,*,#47072,.T.);
#64847=ORIENTED_EDGE('',*,*,#46449,.T.);
#64848=ORIENTED_EDGE('',*,*,#46920,.T.);
#64849=ORIENTED_EDGE('',*,*,#47174,.T.);
#64850=ORIENTED_EDGE('',*,*,#47073,.T.);
#64851=ORIENTED_EDGE('',*,*,#47174,.F.);
#64852=ORIENTED_EDGE('',*,*,#46919,.T.);
#64853=ORIENTED_EDGE('',*,*,#47175,.T.);
#64854=ORIENTED_EDGE('',*,*,#47074,.T.);
#64855=ORIENTED_EDGE('',*,*,#47175,.F.);
#64856=ORIENTED_EDGE('',*,*,#46918,.T.);
#64857=ORIENTED_EDGE('',*,*,#46451,.T.);
#64858=ORIENTED_EDGE('',*,*,#47075,.T.);
#64859=ORIENTED_EDGE('',*,*,#46453,.T.);
#64860=ORIENTED_EDGE('',*,*,#46917,.T.);
#64861=ORIENTED_EDGE('',*,*,#47176,.T.);
#64862=ORIENTED_EDGE('',*,*,#47076,.T.);
#64863=ORIENTED_EDGE('',*,*,#47176,.F.);
#64864=ORIENTED_EDGE('',*,*,#46916,.T.);
#64865=ORIENTED_EDGE('',*,*,#47177,.T.);
#64866=ORIENTED_EDGE('',*,*,#47077,.T.);
#64867=ORIENTED_EDGE('',*,*,#47177,.F.);
#64868=ORIENTED_EDGE('',*,*,#46915,.T.);
#64869=ORIENTED_EDGE('',*,*,#46455,.T.);
#64870=ORIENTED_EDGE('',*,*,#47078,.T.);
#64871=ORIENTED_EDGE('',*,*,#46457,.T.);
#64872=ORIENTED_EDGE('',*,*,#46914,.T.);
#64873=ORIENTED_EDGE('',*,*,#47178,.T.);
#64874=ORIENTED_EDGE('',*,*,#47079,.T.);
#64875=ORIENTED_EDGE('',*,*,#47178,.F.);
#64876=ORIENTED_EDGE('',*,*,#46913,.T.);
#64877=ORIENTED_EDGE('',*,*,#47179,.T.);
#64878=ORIENTED_EDGE('',*,*,#47080,.T.);
#64879=ORIENTED_EDGE('',*,*,#47179,.F.);
#64880=ORIENTED_EDGE('',*,*,#46912,.T.);
#64881=ORIENTED_EDGE('',*,*,#46459,.T.);
#64882=ORIENTED_EDGE('',*,*,#47081,.T.);
#64883=ORIENTED_EDGE('',*,*,#46461,.T.);
#64884=ORIENTED_EDGE('',*,*,#46911,.T.);
#64885=ORIENTED_EDGE('',*,*,#47180,.T.);
#64886=ORIENTED_EDGE('',*,*,#47082,.T.);
#64887=ORIENTED_EDGE('',*,*,#47180,.F.);
#64888=ORIENTED_EDGE('',*,*,#46910,.T.);
#64889=ORIENTED_EDGE('',*,*,#47181,.T.);
#64890=ORIENTED_EDGE('',*,*,#47083,.T.);
#64891=ORIENTED_EDGE('',*,*,#47181,.F.);
#64892=ORIENTED_EDGE('',*,*,#46909,.T.);
#64893=ORIENTED_EDGE('',*,*,#46463,.T.);
#64894=ORIENTED_EDGE('',*,*,#47084,.T.);
#64895=ORIENTED_EDGE('',*,*,#46465,.T.);
#64896=ORIENTED_EDGE('',*,*,#46908,.T.);
#64897=ORIENTED_EDGE('',*,*,#47182,.T.);
#64898=ORIENTED_EDGE('',*,*,#47085,.T.);
#64899=ORIENTED_EDGE('',*,*,#47182,.F.);
#64900=ORIENTED_EDGE('',*,*,#46907,.T.);
#64901=ORIENTED_EDGE('',*,*,#47183,.T.);
#64902=ORIENTED_EDGE('',*,*,#47086,.T.);
#64903=ORIENTED_EDGE('',*,*,#47183,.F.);
#64904=ORIENTED_EDGE('',*,*,#46906,.T.);
#64905=ORIENTED_EDGE('',*,*,#46467,.T.);
#64906=ORIENTED_EDGE('',*,*,#47087,.T.);
#64907=ORIENTED_EDGE('',*,*,#46469,.T.);
#64908=ORIENTED_EDGE('',*,*,#46905,.T.);
#64909=ORIENTED_EDGE('',*,*,#47184,.T.);
#64910=ORIENTED_EDGE('',*,*,#47088,.T.);
#64911=ORIENTED_EDGE('',*,*,#47184,.F.);
#64912=ORIENTED_EDGE('',*,*,#46904,.T.);
#64913=ORIENTED_EDGE('',*,*,#47185,.T.);
#64914=ORIENTED_EDGE('',*,*,#47089,.T.);
#64915=ORIENTED_EDGE('',*,*,#47185,.F.);
#64916=ORIENTED_EDGE('',*,*,#46903,.T.);
#64917=ORIENTED_EDGE('',*,*,#46471,.T.);
#64918=ORIENTED_EDGE('',*,*,#47090,.T.);
#64919=ORIENTED_EDGE('',*,*,#46473,.T.);
#64920=ORIENTED_EDGE('',*,*,#46902,.T.);
#64921=ORIENTED_EDGE('',*,*,#47186,.T.);
#64922=ORIENTED_EDGE('',*,*,#47091,.T.);
#64923=ORIENTED_EDGE('',*,*,#47186,.F.);
#64924=ORIENTED_EDGE('',*,*,#46901,.T.);
#64925=ORIENTED_EDGE('',*,*,#47187,.T.);
#64926=ORIENTED_EDGE('',*,*,#47092,.T.);
#64927=ORIENTED_EDGE('',*,*,#47187,.F.);
#64928=ORIENTED_EDGE('',*,*,#46900,.T.);
#64929=ORIENTED_EDGE('',*,*,#46475,.T.);
#64930=ORIENTED_EDGE('',*,*,#47093,.T.);
#64931=ORIENTED_EDGE('',*,*,#46477,.T.);
#64932=ORIENTED_EDGE('',*,*,#46899,.T.);
#64933=ORIENTED_EDGE('',*,*,#47188,.T.);
#64934=ORIENTED_EDGE('',*,*,#47094,.T.);
#64935=ORIENTED_EDGE('',*,*,#47188,.F.);
#64936=ORIENTED_EDGE('',*,*,#46898,.T.);
#64937=ORIENTED_EDGE('',*,*,#47189,.T.);
#64938=ORIENTED_EDGE('',*,*,#47095,.T.);
#64939=ORIENTED_EDGE('',*,*,#47189,.F.);
#64940=ORIENTED_EDGE('',*,*,#46897,.T.);
#64941=ORIENTED_EDGE('',*,*,#46479,.T.);
#64942=ORIENTED_EDGE('',*,*,#47096,.T.);
#64943=ORIENTED_EDGE('',*,*,#46481,.T.);
#64944=ORIENTED_EDGE('',*,*,#46896,.T.);
#64945=ORIENTED_EDGE('',*,*,#47190,.T.);
#64946=ORIENTED_EDGE('',*,*,#47097,.T.);
#64947=ORIENTED_EDGE('',*,*,#47190,.F.);
#64948=ORIENTED_EDGE('',*,*,#46895,.T.);
#64949=ORIENTED_EDGE('',*,*,#47191,.T.);
#64950=ORIENTED_EDGE('',*,*,#47098,.T.);
#64951=ORIENTED_EDGE('',*,*,#47191,.F.);
#64952=ORIENTED_EDGE('',*,*,#46894,.T.);
#64953=ORIENTED_EDGE('',*,*,#46483,.T.);
#64954=ORIENTED_EDGE('',*,*,#47099,.T.);
#64955=ORIENTED_EDGE('',*,*,#46485,.T.);
#64956=ORIENTED_EDGE('',*,*,#46893,.T.);
#64957=ORIENTED_EDGE('',*,*,#47192,.T.);
#64958=ORIENTED_EDGE('',*,*,#47100,.T.);
#64959=ORIENTED_EDGE('',*,*,#47192,.F.);
#64960=ORIENTED_EDGE('',*,*,#46892,.T.);
#64961=ORIENTED_EDGE('',*,*,#47193,.T.);
#64962=ORIENTED_EDGE('',*,*,#47101,.T.);
#64963=ORIENTED_EDGE('',*,*,#47193,.F.);
#64964=ORIENTED_EDGE('',*,*,#46891,.T.);
#64965=ORIENTED_EDGE('',*,*,#46487,.T.);
#64966=ORIENTED_EDGE('',*,*,#47102,.T.);
#64967=ORIENTED_EDGE('',*,*,#46489,.T.);
#64968=ORIENTED_EDGE('',*,*,#46890,.T.);
#64969=ORIENTED_EDGE('',*,*,#47194,.T.);
#64970=ORIENTED_EDGE('',*,*,#47103,.T.);
#64971=ORIENTED_EDGE('',*,*,#47194,.F.);
#64972=ORIENTED_EDGE('',*,*,#46889,.T.);
#64973=ORIENTED_EDGE('',*,*,#47195,.T.);
#64974=ORIENTED_EDGE('',*,*,#47104,.T.);
#64975=ORIENTED_EDGE('',*,*,#47195,.F.);
#64976=ORIENTED_EDGE('',*,*,#46888,.T.);
#64977=ORIENTED_EDGE('',*,*,#46491,.T.);
#64978=ORIENTED_EDGE('',*,*,#47105,.T.);
#64979=ORIENTED_EDGE('',*,*,#46493,.T.);
#64980=ORIENTED_EDGE('',*,*,#46887,.T.);
#64981=ORIENTED_EDGE('',*,*,#47196,.T.);
#64982=ORIENTED_EDGE('',*,*,#47106,.T.);
#64983=ORIENTED_EDGE('',*,*,#47196,.F.);
#64984=ORIENTED_EDGE('',*,*,#46886,.T.);
#64985=ORIENTED_EDGE('',*,*,#47197,.T.);
#64986=ORIENTED_EDGE('',*,*,#47107,.T.);
#64987=ORIENTED_EDGE('',*,*,#47197,.F.);
#64988=ORIENTED_EDGE('',*,*,#46885,.T.);
#64989=ORIENTED_EDGE('',*,*,#46495,.T.);
#64990=ORIENTED_EDGE('',*,*,#47108,.T.);
#64991=ORIENTED_EDGE('',*,*,#46497,.T.);
#64992=ORIENTED_EDGE('',*,*,#46884,.T.);
#64993=ORIENTED_EDGE('',*,*,#47198,.T.);
#64994=ORIENTED_EDGE('',*,*,#47109,.T.);
#64995=ORIENTED_EDGE('',*,*,#47198,.F.);
#64996=ORIENTED_EDGE('',*,*,#46883,.T.);
#64997=ORIENTED_EDGE('',*,*,#47199,.T.);
#64998=ORIENTED_EDGE('',*,*,#47110,.T.);
#64999=ORIENTED_EDGE('',*,*,#47199,.F.);
#65000=ORIENTED_EDGE('',*,*,#46882,.T.);
#65001=ORIENTED_EDGE('',*,*,#46499,.T.);
#65002=ORIENTED_EDGE('',*,*,#47111,.T.);
#65003=ORIENTED_EDGE('',*,*,#46501,.T.);
#65004=ORIENTED_EDGE('',*,*,#46881,.T.);
#65005=ORIENTED_EDGE('',*,*,#47200,.T.);
#65006=ORIENTED_EDGE('',*,*,#47112,.T.);
#65007=ORIENTED_EDGE('',*,*,#47200,.F.);
#65008=ORIENTED_EDGE('',*,*,#46880,.T.);
#65009=ORIENTED_EDGE('',*,*,#47201,.T.);
#65010=ORIENTED_EDGE('',*,*,#47113,.T.);
#65011=ORIENTED_EDGE('',*,*,#47201,.F.);
#65012=ORIENTED_EDGE('',*,*,#46879,.T.);
#65013=ORIENTED_EDGE('',*,*,#46503,.T.);
#65014=ORIENTED_EDGE('',*,*,#47114,.T.);
#65015=ORIENTED_EDGE('',*,*,#46505,.T.);
#65016=ORIENTED_EDGE('',*,*,#46878,.T.);
#65017=ORIENTED_EDGE('',*,*,#47202,.T.);
#65018=ORIENTED_EDGE('',*,*,#47115,.T.);
#65019=ORIENTED_EDGE('',*,*,#47202,.F.);
#65020=ORIENTED_EDGE('',*,*,#46877,.T.);
#65021=ORIENTED_EDGE('',*,*,#47203,.T.);
#65022=ORIENTED_EDGE('',*,*,#47116,.T.);
#65023=ORIENTED_EDGE('',*,*,#47203,.F.);
#65024=ORIENTED_EDGE('',*,*,#46876,.T.);
#65025=ORIENTED_EDGE('',*,*,#46507,.T.);
#65026=ORIENTED_EDGE('',*,*,#47117,.T.);
#65027=ORIENTED_EDGE('',*,*,#46509,.T.);
#65028=ORIENTED_EDGE('',*,*,#46875,.T.);
#65029=ORIENTED_EDGE('',*,*,#47204,.T.);
#65030=ORIENTED_EDGE('',*,*,#47118,.T.);
#65031=ORIENTED_EDGE('',*,*,#47204,.F.);
#65032=ORIENTED_EDGE('',*,*,#46874,.T.);
#65033=ORIENTED_EDGE('',*,*,#47205,.T.);
#65034=ORIENTED_EDGE('',*,*,#47119,.T.);
#65035=ORIENTED_EDGE('',*,*,#47205,.F.);
#65036=ORIENTED_EDGE('',*,*,#46873,.T.);
#65037=ORIENTED_EDGE('',*,*,#46511,.T.);
#65038=ORIENTED_EDGE('',*,*,#47120,.T.);
#65039=ORIENTED_EDGE('',*,*,#46513,.T.);
#65040=ORIENTED_EDGE('',*,*,#46872,.T.);
#65041=ORIENTED_EDGE('',*,*,#47206,.T.);
#65042=ORIENTED_EDGE('',*,*,#47121,.T.);
#65043=ORIENTED_EDGE('',*,*,#47206,.F.);
#65044=ORIENTED_EDGE('',*,*,#46871,.T.);
#65045=ORIENTED_EDGE('',*,*,#47207,.T.);
#65046=ORIENTED_EDGE('',*,*,#47122,.T.);
#65047=ORIENTED_EDGE('',*,*,#47207,.F.);
#65048=ORIENTED_EDGE('',*,*,#46870,.T.);
#65049=ORIENTED_EDGE('',*,*,#46515,.T.);
#65050=ORIENTED_EDGE('',*,*,#47123,.T.);
#65051=ORIENTED_EDGE('',*,*,#46517,.T.);
#65052=ORIENTED_EDGE('',*,*,#46869,.T.);
#65053=ORIENTED_EDGE('',*,*,#47208,.T.);
#65054=ORIENTED_EDGE('',*,*,#47124,.T.);
#65055=ORIENTED_EDGE('',*,*,#47208,.F.);
#65056=ORIENTED_EDGE('',*,*,#46868,.T.);
#65057=ORIENTED_EDGE('',*,*,#47209,.T.);
#65058=ORIENTED_EDGE('',*,*,#47125,.T.);
#65059=ORIENTED_EDGE('',*,*,#47209,.F.);
#65060=ORIENTED_EDGE('',*,*,#46867,.T.);
#65061=ORIENTED_EDGE('',*,*,#46519,.T.);
#65062=ORIENTED_EDGE('',*,*,#47126,.T.);
#65063=ORIENTED_EDGE('',*,*,#46521,.T.);
#65064=ORIENTED_EDGE('',*,*,#46866,.T.);
#65065=ORIENTED_EDGE('',*,*,#47210,.T.);
#65066=ORIENTED_EDGE('',*,*,#47127,.T.);
#65067=ORIENTED_EDGE('',*,*,#47210,.F.);
#65068=ORIENTED_EDGE('',*,*,#46865,.T.);
#65069=ORIENTED_EDGE('',*,*,#47211,.T.);
#65070=ORIENTED_EDGE('',*,*,#47128,.T.);
#65071=ORIENTED_EDGE('',*,*,#47211,.F.);
#65072=ORIENTED_EDGE('',*,*,#46864,.T.);
#65073=ORIENTED_EDGE('',*,*,#46523,.T.);
#65074=ORIENTED_EDGE('',*,*,#47129,.T.);
#65075=ORIENTED_EDGE('',*,*,#46525,.T.);
#65076=ORIENTED_EDGE('',*,*,#46863,.T.);
#65077=ORIENTED_EDGE('',*,*,#47212,.T.);
#65078=ORIENTED_EDGE('',*,*,#47130,.T.);
#65079=ORIENTED_EDGE('',*,*,#47212,.F.);
#65080=ORIENTED_EDGE('',*,*,#46862,.T.);
#65081=ORIENTED_EDGE('',*,*,#47213,.T.);
#65082=ORIENTED_EDGE('',*,*,#47131,.T.);
#65083=ORIENTED_EDGE('',*,*,#47213,.F.);
#65084=ORIENTED_EDGE('',*,*,#46861,.T.);
#65085=ORIENTED_EDGE('',*,*,#46527,.T.);
#65086=ORIENTED_EDGE('',*,*,#47132,.T.);
#65087=ORIENTED_EDGE('',*,*,#46529,.T.);
#65088=ORIENTED_EDGE('',*,*,#46860,.T.);
#65089=ORIENTED_EDGE('',*,*,#47214,.T.);
#65090=ORIENTED_EDGE('',*,*,#47133,.T.);
#65091=ORIENTED_EDGE('',*,*,#47214,.F.);
#65092=ORIENTED_EDGE('',*,*,#46859,.T.);
#65093=ORIENTED_EDGE('',*,*,#47215,.T.);
#65094=ORIENTED_EDGE('',*,*,#47134,.T.);
#65095=ORIENTED_EDGE('',*,*,#47215,.F.);
#65096=ORIENTED_EDGE('',*,*,#46858,.T.);
#65097=ORIENTED_EDGE('',*,*,#46531,.T.);
#65098=ORIENTED_EDGE('',*,*,#47135,.T.);
#65099=ORIENTED_EDGE('',*,*,#46533,.T.);
#65100=ORIENTED_EDGE('',*,*,#46857,.T.);
#65101=ORIENTED_EDGE('',*,*,#47216,.T.);
#65102=ORIENTED_EDGE('',*,*,#47136,.T.);
#65103=ORIENTED_EDGE('',*,*,#47216,.F.);
#65104=ORIENTED_EDGE('',*,*,#46856,.T.);
#65105=ORIENTED_EDGE('',*,*,#47217,.T.);
#65106=ORIENTED_EDGE('',*,*,#47137,.T.);
#65107=ORIENTED_EDGE('',*,*,#47217,.F.);
#65108=ORIENTED_EDGE('',*,*,#46855,.T.);
#65109=ORIENTED_EDGE('',*,*,#46535,.T.);
#65110=ORIENTED_EDGE('',*,*,#47138,.T.);
#65111=ORIENTED_EDGE('',*,*,#46537,.T.);
#65112=ORIENTED_EDGE('',*,*,#46854,.T.);
#65113=ORIENTED_EDGE('',*,*,#47218,.T.);
#65114=ORIENTED_EDGE('',*,*,#47139,.T.);
#65115=ORIENTED_EDGE('',*,*,#47218,.F.);
#65116=ORIENTED_EDGE('',*,*,#46853,.T.);
#65117=ORIENTED_EDGE('',*,*,#47219,.T.);
#65118=ORIENTED_EDGE('',*,*,#47140,.T.);
#65119=ORIENTED_EDGE('',*,*,#47219,.F.);
#65120=ORIENTED_EDGE('',*,*,#46852,.T.);
#65121=ORIENTED_EDGE('',*,*,#46539,.T.);
#65122=ORIENTED_EDGE('',*,*,#47141,.T.);
#65123=ORIENTED_EDGE('',*,*,#46541,.T.);
#65124=ORIENTED_EDGE('',*,*,#46851,.T.);
#65125=ORIENTED_EDGE('',*,*,#47220,.T.);
#65126=ORIENTED_EDGE('',*,*,#47142,.T.);
#65127=ORIENTED_EDGE('',*,*,#47220,.F.);
#65128=ORIENTED_EDGE('',*,*,#46850,.T.);
#65129=ORIENTED_EDGE('',*,*,#47221,.T.);
#65130=ORIENTED_EDGE('',*,*,#47143,.T.);
#65131=ORIENTED_EDGE('',*,*,#47221,.F.);
#65132=ORIENTED_EDGE('',*,*,#46849,.T.);
#65133=ORIENTED_EDGE('',*,*,#46543,.T.);
#65134=ORIENTED_EDGE('',*,*,#47144,.T.);
#65135=ORIENTED_EDGE('',*,*,#46545,.T.);
#65136=ORIENTED_EDGE('',*,*,#46848,.T.);
#65137=ORIENTED_EDGE('',*,*,#47222,.T.);
#65138=ORIENTED_EDGE('',*,*,#47145,.T.);
#65139=ORIENTED_EDGE('',*,*,#47222,.F.);
#65140=ORIENTED_EDGE('',*,*,#46847,.T.);
#65141=ORIENTED_EDGE('',*,*,#47223,.T.);
#65142=ORIENTED_EDGE('',*,*,#47146,.T.);
#65143=ORIENTED_EDGE('',*,*,#47223,.F.);
#65144=ORIENTED_EDGE('',*,*,#46846,.T.);
#65145=ORIENTED_EDGE('',*,*,#46547,.T.);
#65146=ORIENTED_EDGE('',*,*,#47147,.T.);
#65147=ORIENTED_EDGE('',*,*,#46549,.T.);
#65148=ORIENTED_EDGE('',*,*,#46845,.T.);
#65149=ORIENTED_EDGE('',*,*,#47224,.T.);
#65150=ORIENTED_EDGE('',*,*,#47148,.T.);
#65151=ORIENTED_EDGE('',*,*,#47224,.F.);
#65152=ORIENTED_EDGE('',*,*,#46844,.T.);
#65153=ORIENTED_EDGE('',*,*,#47225,.T.);
#65154=ORIENTED_EDGE('',*,*,#47149,.T.);
#65155=ORIENTED_EDGE('',*,*,#47225,.F.);
#65156=ORIENTED_EDGE('',*,*,#46843,.T.);
#65157=ORIENTED_EDGE('',*,*,#46551,.T.);
#65158=ORIENTED_EDGE('',*,*,#47150,.T.);
#65159=ORIENTED_EDGE('',*,*,#46553,.T.);
#65160=ORIENTED_EDGE('',*,*,#46842,.T.);
#65161=ORIENTED_EDGE('',*,*,#47226,.T.);
#65162=ORIENTED_EDGE('',*,*,#47151,.T.);
#65163=ORIENTED_EDGE('',*,*,#47226,.F.);
#65164=ORIENTED_EDGE('',*,*,#46841,.T.);
#65165=ORIENTED_EDGE('',*,*,#47227,.T.);
#65166=ORIENTED_EDGE('',*,*,#47152,.T.);
#65167=ORIENTED_EDGE('',*,*,#47227,.F.);
#65168=ORIENTED_EDGE('',*,*,#46840,.T.);
#65169=ORIENTED_EDGE('',*,*,#46555,.T.);
#65170=ORIENTED_EDGE('',*,*,#47153,.T.);
#65171=ORIENTED_EDGE('',*,*,#46557,.T.);
#65172=ORIENTED_EDGE('',*,*,#46839,.T.);
#65173=ORIENTED_EDGE('',*,*,#47228,.T.);
#65174=ORIENTED_EDGE('',*,*,#46944,.T.);
#65175=ORIENTED_EDGE('',*,*,#47154,.T.);
#65176=ORIENTED_EDGE('',*,*,#47228,.F.);
#65177=ORIENTED_EDGE('',*,*,#46838,.T.);
#65178=ORIENTED_EDGE('',*,*,#46835,.T.);
#65179=ORIENTED_EDGE('',*,*,#47229,.T.);
#65180=ORIENTED_EDGE('',*,*,#46945,.T.);
#65181=ORIENTED_EDGE('',*,*,#47229,.F.);
#65182=ORIENTED_EDGE('',*,*,#46834,.T.);
#65183=ORIENTED_EDGE('',*,*,#46559,.T.);
#65184=ORIENTED_EDGE('',*,*,#46946,.T.);
#65185=ORIENTED_EDGE('',*,*,#46561,.T.);
#65186=ORIENTED_EDGE('',*,*,#46833,.T.);
#65187=ORIENTED_EDGE('',*,*,#47230,.T.);
#65188=ORIENTED_EDGE('',*,*,#46947,.T.);
#65189=ORIENTED_EDGE('',*,*,#47230,.F.);
#65190=ORIENTED_EDGE('',*,*,#46832,.T.);
#65191=ORIENTED_EDGE('',*,*,#47231,.T.);
#65192=ORIENTED_EDGE('',*,*,#46948,.T.);
#65193=ORIENTED_EDGE('',*,*,#47231,.F.);
#65194=ORIENTED_EDGE('',*,*,#46831,.T.);
#65195=ORIENTED_EDGE('',*,*,#46563,.T.);
#65196=ORIENTED_EDGE('',*,*,#46949,.T.);
#65197=ORIENTED_EDGE('',*,*,#46565,.T.);
#65198=ORIENTED_EDGE('',*,*,#46830,.T.);
#65199=ORIENTED_EDGE('',*,*,#47232,.T.);
#65200=ORIENTED_EDGE('',*,*,#46950,.T.);
#65201=ORIENTED_EDGE('',*,*,#47232,.F.);
#65202=ORIENTED_EDGE('',*,*,#46829,.T.);
#65203=ORIENTED_EDGE('',*,*,#47233,.T.);
#65204=ORIENTED_EDGE('',*,*,#46951,.T.);
#65205=ORIENTED_EDGE('',*,*,#47233,.F.);
#65206=ORIENTED_EDGE('',*,*,#46828,.T.);
#65207=ORIENTED_EDGE('',*,*,#46567,.T.);
#65208=ORIENTED_EDGE('',*,*,#46952,.T.);
#65209=ORIENTED_EDGE('',*,*,#46569,.T.);
#65210=ORIENTED_EDGE('',*,*,#46827,.T.);
#65211=ORIENTED_EDGE('',*,*,#47234,.T.);
#65212=ORIENTED_EDGE('',*,*,#46953,.T.);
#65213=ORIENTED_EDGE('',*,*,#47234,.F.);
#65214=ORIENTED_EDGE('',*,*,#46826,.T.);
#65215=ORIENTED_EDGE('',*,*,#47235,.T.);
#65216=ORIENTED_EDGE('',*,*,#46954,.T.);
#65217=ORIENTED_EDGE('',*,*,#47235,.F.);
#65218=ORIENTED_EDGE('',*,*,#46825,.T.);
#65219=ORIENTED_EDGE('',*,*,#46571,.T.);
#65220=ORIENTED_EDGE('',*,*,#46955,.T.);
#65221=ORIENTED_EDGE('',*,*,#46573,.T.);
#65222=ORIENTED_EDGE('',*,*,#46824,.T.);
#65223=ORIENTED_EDGE('',*,*,#47236,.T.);
#65224=ORIENTED_EDGE('',*,*,#46956,.T.);
#65225=ORIENTED_EDGE('',*,*,#47236,.F.);
#65226=ORIENTED_EDGE('',*,*,#46823,.T.);
#65227=ORIENTED_EDGE('',*,*,#47237,.T.);
#65228=ORIENTED_EDGE('',*,*,#46957,.T.);
#65229=ORIENTED_EDGE('',*,*,#47237,.F.);
#65230=ORIENTED_EDGE('',*,*,#46822,.T.);
#65231=ORIENTED_EDGE('',*,*,#46575,.T.);
#65232=ORIENTED_EDGE('',*,*,#46958,.T.);
#65233=ORIENTED_EDGE('',*,*,#46577,.T.);
#65234=ORIENTED_EDGE('',*,*,#46821,.T.);
#65235=ORIENTED_EDGE('',*,*,#47238,.T.);
#65236=ORIENTED_EDGE('',*,*,#46959,.T.);
#65237=ORIENTED_EDGE('',*,*,#47238,.F.);
#65238=ORIENTED_EDGE('',*,*,#46820,.T.);
#65239=ORIENTED_EDGE('',*,*,#47239,.T.);
#65240=ORIENTED_EDGE('',*,*,#46960,.T.);
#65241=ORIENTED_EDGE('',*,*,#47239,.F.);
#65242=ORIENTED_EDGE('',*,*,#46819,.T.);
#65243=ORIENTED_EDGE('',*,*,#46579,.T.);
#65244=ORIENTED_EDGE('',*,*,#46961,.T.);
#65245=ORIENTED_EDGE('',*,*,#46581,.T.);
#65246=ORIENTED_EDGE('',*,*,#46818,.T.);
#65247=ORIENTED_EDGE('',*,*,#47240,.T.);
#65248=ORIENTED_EDGE('',*,*,#46962,.T.);
#65249=ORIENTED_EDGE('',*,*,#47240,.F.);
#65250=ORIENTED_EDGE('',*,*,#46817,.T.);
#65251=ORIENTED_EDGE('',*,*,#47241,.T.);
#65252=ORIENTED_EDGE('',*,*,#46963,.T.);
#65253=ORIENTED_EDGE('',*,*,#47241,.F.);
#65254=ORIENTED_EDGE('',*,*,#46816,.T.);
#65255=ORIENTED_EDGE('',*,*,#46583,.T.);
#65256=ORIENTED_EDGE('',*,*,#46964,.T.);
#65257=ORIENTED_EDGE('',*,*,#46585,.T.);
#65258=ORIENTED_EDGE('',*,*,#46815,.T.);
#65259=ORIENTED_EDGE('',*,*,#47242,.T.);
#65260=ORIENTED_EDGE('',*,*,#46965,.T.);
#65261=ORIENTED_EDGE('',*,*,#47242,.F.);
#65262=ORIENTED_EDGE('',*,*,#46814,.T.);
#65263=ORIENTED_EDGE('',*,*,#47243,.T.);
#65264=ORIENTED_EDGE('',*,*,#46966,.T.);
#65265=ORIENTED_EDGE('',*,*,#47243,.F.);
#65266=ORIENTED_EDGE('',*,*,#46813,.T.);
#65267=ORIENTED_EDGE('',*,*,#46587,.T.);
#65268=ORIENTED_EDGE('',*,*,#46967,.T.);
#65269=ORIENTED_EDGE('',*,*,#46589,.T.);
#65270=ORIENTED_EDGE('',*,*,#46812,.T.);
#65271=ORIENTED_EDGE('',*,*,#47244,.T.);
#65272=ORIENTED_EDGE('',*,*,#46968,.T.);
#65273=ORIENTED_EDGE('',*,*,#47244,.F.);
#65274=ORIENTED_EDGE('',*,*,#46811,.T.);
#65275=ORIENTED_EDGE('',*,*,#47245,.T.);
#65276=ORIENTED_EDGE('',*,*,#46969,.T.);
#65277=ORIENTED_EDGE('',*,*,#47245,.F.);
#65278=ORIENTED_EDGE('',*,*,#46810,.T.);
#65279=ORIENTED_EDGE('',*,*,#46591,.T.);
#65280=ORIENTED_EDGE('',*,*,#46970,.T.);
#65281=ORIENTED_EDGE('',*,*,#46593,.T.);
#65282=ORIENTED_EDGE('',*,*,#46809,.T.);
#65283=ORIENTED_EDGE('',*,*,#47246,.T.);
#65284=ORIENTED_EDGE('',*,*,#46971,.T.);
#65285=ORIENTED_EDGE('',*,*,#47246,.F.);
#65286=ORIENTED_EDGE('',*,*,#46808,.T.);
#65287=ORIENTED_EDGE('',*,*,#47247,.T.);
#65288=ORIENTED_EDGE('',*,*,#46972,.T.);
#65289=ORIENTED_EDGE('',*,*,#47247,.F.);
#65290=ORIENTED_EDGE('',*,*,#46807,.T.);
#65291=ORIENTED_EDGE('',*,*,#46595,.T.);
#65292=ORIENTED_EDGE('',*,*,#46973,.T.);
#65293=ORIENTED_EDGE('',*,*,#46597,.T.);
#65294=ORIENTED_EDGE('',*,*,#46806,.T.);
#65295=ORIENTED_EDGE('',*,*,#47248,.T.);
#65296=ORIENTED_EDGE('',*,*,#46974,.T.);
#65297=ORIENTED_EDGE('',*,*,#47248,.F.);
#65298=ORIENTED_EDGE('',*,*,#46805,.T.);
#65299=ORIENTED_EDGE('',*,*,#47249,.T.);
#65300=ORIENTED_EDGE('',*,*,#46975,.T.);
#65301=ORIENTED_EDGE('',*,*,#47249,.F.);
#65302=ORIENTED_EDGE('',*,*,#46804,.T.);
#65303=ORIENTED_EDGE('',*,*,#46599,.T.);
#65304=ORIENTED_EDGE('',*,*,#46976,.T.);
#65305=ORIENTED_EDGE('',*,*,#46601,.T.);
#65306=ORIENTED_EDGE('',*,*,#46803,.T.);
#65307=ORIENTED_EDGE('',*,*,#47250,.T.);
#65308=ORIENTED_EDGE('',*,*,#46977,.T.);
#65309=ORIENTED_EDGE('',*,*,#47250,.F.);
#65310=ORIENTED_EDGE('',*,*,#46802,.T.);
#65311=ORIENTED_EDGE('',*,*,#47251,.T.);
#65312=ORIENTED_EDGE('',*,*,#46978,.T.);
#65313=ORIENTED_EDGE('',*,*,#47251,.F.);
#65314=ORIENTED_EDGE('',*,*,#46801,.T.);
#65315=ORIENTED_EDGE('',*,*,#46603,.T.);
#65316=ORIENTED_EDGE('',*,*,#46979,.T.);
#65317=ORIENTED_EDGE('',*,*,#46605,.T.);
#65318=ORIENTED_EDGE('',*,*,#46800,.T.);
#65319=ORIENTED_EDGE('',*,*,#47252,.T.);
#65320=ORIENTED_EDGE('',*,*,#46980,.T.);
#65321=ORIENTED_EDGE('',*,*,#47252,.F.);
#65322=ORIENTED_EDGE('',*,*,#46799,.T.);
#65323=ORIENTED_EDGE('',*,*,#47253,.T.);
#65324=ORIENTED_EDGE('',*,*,#46981,.T.);
#65325=ORIENTED_EDGE('',*,*,#47253,.F.);
#65326=ORIENTED_EDGE('',*,*,#46798,.T.);
#65327=ORIENTED_EDGE('',*,*,#46607,.T.);
#65328=ORIENTED_EDGE('',*,*,#46982,.T.);
#65329=ORIENTED_EDGE('',*,*,#46609,.T.);
#65330=ORIENTED_EDGE('',*,*,#46797,.T.);
#65331=ORIENTED_EDGE('',*,*,#47254,.T.);
#65332=ORIENTED_EDGE('',*,*,#46983,.T.);
#65333=ORIENTED_EDGE('',*,*,#47254,.F.);
#65334=ORIENTED_EDGE('',*,*,#46796,.T.);
#65335=ORIENTED_EDGE('',*,*,#47255,.T.);
#65336=ORIENTED_EDGE('',*,*,#46984,.T.);
#65337=ORIENTED_EDGE('',*,*,#47255,.F.);
#65338=ORIENTED_EDGE('',*,*,#46795,.T.);
#65339=ORIENTED_EDGE('',*,*,#46611,.T.);
#65340=ORIENTED_EDGE('',*,*,#46985,.T.);
#65341=ORIENTED_EDGE('',*,*,#46613,.T.);
#65342=ORIENTED_EDGE('',*,*,#46794,.T.);
#65343=ORIENTED_EDGE('',*,*,#47256,.T.);
#65344=ORIENTED_EDGE('',*,*,#46986,.T.);
#65345=ORIENTED_EDGE('',*,*,#47256,.F.);
#65346=ORIENTED_EDGE('',*,*,#46793,.T.);
#65347=ORIENTED_EDGE('',*,*,#47257,.T.);
#65348=ORIENTED_EDGE('',*,*,#46987,.T.);
#65349=ORIENTED_EDGE('',*,*,#47257,.F.);
#65350=ORIENTED_EDGE('',*,*,#46792,.T.);
#65351=ORIENTED_EDGE('',*,*,#46615,.T.);
#65352=ORIENTED_EDGE('',*,*,#46988,.T.);
#65353=ORIENTED_EDGE('',*,*,#46617,.T.);
#65354=ORIENTED_EDGE('',*,*,#46791,.T.);
#65355=ORIENTED_EDGE('',*,*,#47258,.T.);
#65356=ORIENTED_EDGE('',*,*,#46989,.T.);
#65357=ORIENTED_EDGE('',*,*,#47258,.F.);
#65358=ORIENTED_EDGE('',*,*,#46790,.T.);
#65359=ORIENTED_EDGE('',*,*,#47259,.T.);
#65360=ORIENTED_EDGE('',*,*,#46990,.T.);
#65361=ORIENTED_EDGE('',*,*,#47259,.F.);
#65362=ORIENTED_EDGE('',*,*,#46789,.T.);
#65363=ORIENTED_EDGE('',*,*,#46619,.T.);
#65364=ORIENTED_EDGE('',*,*,#46991,.T.);
#65365=ORIENTED_EDGE('',*,*,#46621,.T.);
#65366=ORIENTED_EDGE('',*,*,#46788,.T.);
#65367=ORIENTED_EDGE('',*,*,#47260,.T.);
#65368=ORIENTED_EDGE('',*,*,#46992,.T.);
#65369=ORIENTED_EDGE('',*,*,#47260,.F.);
#65370=ORIENTED_EDGE('',*,*,#46787,.T.);
#65371=ORIENTED_EDGE('',*,*,#47261,.T.);
#65372=ORIENTED_EDGE('',*,*,#46993,.T.);
#65373=ORIENTED_EDGE('',*,*,#47261,.F.);
#65374=ORIENTED_EDGE('',*,*,#46786,.T.);
#65375=ORIENTED_EDGE('',*,*,#46623,.T.);
#65376=ORIENTED_EDGE('',*,*,#46994,.T.);
#65377=ORIENTED_EDGE('',*,*,#46625,.T.);
#65378=ORIENTED_EDGE('',*,*,#46785,.T.);
#65379=ORIENTED_EDGE('',*,*,#47262,.T.);
#65380=ORIENTED_EDGE('',*,*,#46995,.T.);
#65381=ORIENTED_EDGE('',*,*,#47262,.F.);
#65382=ORIENTED_EDGE('',*,*,#46784,.T.);
#65383=ORIENTED_EDGE('',*,*,#47263,.T.);
#65384=ORIENTED_EDGE('',*,*,#46996,.T.);
#65385=ORIENTED_EDGE('',*,*,#47263,.F.);
#65386=ORIENTED_EDGE('',*,*,#46783,.T.);
#65387=ORIENTED_EDGE('',*,*,#46627,.T.);
#65388=ORIENTED_EDGE('',*,*,#46997,.T.);
#65389=ORIENTED_EDGE('',*,*,#46629,.T.);
#65390=ORIENTED_EDGE('',*,*,#46782,.T.);
#65391=ORIENTED_EDGE('',*,*,#47264,.T.);
#65392=ORIENTED_EDGE('',*,*,#46998,.T.);
#65393=ORIENTED_EDGE('',*,*,#47264,.F.);
#65394=ORIENTED_EDGE('',*,*,#46781,.T.);
#65395=ORIENTED_EDGE('',*,*,#47265,.T.);
#65396=ORIENTED_EDGE('',*,*,#46999,.T.);
#65397=ORIENTED_EDGE('',*,*,#47265,.F.);
#65398=ORIENTED_EDGE('',*,*,#46780,.T.);
#65399=ORIENTED_EDGE('',*,*,#46631,.T.);
#65400=ORIENTED_EDGE('',*,*,#47000,.T.);
#65401=ORIENTED_EDGE('',*,*,#46633,.T.);
#65402=ORIENTED_EDGE('',*,*,#46779,.T.);
#65403=ORIENTED_EDGE('',*,*,#47266,.T.);
#65404=ORIENTED_EDGE('',*,*,#47001,.T.);
#65405=ORIENTED_EDGE('',*,*,#47266,.F.);
#65406=ORIENTED_EDGE('',*,*,#46778,.T.);
#65407=ORIENTED_EDGE('',*,*,#47267,.T.);
#65408=ORIENTED_EDGE('',*,*,#47002,.T.);
#65409=ORIENTED_EDGE('',*,*,#47267,.F.);
#65410=ORIENTED_EDGE('',*,*,#46777,.T.);
#65411=ORIENTED_EDGE('',*,*,#46635,.T.);
#65412=ORIENTED_EDGE('',*,*,#47003,.T.);
#65413=ORIENTED_EDGE('',*,*,#46637,.T.);
#65414=ORIENTED_EDGE('',*,*,#46776,.T.);
#65415=ORIENTED_EDGE('',*,*,#47268,.T.);
#65416=ORIENTED_EDGE('',*,*,#47004,.T.);
#65417=ORIENTED_EDGE('',*,*,#47268,.F.);
#65418=ORIENTED_EDGE('',*,*,#46775,.T.);
#65419=ORIENTED_EDGE('',*,*,#47269,.T.);
#65420=ORIENTED_EDGE('',*,*,#47005,.T.);
#65421=ORIENTED_EDGE('',*,*,#47269,.F.);
#65422=ORIENTED_EDGE('',*,*,#46774,.T.);
#65423=ORIENTED_EDGE('',*,*,#46639,.T.);
#65424=ORIENTED_EDGE('',*,*,#47006,.T.);
#65425=ORIENTED_EDGE('',*,*,#46641,.T.);
#65426=ORIENTED_EDGE('',*,*,#46773,.T.);
#65427=ORIENTED_EDGE('',*,*,#47270,.T.);
#65428=ORIENTED_EDGE('',*,*,#47007,.T.);
#65429=ORIENTED_EDGE('',*,*,#47270,.F.);
#65430=ORIENTED_EDGE('',*,*,#46772,.T.);
#65431=ORIENTED_EDGE('',*,*,#47271,.T.);
#65432=ORIENTED_EDGE('',*,*,#47008,.T.);
#65433=ORIENTED_EDGE('',*,*,#47271,.F.);
#65434=ORIENTED_EDGE('',*,*,#46771,.T.);
#65435=ORIENTED_EDGE('',*,*,#46643,.T.);
#65436=ORIENTED_EDGE('',*,*,#47009,.T.);
#65437=ORIENTED_EDGE('',*,*,#46645,.T.);
#65438=ORIENTED_EDGE('',*,*,#46770,.T.);
#65439=ORIENTED_EDGE('',*,*,#47272,.T.);
#65440=ORIENTED_EDGE('',*,*,#47010,.T.);
#65441=ORIENTED_EDGE('',*,*,#47272,.F.);
#65442=ORIENTED_EDGE('',*,*,#46769,.T.);
#65443=ORIENTED_EDGE('',*,*,#47273,.T.);
#65444=ORIENTED_EDGE('',*,*,#47011,.T.);
#65445=ORIENTED_EDGE('',*,*,#47273,.F.);
#65446=ORIENTED_EDGE('',*,*,#46768,.T.);
#65447=ORIENTED_EDGE('',*,*,#46647,.T.);
#65448=ORIENTED_EDGE('',*,*,#47012,.T.);
#65449=ORIENTED_EDGE('',*,*,#46649,.T.);
#65450=ORIENTED_EDGE('',*,*,#46767,.T.);
#65451=ORIENTED_EDGE('',*,*,#47274,.T.);
#65452=ORIENTED_EDGE('',*,*,#47013,.T.);
#65453=ORIENTED_EDGE('',*,*,#47274,.F.);
#65454=ORIENTED_EDGE('',*,*,#46766,.T.);
#65455=ORIENTED_EDGE('',*,*,#47275,.T.);
#65456=ORIENTED_EDGE('',*,*,#47014,.T.);
#65457=ORIENTED_EDGE('',*,*,#47275,.F.);
#65458=ORIENTED_EDGE('',*,*,#46765,.T.);
#65459=ORIENTED_EDGE('',*,*,#46651,.T.);
#65460=ORIENTED_EDGE('',*,*,#47015,.T.);
#65461=ORIENTED_EDGE('',*,*,#46653,.T.);
#65462=ORIENTED_EDGE('',*,*,#46764,.T.);
#65463=ORIENTED_EDGE('',*,*,#47276,.T.);
#65464=ORIENTED_EDGE('',*,*,#47016,.T.);
#65465=ORIENTED_EDGE('',*,*,#47276,.F.);
#65466=ORIENTED_EDGE('',*,*,#46763,.T.);
#65467=ORIENTED_EDGE('',*,*,#47277,.T.);
#65468=ORIENTED_EDGE('',*,*,#47017,.T.);
#65469=ORIENTED_EDGE('',*,*,#47277,.F.);
#65470=ORIENTED_EDGE('',*,*,#46762,.T.);
#65471=ORIENTED_EDGE('',*,*,#46655,.T.);
#65472=ORIENTED_EDGE('',*,*,#47018,.T.);
#65473=ORIENTED_EDGE('',*,*,#46657,.T.);
#65474=ORIENTED_EDGE('',*,*,#46761,.T.);
#65475=ORIENTED_EDGE('',*,*,#47278,.T.);
#65476=ORIENTED_EDGE('',*,*,#47019,.T.);
#65477=ORIENTED_EDGE('',*,*,#47278,.F.);
#65478=ORIENTED_EDGE('',*,*,#46760,.T.);
#65479=ORIENTED_EDGE('',*,*,#47279,.T.);
#65480=ORIENTED_EDGE('',*,*,#47020,.T.);
#65481=ORIENTED_EDGE('',*,*,#47279,.F.);
#65482=ORIENTED_EDGE('',*,*,#46759,.T.);
#65483=ORIENTED_EDGE('',*,*,#46659,.T.);
#65484=ORIENTED_EDGE('',*,*,#47021,.T.);
#65485=ORIENTED_EDGE('',*,*,#46661,.T.);
#65486=ORIENTED_EDGE('',*,*,#46758,.T.);
#65487=ORIENTED_EDGE('',*,*,#47280,.T.);
#65488=ORIENTED_EDGE('',*,*,#47022,.T.);
#65489=ORIENTED_EDGE('',*,*,#47280,.F.);
#65490=ORIENTED_EDGE('',*,*,#46757,.T.);
#65491=ORIENTED_EDGE('',*,*,#47281,.T.);
#65492=ORIENTED_EDGE('',*,*,#47023,.T.);
#65493=ORIENTED_EDGE('',*,*,#47281,.F.);
#65494=ORIENTED_EDGE('',*,*,#46756,.T.);
#65495=ORIENTED_EDGE('',*,*,#46663,.T.);
#65496=ORIENTED_EDGE('',*,*,#47024,.T.);
#65497=ORIENTED_EDGE('',*,*,#46665,.T.);
#65498=ORIENTED_EDGE('',*,*,#46755,.T.);
#65499=ORIENTED_EDGE('',*,*,#47282,.T.);
#65500=ORIENTED_EDGE('',*,*,#47025,.T.);
#65501=ORIENTED_EDGE('',*,*,#47282,.F.);
#65502=ORIENTED_EDGE('',*,*,#46754,.T.);
#65503=ORIENTED_EDGE('',*,*,#47283,.T.);
#65504=ORIENTED_EDGE('',*,*,#47026,.T.);
#65505=ORIENTED_EDGE('',*,*,#47283,.F.);
#65506=ORIENTED_EDGE('',*,*,#46753,.T.);
#65507=ORIENTED_EDGE('',*,*,#46667,.T.);
#65508=ORIENTED_EDGE('',*,*,#47027,.T.);
#65509=ORIENTED_EDGE('',*,*,#46669,.T.);
#65510=ORIENTED_EDGE('',*,*,#46752,.T.);
#65511=ORIENTED_EDGE('',*,*,#47284,.T.);
#65512=ORIENTED_EDGE('',*,*,#47028,.T.);
#65513=ORIENTED_EDGE('',*,*,#47284,.F.);
#65514=ORIENTED_EDGE('',*,*,#46751,.T.);
#65515=ORIENTED_EDGE('',*,*,#47285,.T.);
#65516=ORIENTED_EDGE('',*,*,#47029,.T.);
#65517=ORIENTED_EDGE('',*,*,#47285,.F.);
#65518=ORIENTED_EDGE('',*,*,#46750,.T.);
#65519=ORIENTED_EDGE('',*,*,#46671,.T.);
#65520=ORIENTED_EDGE('',*,*,#47030,.T.);
#65521=ORIENTED_EDGE('',*,*,#46673,.T.);
#65522=ORIENTED_EDGE('',*,*,#46749,.T.);
#65523=ORIENTED_EDGE('',*,*,#47286,.T.);
#65524=ORIENTED_EDGE('',*,*,#47031,.T.);
#65525=ORIENTED_EDGE('',*,*,#47286,.F.);
#65526=ORIENTED_EDGE('',*,*,#46748,.T.);
#65527=ORIENTED_EDGE('',*,*,#47287,.T.);
#65528=ORIENTED_EDGE('',*,*,#47032,.T.);
#65529=ORIENTED_EDGE('',*,*,#47287,.F.);
#65530=ORIENTED_EDGE('',*,*,#46747,.T.);
#65531=ORIENTED_EDGE('',*,*,#46675,.T.);
#65532=ORIENTED_EDGE('',*,*,#47033,.T.);
#65533=ORIENTED_EDGE('',*,*,#46677,.T.);
#65534=ORIENTED_EDGE('',*,*,#46746,.T.);
#65535=ORIENTED_EDGE('',*,*,#47288,.T.);
#65536=ORIENTED_EDGE('',*,*,#47034,.T.);
#65537=ORIENTED_EDGE('',*,*,#47288,.F.);
#65538=ORIENTED_EDGE('',*,*,#46745,.T.);
#65539=ORIENTED_EDGE('',*,*,#47289,.T.);
#65540=ORIENTED_EDGE('',*,*,#47035,.T.);
#65541=ORIENTED_EDGE('',*,*,#47289,.F.);
#65542=ORIENTED_EDGE('',*,*,#46744,.T.);
#65543=ORIENTED_EDGE('',*,*,#46679,.T.);
#65544=ORIENTED_EDGE('',*,*,#47036,.T.);
#65545=ORIENTED_EDGE('',*,*,#46681,.T.);
#65546=ORIENTED_EDGE('',*,*,#46743,.T.);
#65547=ORIENTED_EDGE('',*,*,#47290,.T.);
#65548=ORIENTED_EDGE('',*,*,#47037,.T.);
#65549=ORIENTED_EDGE('',*,*,#47290,.F.);
#65550=ORIENTED_EDGE('',*,*,#46742,.T.);
#65551=ORIENTED_EDGE('',*,*,#47291,.T.);
#65552=ORIENTED_EDGE('',*,*,#47038,.T.);
#65553=ORIENTED_EDGE('',*,*,#47291,.F.);
#65554=ORIENTED_EDGE('',*,*,#46741,.T.);
#65555=ORIENTED_EDGE('',*,*,#46683,.T.);
#65556=ORIENTED_EDGE('',*,*,#47039,.T.);
#65557=ORIENTED_EDGE('',*,*,#46685,.T.);
#65558=ORIENTED_EDGE('',*,*,#46740,.T.);
#65559=ORIENTED_EDGE('',*,*,#47292,.T.);
#65560=ORIENTED_EDGE('',*,*,#47040,.T.);
#65561=ORIENTED_EDGE('',*,*,#47292,.F.);
#65562=ORIENTED_EDGE('',*,*,#46739,.T.);
#65563=ORIENTED_EDGE('',*,*,#47293,.T.);
#65564=ORIENTED_EDGE('',*,*,#47041,.T.);
#65565=ORIENTED_EDGE('',*,*,#47293,.F.);
#65566=ORIENTED_EDGE('',*,*,#46738,.T.);
#65567=ORIENTED_EDGE('',*,*,#46687,.T.);
#65568=ORIENTED_EDGE('',*,*,#47042,.T.);
#65569=ORIENTED_EDGE('',*,*,#46689,.T.);
#65570=ORIENTED_EDGE('',*,*,#46737,.T.);
#65571=ORIENTED_EDGE('',*,*,#47294,.T.);
#65572=ORIENTED_EDGE('',*,*,#47043,.T.);
#65573=ORIENTED_EDGE('',*,*,#47294,.F.);
#65574=ORIENTED_EDGE('',*,*,#46736,.T.);
#65575=ORIENTED_EDGE('',*,*,#47295,.T.);
#65576=ORIENTED_EDGE('',*,*,#47044,.T.);
#65577=ORIENTED_EDGE('',*,*,#47295,.F.);
#65578=ORIENTED_EDGE('',*,*,#46735,.T.);
#65579=ORIENTED_EDGE('',*,*,#46691,.T.);
#65580=ORIENTED_EDGE('',*,*,#47045,.T.);
#65581=ORIENTED_EDGE('',*,*,#46693,.T.);
#65582=ORIENTED_EDGE('',*,*,#46734,.T.);
#65583=ORIENTED_EDGE('',*,*,#47296,.T.);
#65584=ORIENTED_EDGE('',*,*,#47046,.T.);
#65585=ORIENTED_EDGE('',*,*,#47296,.F.);
#65586=ORIENTED_EDGE('',*,*,#46733,.T.);
#65587=ORIENTED_EDGE('',*,*,#47297,.T.);
#65588=ORIENTED_EDGE('',*,*,#47047,.T.);
#65589=ORIENTED_EDGE('',*,*,#47297,.F.);
#65590=ORIENTED_EDGE('',*,*,#46732,.T.);
#65591=ORIENTED_EDGE('',*,*,#46695,.T.);
#65592=ORIENTED_EDGE('',*,*,#47298,.F.);
#65593=ORIENTED_EDGE('',*,*,#47299,.T.);
#65594=ORIENTED_EDGE('',*,*,#47300,.T.);
#65595=ORIENTED_EDGE('',*,*,#47299,.F.);
#65596=ORIENTED_EDGE('',*,*,#47301,.F.);
#65597=ORIENTED_EDGE('',*,*,#47302,.T.);
#65598=ORIENTED_EDGE('',*,*,#47303,.T.);
#65599=ORIENTED_EDGE('',*,*,#47302,.F.);
#65600=ORIENTED_EDGE('',*,*,#47304,.F.);
#65601=ORIENTED_EDGE('',*,*,#47305,.T.);
#65602=ORIENTED_EDGE('',*,*,#47306,.F.);
#65603=ORIENTED_EDGE('',*,*,#47305,.F.);
#65604=ORIENTED_EDGE('',*,*,#47307,.F.);
#65605=ORIENTED_EDGE('',*,*,#47308,.T.);
#65606=ORIENTED_EDGE('',*,*,#47309,.F.);
#65607=ORIENTED_EDGE('',*,*,#47308,.F.);
#65608=ORIENTED_EDGE('',*,*,#47310,.F.);
#65609=ORIENTED_EDGE('',*,*,#47311,.T.);
#65610=ORIENTED_EDGE('',*,*,#47312,.F.);
#65611=ORIENTED_EDGE('',*,*,#47311,.F.);
#65612=ORIENTED_EDGE('',*,*,#47313,.F.);
#65613=ORIENTED_EDGE('',*,*,#47314,.F.);
#65614=ORIENTED_EDGE('',*,*,#47315,.T.);
#65615=ORIENTED_EDGE('',*,*,#47316,.F.);
#65616=ORIENTED_EDGE('',*,*,#47315,.F.);
#65617=ORIENTED_EDGE('',*,*,#47317,.F.);
#65618=ORIENTED_EDGE('',*,*,#47318,.T.);
#65619=ORIENTED_EDGE('',*,*,#47319,.F.);
#65620=ORIENTED_EDGE('',*,*,#47320,.F.);
#65621=ORIENTED_EDGE('',*,*,#47318,.F.);
#65622=ORIENTED_EDGE('',*,*,#47321,.F.);
#65623=ORIENTED_EDGE('',*,*,#47322,.T.);
#65624=ORIENTED_EDGE('',*,*,#47323,.F.);
#65625=ORIENTED_EDGE('',*,*,#47324,.F.);
#65626=ORIENTED_EDGE('',*,*,#47325,.F.);
#65627=ORIENTED_EDGE('',*,*,#47326,.T.);
#65628=ORIENTED_EDGE('',*,*,#47327,.F.);
#65629=ORIENTED_EDGE('',*,*,#47328,.F.);
#65630=ORIENTED_EDGE('',*,*,#47329,.F.);
#65631=ORIENTED_EDGE('',*,*,#47330,.T.);
#65632=ORIENTED_EDGE('',*,*,#47331,.F.);
#65633=ORIENTED_EDGE('',*,*,#47332,.F.);
#65634=ORIENTED_EDGE('',*,*,#47330,.F.);
#65635=ORIENTED_EDGE('',*,*,#47333,.F.);
#65636=ORIENTED_EDGE('',*,*,#47334,.T.);
#65637=ORIENTED_EDGE('',*,*,#47335,.F.);
#65638=ORIENTED_EDGE('',*,*,#47336,.F.);
#65639=ORIENTED_EDGE('',*,*,#47334,.F.);
#65640=ORIENTED_EDGE('',*,*,#47337,.F.);
#65641=ORIENTED_EDGE('',*,*,#47338,.T.);
#65642=ORIENTED_EDGE('',*,*,#47339,.F.);
#65643=ORIENTED_EDGE('',*,*,#47340,.F.);
#65644=ORIENTED_EDGE('',*,*,#47338,.F.);
#65645=ORIENTED_EDGE('',*,*,#47341,.T.);
#65646=ORIENTED_EDGE('',*,*,#47342,.F.);
#65647=ORIENTED_EDGE('',*,*,#47343,.T.);
#65648=ORIENTED_EDGE('',*,*,#47344,.T.);
#65649=ORIENTED_EDGE('',*,*,#47345,.T.);
#65650=ORIENTED_EDGE('',*,*,#47346,.F.);
#65651=ORIENTED_EDGE('',*,*,#47347,.T.);
#65652=ORIENTED_EDGE('',*,*,#47348,.T.);
#65653=ORIENTED_EDGE('',*,*,#47349,.F.);
#65654=ORIENTED_EDGE('',*,*,#47350,.T.);
#65655=ORIENTED_EDGE('',*,*,#47331,.T.);
#65656=ORIENTED_EDGE('',*,*,#47332,.T.);
#65657=ORIENTED_EDGE('',*,*,#47350,.F.);
#65658=ORIENTED_EDGE('',*,*,#47306,.T.);
#65659=ORIENTED_EDGE('',*,*,#47351,.T.);
#65660=ORIENTED_EDGE('',*,*,#47335,.T.);
#65661=ORIENTED_EDGE('',*,*,#47336,.T.);
#65662=ORIENTED_EDGE('',*,*,#47351,.F.);
#65663=ORIENTED_EDGE('',*,*,#47309,.T.);
#65664=ORIENTED_EDGE('',*,*,#47352,.T.);
#65665=ORIENTED_EDGE('',*,*,#47339,.T.);
#65666=ORIENTED_EDGE('',*,*,#47340,.T.);
#65667=ORIENTED_EDGE('',*,*,#47352,.F.);
#65668=ORIENTED_EDGE('',*,*,#47353,.T.);
#65669=ORIENTED_EDGE('',*,*,#47354,.T.);
#65670=ORIENTED_EDGE('',*,*,#47319,.T.);
#65671=ORIENTED_EDGE('',*,*,#47320,.T.);
#65672=ORIENTED_EDGE('',*,*,#47354,.F.);
#65673=ORIENTED_EDGE('',*,*,#47355,.T.);
#65674=ORIENTED_EDGE('',*,*,#47356,.T.);
#65675=ORIENTED_EDGE('',*,*,#47357,.F.);
#65676=ORIENTED_EDGE('',*,*,#47358,.F.);
#65677=ORIENTED_EDGE('',*,*,#47359,.T.);
#65678=ORIENTED_EDGE('',*,*,#47360,.T.);
#65679=ORIENTED_EDGE('',*,*,#47361,.F.);
#65680=ORIENTED_EDGE('',*,*,#47362,.F.);
#65681=ORIENTED_EDGE('',*,*,#47363,.T.);
#65682=ORIENTED_EDGE('',*,*,#47364,.T.);
#65683=ORIENTED_EDGE('',*,*,#47365,.T.);
#65684=ORIENTED_EDGE('',*,*,#47366,.T.);
#65685=ORIENTED_EDGE('',*,*,#47367,.T.);
#65686=ORIENTED_EDGE('',*,*,#47368,.T.);
#65687=ORIENTED_EDGE('',*,*,#47369,.T.);
#65688=ORIENTED_EDGE('',*,*,#47370,.T.);
#65689=ORIENTED_EDGE('',*,*,#47310,.T.);
#65690=ORIENTED_EDGE('',*,*,#47371,.T.);
#65691=ORIENTED_EDGE('',*,*,#47314,.T.);
#65692=ORIENTED_EDGE('',*,*,#47371,.F.);
#65693=ORIENTED_EDGE('',*,*,#47313,.T.);
#65694=ORIENTED_EDGE('',*,*,#47372,.F.);
#65695=ORIENTED_EDGE('',*,*,#47373,.F.);
#65696=ORIENTED_EDGE('',*,*,#47374,.F.);
#65697=ORIENTED_EDGE('',*,*,#47375,.F.);
#65698=ORIENTED_EDGE('',*,*,#47376,.F.);
#65699=ORIENTED_EDGE('',*,*,#47377,.F.);
#65700=ORIENTED_EDGE('',*,*,#47378,.F.);
#65701=ORIENTED_EDGE('',*,*,#47379,.F.);
#65702=ORIENTED_EDGE('',*,*,#47380,.F.);
#65703=ORIENTED_EDGE('',*,*,#47381,.F.);
#65704=ORIENTED_EDGE('',*,*,#47382,.F.);
#65705=ORIENTED_EDGE('',*,*,#47383,.F.);
#65706=ORIENTED_EDGE('',*,*,#47384,.F.);
#65707=ORIENTED_EDGE('',*,*,#47385,.F.);
#65708=ORIENTED_EDGE('',*,*,#47386,.F.);
#65709=ORIENTED_EDGE('',*,*,#47387,.F.);
#65710=ORIENTED_EDGE('',*,*,#47388,.F.);
#65711=ORIENTED_EDGE('',*,*,#47389,.F.);
#65712=ORIENTED_EDGE('',*,*,#47390,.F.);
#65713=ORIENTED_EDGE('',*,*,#47391,.F.);
#65714=ORIENTED_EDGE('',*,*,#47392,.F.);
#65715=ORIENTED_EDGE('',*,*,#47393,.F.);
#65716=ORIENTED_EDGE('',*,*,#47394,.F.);
#65717=ORIENTED_EDGE('',*,*,#47395,.F.);
#65718=ORIENTED_EDGE('',*,*,#47396,.F.);
#65719=ORIENTED_EDGE('',*,*,#47397,.F.);
#65720=ORIENTED_EDGE('',*,*,#47398,.F.);
#65721=ORIENTED_EDGE('',*,*,#47399,.F.);
#65722=ORIENTED_EDGE('',*,*,#47400,.F.);
#65723=ORIENTED_EDGE('',*,*,#47401,.F.);
#65724=ORIENTED_EDGE('',*,*,#47363,.F.);
#65725=ORIENTED_EDGE('',*,*,#47402,.F.);
#65726=ORIENTED_EDGE('',*,*,#47403,.F.);
#65727=ORIENTED_EDGE('',*,*,#47404,.F.);
#65728=ORIENTED_EDGE('',*,*,#47367,.F.);
#65729=ORIENTED_EDGE('',*,*,#47405,.F.);
#65730=ORIENTED_EDGE('',*,*,#47406,.F.);
#65731=ORIENTED_EDGE('',*,*,#47407,.F.);
#65732=ORIENTED_EDGE('',*,*,#47408,.F.);
#65733=ORIENTED_EDGE('',*,*,#47409,.F.);
#65734=ORIENTED_EDGE('',*,*,#47410,.F.);
#65735=ORIENTED_EDGE('',*,*,#47411,.F.);
#65736=ORIENTED_EDGE('',*,*,#47412,.F.);
#65737=ORIENTED_EDGE('',*,*,#47413,.F.);
#65738=ORIENTED_EDGE('',*,*,#47414,.F.);
#65739=ORIENTED_EDGE('',*,*,#47415,.F.);
#65740=ORIENTED_EDGE('',*,*,#47416,.F.);
#65741=ORIENTED_EDGE('',*,*,#47417,.F.);
#65742=ORIENTED_EDGE('',*,*,#47418,.F.);
#65743=ORIENTED_EDGE('',*,*,#47419,.F.);
#65744=ORIENTED_EDGE('',*,*,#47420,.F.);
#65745=ORIENTED_EDGE('',*,*,#47421,.F.);
#65746=ORIENTED_EDGE('',*,*,#47422,.F.);
#65747=ORIENTED_EDGE('',*,*,#47423,.F.);
#65748=ORIENTED_EDGE('',*,*,#47424,.F.);
#65749=ORIENTED_EDGE('',*,*,#47425,.F.);
#65750=ORIENTED_EDGE('',*,*,#47426,.F.);
#65751=ORIENTED_EDGE('',*,*,#47427,.F.);
#65752=ORIENTED_EDGE('',*,*,#47428,.F.);
#65753=ORIENTED_EDGE('',*,*,#47429,.F.);
#65754=ORIENTED_EDGE('',*,*,#47430,.F.);
#65755=ORIENTED_EDGE('',*,*,#47431,.F.);
#65756=ORIENTED_EDGE('',*,*,#47432,.F.);
#65757=ORIENTED_EDGE('',*,*,#47433,.F.);
#65758=ORIENTED_EDGE('',*,*,#47434,.F.);
#65759=ORIENTED_EDGE('',*,*,#47435,.F.);
#65760=ORIENTED_EDGE('',*,*,#47436,.F.);
#65761=ORIENTED_EDGE('',*,*,#47437,.F.);
#65762=ORIENTED_EDGE('',*,*,#47438,.F.);
#65763=ORIENTED_EDGE('',*,*,#47439,.F.);
#65764=ORIENTED_EDGE('',*,*,#47440,.F.);
#65765=ORIENTED_EDGE('',*,*,#47441,.F.);
#65766=ORIENTED_EDGE('',*,*,#47442,.F.);
#65767=ORIENTED_EDGE('',*,*,#47443,.F.);
#65768=ORIENTED_EDGE('',*,*,#47444,.F.);
#65769=ORIENTED_EDGE('',*,*,#47445,.F.);
#65770=ORIENTED_EDGE('',*,*,#47446,.F.);
#65771=ORIENTED_EDGE('',*,*,#47447,.F.);
#65772=ORIENTED_EDGE('',*,*,#47448,.F.);
#65773=ORIENTED_EDGE('',*,*,#47449,.F.);
#65774=ORIENTED_EDGE('',*,*,#47450,.F.);
#65775=ORIENTED_EDGE('',*,*,#47451,.F.);
#65776=ORIENTED_EDGE('',*,*,#47452,.F.);
#65777=ORIENTED_EDGE('',*,*,#47453,.F.);
#65778=ORIENTED_EDGE('',*,*,#47454,.F.);
#65779=ORIENTED_EDGE('',*,*,#47455,.F.);
#65780=ORIENTED_EDGE('',*,*,#47456,.F.);
#65781=ORIENTED_EDGE('',*,*,#47457,.F.);
#65782=ORIENTED_EDGE('',*,*,#47458,.F.);
#65783=ORIENTED_EDGE('',*,*,#47459,.F.);
#65784=ORIENTED_EDGE('',*,*,#47460,.F.);
#65785=ORIENTED_EDGE('',*,*,#47461,.F.);
#65786=ORIENTED_EDGE('',*,*,#47462,.F.);
#65787=ORIENTED_EDGE('',*,*,#47463,.F.);
#65788=ORIENTED_EDGE('',*,*,#47464,.F.);
#65789=ORIENTED_EDGE('',*,*,#47465,.F.);
#65790=ORIENTED_EDGE('',*,*,#47466,.F.);
#65791=ORIENTED_EDGE('',*,*,#47467,.F.);
#65792=ORIENTED_EDGE('',*,*,#47468,.F.);
#65793=ORIENTED_EDGE('',*,*,#47469,.F.);
#65794=ORIENTED_EDGE('',*,*,#47470,.F.);
#65795=ORIENTED_EDGE('',*,*,#47471,.F.);
#65796=ORIENTED_EDGE('',*,*,#47472,.F.);
#65797=ORIENTED_EDGE('',*,*,#47473,.F.);
#65798=ORIENTED_EDGE('',*,*,#47474,.F.);
#65799=ORIENTED_EDGE('',*,*,#47475,.F.);
#65800=ORIENTED_EDGE('',*,*,#47476,.F.);
#65801=ORIENTED_EDGE('',*,*,#47477,.F.);
#65802=ORIENTED_EDGE('',*,*,#47478,.F.);
#65803=ORIENTED_EDGE('',*,*,#47479,.F.);
#65804=ORIENTED_EDGE('',*,*,#47480,.F.);
#65805=ORIENTED_EDGE('',*,*,#47481,.F.);
#65806=ORIENTED_EDGE('',*,*,#47482,.F.);
#65807=ORIENTED_EDGE('',*,*,#47483,.F.);
#65808=ORIENTED_EDGE('',*,*,#47484,.F.);
#65809=ORIENTED_EDGE('',*,*,#47485,.F.);
#65810=ORIENTED_EDGE('',*,*,#47486,.F.);
#65811=ORIENTED_EDGE('',*,*,#47487,.F.);
#65812=ORIENTED_EDGE('',*,*,#47488,.F.);
#65813=ORIENTED_EDGE('',*,*,#47489,.F.);
#65814=ORIENTED_EDGE('',*,*,#47355,.F.);
#65815=ORIENTED_EDGE('',*,*,#47490,.F.);
#65816=ORIENTED_EDGE('',*,*,#47491,.F.);
#65817=ORIENTED_EDGE('',*,*,#47492,.F.);
#65818=ORIENTED_EDGE('',*,*,#47359,.F.);
#65819=ORIENTED_EDGE('',*,*,#47493,.F.);
#65820=ORIENTED_EDGE('',*,*,#47494,.F.);
#65821=ORIENTED_EDGE('',*,*,#47495,.F.);
#65822=ORIENTED_EDGE('',*,*,#47496,.F.);
#65823=ORIENTED_EDGE('',*,*,#47497,.F.);
#65824=ORIENTED_EDGE('',*,*,#47498,.F.);
#65825=ORIENTED_EDGE('',*,*,#47499,.F.);
#65826=ORIENTED_EDGE('',*,*,#47500,.F.);
#65827=ORIENTED_EDGE('',*,*,#47501,.F.);
#65828=ORIENTED_EDGE('',*,*,#47502,.F.);
#65829=ORIENTED_EDGE('',*,*,#47503,.F.);
#65830=ORIENTED_EDGE('',*,*,#47504,.F.);
#65831=ORIENTED_EDGE('',*,*,#47505,.F.);
#65832=ORIENTED_EDGE('',*,*,#47506,.F.);
#65833=ORIENTED_EDGE('',*,*,#47507,.F.);
#65834=ORIENTED_EDGE('',*,*,#47508,.F.);
#65835=ORIENTED_EDGE('',*,*,#47509,.F.);
#65836=ORIENTED_EDGE('',*,*,#47510,.F.);
#65837=ORIENTED_EDGE('',*,*,#47511,.F.);
#65838=ORIENTED_EDGE('',*,*,#47512,.F.);
#65839=ORIENTED_EDGE('',*,*,#47513,.F.);
#65840=ORIENTED_EDGE('',*,*,#47514,.F.);
#65841=ORIENTED_EDGE('',*,*,#47515,.F.);
#65842=ORIENTED_EDGE('',*,*,#47307,.T.);
#65843=ORIENTED_EDGE('',*,*,#47304,.T.);
#65844=ORIENTED_EDGE('',*,*,#47516,.T.);
#65845=ORIENTED_EDGE('',*,*,#47517,.T.);
#65846=ORIENTED_EDGE('',*,*,#47518,.T.);
#65847=ORIENTED_EDGE('',*,*,#47327,.T.);
#65848=ORIENTED_EDGE('',*,*,#47519,.T.);
#65849=ORIENTED_EDGE('',*,*,#47520,.T.);
#65850=ORIENTED_EDGE('',*,*,#47521,.T.);
#65851=ORIENTED_EDGE('',*,*,#47522,.T.);
#65852=ORIENTED_EDGE('',*,*,#47523,.T.);
#65853=ORIENTED_EDGE('',*,*,#47524,.T.);
#65854=ORIENTED_EDGE('',*,*,#47525,.T.);
#65855=ORIENTED_EDGE('',*,*,#47323,.T.);
#65856=ORIENTED_EDGE('',*,*,#47526,.T.);
#65857=ORIENTED_EDGE('',*,*,#47527,.T.);
#65858=ORIENTED_EDGE('',*,*,#47528,.T.);
#65859=ORIENTED_EDGE('',*,*,#47529,.T.);
#65860=ORIENTED_EDGE('',*,*,#47329,.T.);
#65861=ORIENTED_EDGE('',*,*,#47530,.F.);
#65862=ORIENTED_EDGE('',*,*,#47515,.T.);
#65863=ORIENTED_EDGE('',*,*,#47531,.F.);
#65864=ORIENTED_EDGE('',*,*,#47532,.F.);
#65865=ORIENTED_EDGE('',*,*,#47533,.F.);
#65866=ORIENTED_EDGE('',*,*,#47534,.F.);
#65867=ORIENTED_EDGE('',*,*,#47535,.F.);
#65868=ORIENTED_EDGE('',*,*,#47375,.T.);
#65869=ORIENTED_EDGE('',*,*,#47536,.F.);
#65870=ORIENTED_EDGE('',*,*,#47511,.T.);
#65871=ORIENTED_EDGE('',*,*,#47537,.F.);
#65872=ORIENTED_EDGE('',*,*,#47538,.F.);
#65873=ORIENTED_EDGE('',*,*,#47539,.F.);
#65874=ORIENTED_EDGE('',*,*,#47507,.T.);
#65875=ORIENTED_EDGE('',*,*,#47540,.F.);
#65876=ORIENTED_EDGE('',*,*,#47541,.F.);
#65877=ORIENTED_EDGE('',*,*,#47542,.F.);
#65878=ORIENTED_EDGE('',*,*,#47503,.T.);
#65879=ORIENTED_EDGE('',*,*,#47543,.F.);
#65880=ORIENTED_EDGE('',*,*,#47544,.F.);
#65881=ORIENTED_EDGE('',*,*,#47356,.F.);
#65882=ORIENTED_EDGE('',*,*,#47489,.T.);
#65883=ORIENTED_EDGE('',*,*,#47545,.F.);
#65884=ORIENTED_EDGE('',*,*,#47546,.F.);
#65885=ORIENTED_EDGE('',*,*,#47547,.F.);
#65886=ORIENTED_EDGE('',*,*,#47548,.F.);
#65887=ORIENTED_EDGE('',*,*,#47360,.F.);
#65888=ORIENTED_EDGE('',*,*,#47492,.T.);
#65889=ORIENTED_EDGE('',*,*,#47549,.F.);
#65890=ORIENTED_EDGE('',*,*,#47550,.F.);
#65891=ORIENTED_EDGE('',*,*,#47551,.F.);
#65892=ORIENTED_EDGE('',*,*,#47495,.T.);
#65893=ORIENTED_EDGE('',*,*,#47552,.F.);
#65894=ORIENTED_EDGE('',*,*,#47499,.T.);
#65895=ORIENTED_EDGE('',*,*,#47553,.F.);
#65896=ORIENTED_EDGE('',*,*,#47554,.F.);
#65897=ORIENTED_EDGE('',*,*,#47555,.F.);
#65898=ORIENTED_EDGE('',*,*,#47395,.T.);
#65899=ORIENTED_EDGE('',*,*,#47556,.F.);
#65900=ORIENTED_EDGE('',*,*,#47557,.F.);
#65901=ORIENTED_EDGE('',*,*,#47558,.F.);
#65902=ORIENTED_EDGE('',*,*,#47559,.F.);
#65903=ORIENTED_EDGE('',*,*,#47560,.F.);
#65904=ORIENTED_EDGE('',*,*,#47399,.T.);
#65905=ORIENTED_EDGE('',*,*,#47561,.F.);
#65906=ORIENTED_EDGE('',*,*,#47391,.T.);
#65907=ORIENTED_EDGE('',*,*,#47562,.F.);
#65908=ORIENTED_EDGE('',*,*,#47563,.F.);
#65909=ORIENTED_EDGE('',*,*,#47366,.F.);
#65910=ORIENTED_EDGE('',*,*,#47564,.F.);
#65911=ORIENTED_EDGE('',*,*,#47565,.F.);
#65912=ORIENTED_EDGE('',*,*,#47402,.T.);
#65913=ORIENTED_EDGE('',*,*,#47370,.F.);
#65914=ORIENTED_EDGE('',*,*,#47566,.F.);
#65915=ORIENTED_EDGE('',*,*,#47567,.F.);
#65916=ORIENTED_EDGE('',*,*,#47405,.T.);
#65917=ORIENTED_EDGE('',*,*,#47568,.F.);
#65918=ORIENTED_EDGE('',*,*,#47569,.F.);
#65919=ORIENTED_EDGE('',*,*,#47570,.F.);
#65920=ORIENTED_EDGE('',*,*,#47409,.T.);
#65921=ORIENTED_EDGE('',*,*,#47571,.F.);
#65922=ORIENTED_EDGE('',*,*,#47383,.T.);
#65923=ORIENTED_EDGE('',*,*,#47572,.F.);
#65924=ORIENTED_EDGE('',*,*,#47573,.F.);
#65925=ORIENTED_EDGE('',*,*,#47574,.F.);
#65926=ORIENTED_EDGE('',*,*,#47575,.F.);
#65927=ORIENTED_EDGE('',*,*,#47576,.F.);
#65928=ORIENTED_EDGE('',*,*,#47387,.T.);
#65929=ORIENTED_EDGE('',*,*,#47577,.F.);
#65930=ORIENTED_EDGE('',*,*,#47379,.T.);
#65931=ORIENTED_EDGE('',*,*,#47578,.F.);
#65932=ORIENTED_EDGE('',*,*,#47579,.F.);
#65933=ORIENTED_EDGE('',*,*,#47580,.F.);
#65934=ORIENTED_EDGE('',*,*,#47429,.T.);
#65935=ORIENTED_EDGE('',*,*,#47581,.F.);
#65936=ORIENTED_EDGE('',*,*,#47582,.F.);
#65937=ORIENTED_EDGE('',*,*,#47583,.F.);
#65938=ORIENTED_EDGE('',*,*,#47584,.F.);
#65939=ORIENTED_EDGE('',*,*,#47585,.F.);
#65940=ORIENTED_EDGE('',*,*,#47433,.T.);
#65941=ORIENTED_EDGE('',*,*,#47586,.F.);
#65942=ORIENTED_EDGE('',*,*,#47425,.T.);
#65943=ORIENTED_EDGE('',*,*,#47587,.F.);
#65944=ORIENTED_EDGE('',*,*,#47588,.F.);
#65945=ORIENTED_EDGE('',*,*,#47589,.F.);
#65946=ORIENTED_EDGE('',*,*,#47590,.F.);
#65947=ORIENTED_EDGE('',*,*,#47591,.F.);
#65948=ORIENTED_EDGE('',*,*,#47437,.T.);
#65949=ORIENTED_EDGE('',*,*,#47592,.F.);
#65950=ORIENTED_EDGE('',*,*,#47593,.F.);
#65951=ORIENTED_EDGE('',*,*,#47594,.F.);
#65952=ORIENTED_EDGE('',*,*,#47441,.T.);
#65953=ORIENTED_EDGE('',*,*,#47595,.F.);
#65954=ORIENTED_EDGE('',*,*,#47596,.F.);
#65955=ORIENTED_EDGE('',*,*,#47597,.F.);
#65956=ORIENTED_EDGE('',*,*,#47445,.T.);
#65957=ORIENTED_EDGE('',*,*,#47598,.F.);
#65958=ORIENTED_EDGE('',*,*,#47417,.T.);
#65959=ORIENTED_EDGE('',*,*,#47599,.F.);
#65960=ORIENTED_EDGE('',*,*,#47600,.F.);
#65961=ORIENTED_EDGE('',*,*,#47601,.F.);
#65962=ORIENTED_EDGE('',*,*,#47602,.F.);
#65963=ORIENTED_EDGE('',*,*,#47603,.F.);
#65964=ORIENTED_EDGE('',*,*,#47421,.T.);
#65965=ORIENTED_EDGE('',*,*,#47604,.F.);
#65966=ORIENTED_EDGE('',*,*,#47413,.T.);
#65967=ORIENTED_EDGE('',*,*,#47605,.F.);
#65968=ORIENTED_EDGE('',*,*,#47606,.F.);
#65969=ORIENTED_EDGE('',*,*,#47607,.F.);
#65970=ORIENTED_EDGE('',*,*,#47465,.T.);
#65971=ORIENTED_EDGE('',*,*,#47608,.F.);
#65972=ORIENTED_EDGE('',*,*,#47609,.F.);
#65973=ORIENTED_EDGE('',*,*,#47610,.F.);
#65974=ORIENTED_EDGE('',*,*,#47611,.F.);
#65975=ORIENTED_EDGE('',*,*,#47612,.F.);
#65976=ORIENTED_EDGE('',*,*,#47469,.T.);
#65977=ORIENTED_EDGE('',*,*,#47613,.F.);
#65978=ORIENTED_EDGE('',*,*,#47461,.T.);
#65979=ORIENTED_EDGE('',*,*,#47614,.F.);
#65980=ORIENTED_EDGE('',*,*,#47615,.F.);
#65981=ORIENTED_EDGE('',*,*,#47616,.F.);
#65982=ORIENTED_EDGE('',*,*,#47617,.F.);
#65983=ORIENTED_EDGE('',*,*,#47618,.F.);
#65984=ORIENTED_EDGE('',*,*,#47473,.T.);
#65985=ORIENTED_EDGE('',*,*,#47619,.F.);
#65986=ORIENTED_EDGE('',*,*,#47620,.F.);
#65987=ORIENTED_EDGE('',*,*,#47621,.F.);
#65988=ORIENTED_EDGE('',*,*,#47477,.T.);
#65989=ORIENTED_EDGE('',*,*,#47622,.F.);
#65990=ORIENTED_EDGE('',*,*,#47623,.F.);
#65991=ORIENTED_EDGE('',*,*,#47624,.F.);
#65992=ORIENTED_EDGE('',*,*,#47481,.T.);
#65993=ORIENTED_EDGE('',*,*,#47625,.F.);
#65994=ORIENTED_EDGE('',*,*,#47457,.T.);
#65995=ORIENTED_EDGE('',*,*,#47626,.F.);
#65996=ORIENTED_EDGE('',*,*,#47627,.F.);
#65997=ORIENTED_EDGE('',*,*,#47628,.F.);
#65998=ORIENTED_EDGE('',*,*,#47453,.T.);
#65999=ORIENTED_EDGE('',*,*,#47629,.F.);
#66000=ORIENTED_EDGE('',*,*,#47630,.F.);
#66001=ORIENTED_EDGE('',*,*,#47631,.F.);
#66002=ORIENTED_EDGE('',*,*,#47449,.T.);
#66003=ORIENTED_EDGE('',*,*,#47632,.F.);
#66004=ORIENTED_EDGE('',*,*,#47633,.F.);
#66005=ORIENTED_EDGE('',*,*,#47634,.T.);
#66006=ORIENTED_EDGE('',*,*,#47532,.T.);
#66007=ORIENTED_EDGE('',*,*,#47635,.F.);
#66008=ORIENTED_EDGE('',*,*,#47636,.T.);
#66009=ORIENTED_EDGE('',*,*,#47637,.T.);
#66010=ORIENTED_EDGE('',*,*,#47538,.T.);
#66011=ORIENTED_EDGE('',*,*,#47638,.F.);
#66012=ORIENTED_EDGE('',*,*,#47639,.T.);
#66013=ORIENTED_EDGE('',*,*,#47640,.T.);
#66014=ORIENTED_EDGE('',*,*,#47541,.T.);
#66015=ORIENTED_EDGE('',*,*,#47641,.F.);
#66016=ORIENTED_EDGE('',*,*,#47642,.T.);
#66017=ORIENTED_EDGE('',*,*,#47643,.T.);
#66018=ORIENTED_EDGE('',*,*,#47544,.T.);
#66019=ORIENTED_EDGE('',*,*,#47644,.F.);
#66020=ORIENTED_EDGE('',*,*,#47645,.T.);
#66021=ORIENTED_EDGE('',*,*,#47646,.T.);
#66022=ORIENTED_EDGE('',*,*,#47554,.T.);
#66023=ORIENTED_EDGE('',*,*,#47647,.F.);
#66024=ORIENTED_EDGE('',*,*,#47648,.T.);
#66025=ORIENTED_EDGE('',*,*,#47649,.T.);
#66026=ORIENTED_EDGE('',*,*,#47550,.T.);
#66027=ORIENTED_EDGE('',*,*,#47650,.F.);
#66028=ORIENTED_EDGE('',*,*,#47651,.T.);
#66029=ORIENTED_EDGE('',*,*,#47361,.T.);
#66030=ORIENTED_EDGE('',*,*,#47548,.T.);
#66031=ORIENTED_EDGE('',*,*,#47652,.F.);
#66032=ORIENTED_EDGE('',*,*,#47653,.T.);
#66033=ORIENTED_EDGE('',*,*,#47357,.T.);
#66034=ORIENTED_EDGE('',*,*,#47546,.T.);
#66035=ORIENTED_EDGE('',*,*,#47654,.F.);
#66036=ORIENTED_EDGE('',*,*,#47655,.T.);
#66037=ORIENTED_EDGE('',*,*,#47656,.T.);
#66038=ORIENTED_EDGE('',*,*,#47657,.T.);
#66039=ORIENTED_EDGE('',*,*,#47658,.F.);
#66040=ORIENTED_EDGE('',*,*,#47659,.T.);
#66041=ORIENTED_EDGE('',*,*,#47660,.T.);
#66042=ORIENTED_EDGE('',*,*,#47623,.T.);
#66043=ORIENTED_EDGE('',*,*,#47661,.F.);
#66044=ORIENTED_EDGE('',*,*,#47662,.T.);
#66045=ORIENTED_EDGE('',*,*,#47663,.T.);
#66046=ORIENTED_EDGE('',*,*,#47620,.T.);
#66047=ORIENTED_EDGE('',*,*,#47664,.F.);
#66048=ORIENTED_EDGE('',*,*,#47665,.T.);
#66049=ORIENTED_EDGE('',*,*,#47666,.T.);
#66050=ORIENTED_EDGE('',*,*,#47617,.T.);
#66051=ORIENTED_EDGE('',*,*,#47667,.F.);
#66052=ORIENTED_EDGE('',*,*,#47668,.T.);
#66053=ORIENTED_EDGE('',*,*,#47669,.T.);
#66054=ORIENTED_EDGE('',*,*,#47611,.T.);
#66055=ORIENTED_EDGE('',*,*,#47670,.F.);
#66056=ORIENTED_EDGE('',*,*,#47671,.T.);
#66057=ORIENTED_EDGE('',*,*,#47672,.T.);
#66058=ORIENTED_EDGE('',*,*,#47609,.T.);
#66059=ORIENTED_EDGE('',*,*,#47673,.F.);
#66060=ORIENTED_EDGE('',*,*,#47674,.T.);
#66061=ORIENTED_EDGE('',*,*,#47675,.T.);
#66062=ORIENTED_EDGE('',*,*,#47615,.T.);
#66063=ORIENTED_EDGE('',*,*,#47676,.F.);
#66064=ORIENTED_EDGE('',*,*,#47677,.T.);
#66065=ORIENTED_EDGE('',*,*,#47678,.T.);
#66066=ORIENTED_EDGE('',*,*,#47627,.T.);
#66067=ORIENTED_EDGE('',*,*,#47679,.F.);
#66068=ORIENTED_EDGE('',*,*,#47680,.T.);
#66069=ORIENTED_EDGE('',*,*,#47681,.T.);
#66070=ORIENTED_EDGE('',*,*,#47630,.T.);
#66071=ORIENTED_EDGE('',*,*,#47682,.F.);
#66072=ORIENTED_EDGE('',*,*,#47683,.T.);
#66073=ORIENTED_EDGE('',*,*,#47684,.T.);
#66074=ORIENTED_EDGE('',*,*,#47633,.T.);
#66075=ORIENTED_EDGE('',*,*,#47685,.F.);
#66076=ORIENTED_EDGE('',*,*,#47686,.T.);
#66077=ORIENTED_EDGE('',*,*,#47687,.T.);
#66078=ORIENTED_EDGE('',*,*,#47596,.T.);
#66079=ORIENTED_EDGE('',*,*,#47688,.F.);
#66080=ORIENTED_EDGE('',*,*,#47689,.T.);
#66081=ORIENTED_EDGE('',*,*,#47690,.T.);
#66082=ORIENTED_EDGE('',*,*,#47593,.T.);
#66083=ORIENTED_EDGE('',*,*,#47691,.F.);
#66084=ORIENTED_EDGE('',*,*,#47692,.T.);
#66085=ORIENTED_EDGE('',*,*,#47693,.T.);
#66086=ORIENTED_EDGE('',*,*,#47590,.T.);
#66087=ORIENTED_EDGE('',*,*,#47694,.F.);
#66088=ORIENTED_EDGE('',*,*,#47695,.T.);
#66089=ORIENTED_EDGE('',*,*,#47696,.T.);
#66090=ORIENTED_EDGE('',*,*,#47584,.T.);
#66091=ORIENTED_EDGE('',*,*,#47697,.F.);
#66092=ORIENTED_EDGE('',*,*,#47698,.T.);
#66093=ORIENTED_EDGE('',*,*,#47699,.T.);
#66094=ORIENTED_EDGE('',*,*,#47582,.T.);
#66095=ORIENTED_EDGE('',*,*,#47700,.F.);
#66096=ORIENTED_EDGE('',*,*,#47701,.T.);
#66097=ORIENTED_EDGE('',*,*,#47702,.T.);
#66098=ORIENTED_EDGE('',*,*,#47588,.T.);
#66099=ORIENTED_EDGE('',*,*,#47703,.F.);
#66100=ORIENTED_EDGE('',*,*,#47704,.T.);
#66101=ORIENTED_EDGE('',*,*,#47705,.T.);
#66102=ORIENTED_EDGE('',*,*,#47602,.T.);
#66103=ORIENTED_EDGE('',*,*,#47706,.F.);
#66104=ORIENTED_EDGE('',*,*,#47707,.T.);
#66105=ORIENTED_EDGE('',*,*,#47708,.T.);
#66106=ORIENTED_EDGE('',*,*,#47600,.T.);
#66107=ORIENTED_EDGE('',*,*,#47709,.F.);
#66108=ORIENTED_EDGE('',*,*,#47710,.T.);
#66109=ORIENTED_EDGE('',*,*,#47711,.T.);
#66110=ORIENTED_EDGE('',*,*,#47606,.T.);
#66111=ORIENTED_EDGE('',*,*,#47712,.F.);
#66112=ORIENTED_EDGE('',*,*,#47713,.T.);
#66113=ORIENTED_EDGE('',*,*,#47714,.T.);
#66114=ORIENTED_EDGE('',*,*,#47569,.T.);
#66115=ORIENTED_EDGE('',*,*,#47715,.F.);
#66116=ORIENTED_EDGE('',*,*,#47716,.T.);
#66117=ORIENTED_EDGE('',*,*,#47717,.T.);
#66118=ORIENTED_EDGE('',*,*,#47566,.T.);
#66119=ORIENTED_EDGE('',*,*,#47369,.F.);
#66120=ORIENTED_EDGE('',*,*,#47718,.T.);
#66121=ORIENTED_EDGE('',*,*,#47719,.T.);
#66122=ORIENTED_EDGE('',*,*,#47564,.T.);
#66123=ORIENTED_EDGE('',*,*,#47365,.F.);
#66124=ORIENTED_EDGE('',*,*,#47720,.T.);
#66125=ORIENTED_EDGE('',*,*,#47721,.T.);
#66126=ORIENTED_EDGE('',*,*,#47559,.T.);
#66127=ORIENTED_EDGE('',*,*,#47722,.F.);
#66128=ORIENTED_EDGE('',*,*,#47723,.T.);
#66129=ORIENTED_EDGE('',*,*,#47724,.T.);
#66130=ORIENTED_EDGE('',*,*,#47557,.T.);
#66131=ORIENTED_EDGE('',*,*,#47725,.F.);
#66132=ORIENTED_EDGE('',*,*,#47726,.T.);
#66133=ORIENTED_EDGE('',*,*,#47727,.T.);
#66134=ORIENTED_EDGE('',*,*,#47563,.T.);
#66135=ORIENTED_EDGE('',*,*,#47728,.F.);
#66136=ORIENTED_EDGE('',*,*,#47729,.T.);
#66137=ORIENTED_EDGE('',*,*,#47730,.T.);
#66138=ORIENTED_EDGE('',*,*,#47575,.T.);
#66139=ORIENTED_EDGE('',*,*,#47731,.F.);
#66140=ORIENTED_EDGE('',*,*,#47732,.T.);
#66141=ORIENTED_EDGE('',*,*,#47733,.T.);
#66142=ORIENTED_EDGE('',*,*,#47573,.T.);
#66143=ORIENTED_EDGE('',*,*,#47734,.F.);
#66144=ORIENTED_EDGE('',*,*,#47735,.T.);
#66145=ORIENTED_EDGE('',*,*,#47736,.T.);
#66146=ORIENTED_EDGE('',*,*,#47579,.T.);
#66147=ORIENTED_EDGE('',*,*,#47737,.F.);
#66148=ORIENTED_EDGE('',*,*,#47738,.T.);
#66149=ORIENTED_EDGE('',*,*,#47739,.T.);
#66150=ORIENTED_EDGE('',*,*,#47534,.T.);
#66151=ORIENTED_EDGE('',*,*,#47740,.F.);
#66152=ORIENTED_EDGE('',*,*,#47741,.T.);
#66153=ORIENTED_EDGE('',*,*,#47300,.F.);
#66154=ORIENTED_EDGE('',*,*,#47303,.F.);
#66155=ORIENTED_EDGE('',*,*,#47353,.F.);
#66156=ORIENTED_EDGE('',*,*,#47742,.F.);
#66157=ORIENTED_EDGE('',*,*,#47485,.T.);
#66158=ORIENTED_EDGE('',*,*,#47743,.F.);
#66159=ORIENTED_EDGE('',*,*,#47657,.F.);
#66160=ORIENTED_EDGE('',*,*,#47624,.T.);
#66161=ORIENTED_EDGE('',*,*,#47660,.F.);
#66162=ORIENTED_EDGE('',*,*,#47744,.F.);
#66163=ORIENTED_EDGE('',*,*,#47482,.T.);
#66164=ORIENTED_EDGE('',*,*,#47743,.T.);
#66165=ORIENTED_EDGE('',*,*,#47484,.T.);
#66166=ORIENTED_EDGE('',*,*,#47745,.T.);
#66167=ORIENTED_EDGE('',*,*,#47658,.T.);
#66168=ORIENTED_EDGE('',*,*,#47659,.F.);
#66169=ORIENTED_EDGE('',*,*,#47745,.F.);
#66170=ORIENTED_EDGE('',*,*,#47483,.T.);
#66171=ORIENTED_EDGE('',*,*,#47744,.T.);
#66172=ORIENTED_EDGE('',*,*,#47742,.T.);
#66173=ORIENTED_EDGE('',*,*,#47656,.F.);
#66174=ORIENTED_EDGE('',*,*,#47746,.F.);
#66175=ORIENTED_EDGE('',*,*,#47486,.T.);
#66176=ORIENTED_EDGE('',*,*,#47545,.T.);
#66177=ORIENTED_EDGE('',*,*,#47488,.T.);
#66178=ORIENTED_EDGE('',*,*,#47747,.T.);
#66179=ORIENTED_EDGE('',*,*,#47654,.T.);
#66180=ORIENTED_EDGE('',*,*,#47655,.F.);
#66181=ORIENTED_EDGE('',*,*,#47747,.F.);
#66182=ORIENTED_EDGE('',*,*,#47487,.T.);
#66183=ORIENTED_EDGE('',*,*,#47746,.T.);
#66184=ORIENTED_EDGE('',*,*,#47597,.T.);
#66185=ORIENTED_EDGE('',*,*,#47687,.F.);
#66186=ORIENTED_EDGE('',*,*,#47748,.F.);
#66187=ORIENTED_EDGE('',*,*,#47446,.T.);
#66188=ORIENTED_EDGE('',*,*,#47632,.T.);
#66189=ORIENTED_EDGE('',*,*,#47448,.T.);
#66190=ORIENTED_EDGE('',*,*,#47749,.T.);
#66191=ORIENTED_EDGE('',*,*,#47685,.T.);
#66192=ORIENTED_EDGE('',*,*,#47686,.F.);
#66193=ORIENTED_EDGE('',*,*,#47749,.F.);
#66194=ORIENTED_EDGE('',*,*,#47447,.T.);
#66195=ORIENTED_EDGE('',*,*,#47748,.T.);
#66196=ORIENTED_EDGE('',*,*,#47631,.T.);
#66197=ORIENTED_EDGE('',*,*,#47684,.F.);
#66198=ORIENTED_EDGE('',*,*,#47750,.F.);
#66199=ORIENTED_EDGE('',*,*,#47450,.T.);
#66200=ORIENTED_EDGE('',*,*,#47629,.T.);
#66201=ORIENTED_EDGE('',*,*,#47452,.T.);
#66202=ORIENTED_EDGE('',*,*,#47751,.T.);
#66203=ORIENTED_EDGE('',*,*,#47682,.T.);
#66204=ORIENTED_EDGE('',*,*,#47683,.F.);
#66205=ORIENTED_EDGE('',*,*,#47751,.F.);
#66206=ORIENTED_EDGE('',*,*,#47451,.T.);
#66207=ORIENTED_EDGE('',*,*,#47750,.T.);
#66208=ORIENTED_EDGE('',*,*,#47628,.T.);
#66209=ORIENTED_EDGE('',*,*,#47681,.F.);
#66210=ORIENTED_EDGE('',*,*,#47752,.F.);
#66211=ORIENTED_EDGE('',*,*,#47454,.T.);
#66212=ORIENTED_EDGE('',*,*,#47626,.T.);
#66213=ORIENTED_EDGE('',*,*,#47456,.T.);
#66214=ORIENTED_EDGE('',*,*,#47753,.T.);
#66215=ORIENTED_EDGE('',*,*,#47679,.T.);
#66216=ORIENTED_EDGE('',*,*,#47680,.F.);
#66217=ORIENTED_EDGE('',*,*,#47753,.F.);
#66218=ORIENTED_EDGE('',*,*,#47455,.T.);
#66219=ORIENTED_EDGE('',*,*,#47752,.T.);
#66220=ORIENTED_EDGE('',*,*,#47625,.T.);
#66221=ORIENTED_EDGE('',*,*,#47678,.F.);
#66222=ORIENTED_EDGE('',*,*,#47754,.F.);
#66223=ORIENTED_EDGE('',*,*,#47458,.T.);
#66224=ORIENTED_EDGE('',*,*,#47614,.T.);
#66225=ORIENTED_EDGE('',*,*,#47460,.T.);
#66226=ORIENTED_EDGE('',*,*,#47755,.T.);
#66227=ORIENTED_EDGE('',*,*,#47676,.T.);
#66228=ORIENTED_EDGE('',*,*,#47677,.F.);
#66229=ORIENTED_EDGE('',*,*,#47755,.F.);
#66230=ORIENTED_EDGE('',*,*,#47459,.T.);
#66231=ORIENTED_EDGE('',*,*,#47754,.T.);
#66232=ORIENTED_EDGE('',*,*,#47621,.T.);
#66233=ORIENTED_EDGE('',*,*,#47663,.F.);
#66234=ORIENTED_EDGE('',*,*,#47756,.F.);
#66235=ORIENTED_EDGE('',*,*,#47478,.T.);
#66236=ORIENTED_EDGE('',*,*,#47622,.T.);
#66237=ORIENTED_EDGE('',*,*,#47480,.T.);
#66238=ORIENTED_EDGE('',*,*,#47757,.T.);
#66239=ORIENTED_EDGE('',*,*,#47661,.T.);
#66240=ORIENTED_EDGE('',*,*,#47662,.F.);
#66241=ORIENTED_EDGE('',*,*,#47757,.F.);
#66242=ORIENTED_EDGE('',*,*,#47479,.T.);
#66243=ORIENTED_EDGE('',*,*,#47756,.T.);
#66244=ORIENTED_EDGE('',*,*,#47618,.T.);
#66245=ORIENTED_EDGE('',*,*,#47666,.F.);
#66246=ORIENTED_EDGE('',*,*,#47758,.F.);
#66247=ORIENTED_EDGE('',*,*,#47474,.T.);
#66248=ORIENTED_EDGE('',*,*,#47619,.T.);
#66249=ORIENTED_EDGE('',*,*,#47476,.T.);
#66250=ORIENTED_EDGE('',*,*,#47759,.T.);
#66251=ORIENTED_EDGE('',*,*,#47664,.T.);
#66252=ORIENTED_EDGE('',*,*,#47665,.F.);
#66253=ORIENTED_EDGE('',*,*,#47759,.F.);
#66254=ORIENTED_EDGE('',*,*,#47475,.T.);
#66255=ORIENTED_EDGE('',*,*,#47758,.T.);
#66256=ORIENTED_EDGE('',*,*,#47612,.T.);
#66257=ORIENTED_EDGE('',*,*,#47669,.F.);
#66258=ORIENTED_EDGE('',*,*,#47760,.F.);
#66259=ORIENTED_EDGE('',*,*,#47470,.T.);
#66260=ORIENTED_EDGE('',*,*,#47616,.T.);
#66261=ORIENTED_EDGE('',*,*,#47472,.T.);
#66262=ORIENTED_EDGE('',*,*,#47761,.T.);
#66263=ORIENTED_EDGE('',*,*,#47667,.T.);
#66264=ORIENTED_EDGE('',*,*,#47668,.F.);
#66265=ORIENTED_EDGE('',*,*,#47761,.F.);
#66266=ORIENTED_EDGE('',*,*,#47471,.T.);
#66267=ORIENTED_EDGE('',*,*,#47760,.T.);
#66268=ORIENTED_EDGE('',*,*,#47613,.T.);
#66269=ORIENTED_EDGE('',*,*,#47675,.F.);
#66270=ORIENTED_EDGE('',*,*,#47762,.F.);
#66271=ORIENTED_EDGE('',*,*,#47462,.T.);
#66272=ORIENTED_EDGE('',*,*,#47608,.T.);
#66273=ORIENTED_EDGE('',*,*,#47464,.T.);
#66274=ORIENTED_EDGE('',*,*,#47763,.T.);
#66275=ORIENTED_EDGE('',*,*,#47673,.T.);
#66276=ORIENTED_EDGE('',*,*,#47674,.F.);
#66277=ORIENTED_EDGE('',*,*,#47763,.F.);
#66278=ORIENTED_EDGE('',*,*,#47463,.T.);
#66279=ORIENTED_EDGE('',*,*,#47762,.T.);
#66280=ORIENTED_EDGE('',*,*,#47607,.T.);
#66281=ORIENTED_EDGE('',*,*,#47672,.F.);
#66282=ORIENTED_EDGE('',*,*,#47764,.F.);
#66283=ORIENTED_EDGE('',*,*,#47466,.T.);
#66284=ORIENTED_EDGE('',*,*,#47610,.T.);
#66285=ORIENTED_EDGE('',*,*,#47468,.T.);
#66286=ORIENTED_EDGE('',*,*,#47765,.T.);
#66287=ORIENTED_EDGE('',*,*,#47670,.T.);
#66288=ORIENTED_EDGE('',*,*,#47671,.F.);
#66289=ORIENTED_EDGE('',*,*,#47765,.F.);
#66290=ORIENTED_EDGE('',*,*,#47467,.T.);
#66291=ORIENTED_EDGE('',*,*,#47764,.T.);
#66292=ORIENTED_EDGE('',*,*,#47570,.T.);
#66293=ORIENTED_EDGE('',*,*,#47714,.F.);
#66294=ORIENTED_EDGE('',*,*,#47766,.F.);
#66295=ORIENTED_EDGE('',*,*,#47410,.T.);
#66296=ORIENTED_EDGE('',*,*,#47605,.T.);
#66297=ORIENTED_EDGE('',*,*,#47412,.T.);
#66298=ORIENTED_EDGE('',*,*,#47767,.T.);
#66299=ORIENTED_EDGE('',*,*,#47712,.T.);
#66300=ORIENTED_EDGE('',*,*,#47713,.F.);
#66301=ORIENTED_EDGE('',*,*,#47767,.F.);
#66302=ORIENTED_EDGE('',*,*,#47411,.T.);
#66303=ORIENTED_EDGE('',*,*,#47766,.T.);
#66304=ORIENTED_EDGE('',*,*,#47604,.T.);
#66305=ORIENTED_EDGE('',*,*,#47711,.F.);
#66306=ORIENTED_EDGE('',*,*,#47768,.F.);
#66307=ORIENTED_EDGE('',*,*,#47414,.T.);
#66308=ORIENTED_EDGE('',*,*,#47599,.T.);
#66309=ORIENTED_EDGE('',*,*,#47416,.T.);
#66310=ORIENTED_EDGE('',*,*,#47769,.T.);
#66311=ORIENTED_EDGE('',*,*,#47709,.T.);
#66312=ORIENTED_EDGE('',*,*,#47710,.F.);
#66313=ORIENTED_EDGE('',*,*,#47769,.F.);
#66314=ORIENTED_EDGE('',*,*,#47415,.T.);
#66315=ORIENTED_EDGE('',*,*,#47768,.T.);
#66316=ORIENTED_EDGE('',*,*,#47603,.T.);
#66317=ORIENTED_EDGE('',*,*,#47705,.F.);
#66318=ORIENTED_EDGE('',*,*,#47770,.F.);
#66319=ORIENTED_EDGE('',*,*,#47422,.T.);
#66320=ORIENTED_EDGE('',*,*,#47587,.T.);
#66321=ORIENTED_EDGE('',*,*,#47424,.T.);
#66322=ORIENTED_EDGE('',*,*,#47771,.T.);
#66323=ORIENTED_EDGE('',*,*,#47703,.T.);
#66324=ORIENTED_EDGE('',*,*,#47704,.F.);
#66325=ORIENTED_EDGE('',*,*,#47771,.F.);
#66326=ORIENTED_EDGE('',*,*,#47423,.T.);
#66327=ORIENTED_EDGE('',*,*,#47770,.T.);
#66328=ORIENTED_EDGE('',*,*,#47598,.T.);
#66329=ORIENTED_EDGE('',*,*,#47708,.F.);
#66330=ORIENTED_EDGE('',*,*,#47772,.F.);
#66331=ORIENTED_EDGE('',*,*,#47418,.T.);
#66332=ORIENTED_EDGE('',*,*,#47601,.T.);
#66333=ORIENTED_EDGE('',*,*,#47420,.T.);
#66334=ORIENTED_EDGE('',*,*,#47773,.T.);
#66335=ORIENTED_EDGE('',*,*,#47706,.T.);
#66336=ORIENTED_EDGE('',*,*,#47707,.F.);
#66337=ORIENTED_EDGE('',*,*,#47773,.F.);
#66338=ORIENTED_EDGE('',*,*,#47419,.T.);
#66339=ORIENTED_EDGE('',*,*,#47772,.T.);
#66340=ORIENTED_EDGE('',*,*,#47594,.T.);
#66341=ORIENTED_EDGE('',*,*,#47690,.F.);
#66342=ORIENTED_EDGE('',*,*,#47774,.F.);
#66343=ORIENTED_EDGE('',*,*,#47442,.T.);
#66344=ORIENTED_EDGE('',*,*,#47595,.T.);
#66345=ORIENTED_EDGE('',*,*,#47444,.T.);
#66346=ORIENTED_EDGE('',*,*,#47775,.T.);
#66347=ORIENTED_EDGE('',*,*,#47688,.T.);
#66348=ORIENTED_EDGE('',*,*,#47689,.F.);
#66349=ORIENTED_EDGE('',*,*,#47775,.F.);
#66350=ORIENTED_EDGE('',*,*,#47443,.T.);
#66351=ORIENTED_EDGE('',*,*,#47774,.T.);
#66352=ORIENTED_EDGE('',*,*,#47591,.T.);
#66353=ORIENTED_EDGE('',*,*,#47693,.F.);
#66354=ORIENTED_EDGE('',*,*,#47776,.F.);
#66355=ORIENTED_EDGE('',*,*,#47438,.T.);
#66356=ORIENTED_EDGE('',*,*,#47592,.T.);
#66357=ORIENTED_EDGE('',*,*,#47440,.T.);
#66358=ORIENTED_EDGE('',*,*,#47777,.T.);
#66359=ORIENTED_EDGE('',*,*,#47691,.T.);
#66360=ORIENTED_EDGE('',*,*,#47692,.F.);
#66361=ORIENTED_EDGE('',*,*,#47777,.F.);
#66362=ORIENTED_EDGE('',*,*,#47439,.T.);
#66363=ORIENTED_EDGE('',*,*,#47776,.T.);
#66364=ORIENTED_EDGE('',*,*,#47585,.T.);
#66365=ORIENTED_EDGE('',*,*,#47696,.F.);
#66366=ORIENTED_EDGE('',*,*,#47778,.F.);
#66367=ORIENTED_EDGE('',*,*,#47434,.T.);
#66368=ORIENTED_EDGE('',*,*,#47589,.T.);
#66369=ORIENTED_EDGE('',*,*,#47436,.T.);
#66370=ORIENTED_EDGE('',*,*,#47779,.T.);
#66371=ORIENTED_EDGE('',*,*,#47694,.T.);
#66372=ORIENTED_EDGE('',*,*,#47695,.F.);
#66373=ORIENTED_EDGE('',*,*,#47779,.F.);
#66374=ORIENTED_EDGE('',*,*,#47435,.T.);
#66375=ORIENTED_EDGE('',*,*,#47778,.T.);
#66376=ORIENTED_EDGE('',*,*,#47586,.T.);
#66377=ORIENTED_EDGE('',*,*,#47702,.F.);
#66378=ORIENTED_EDGE('',*,*,#47780,.F.);
#66379=ORIENTED_EDGE('',*,*,#47426,.T.);
#66380=ORIENTED_EDGE('',*,*,#47581,.T.);
#66381=ORIENTED_EDGE('',*,*,#47428,.T.);
#66382=ORIENTED_EDGE('',*,*,#47781,.T.);
#66383=ORIENTED_EDGE('',*,*,#47700,.T.);
#66384=ORIENTED_EDGE('',*,*,#47701,.F.);
#66385=ORIENTED_EDGE('',*,*,#47781,.F.);
#66386=ORIENTED_EDGE('',*,*,#47427,.T.);
#66387=ORIENTED_EDGE('',*,*,#47780,.T.);
#66388=ORIENTED_EDGE('',*,*,#47580,.T.);
#66389=ORIENTED_EDGE('',*,*,#47699,.F.);
#66390=ORIENTED_EDGE('',*,*,#47782,.F.);
#66391=ORIENTED_EDGE('',*,*,#47430,.T.);
#66392=ORIENTED_EDGE('',*,*,#47583,.T.);
#66393=ORIENTED_EDGE('',*,*,#47432,.T.);
#66394=ORIENTED_EDGE('',*,*,#47783,.T.);
#66395=ORIENTED_EDGE('',*,*,#47697,.T.);
#66396=ORIENTED_EDGE('',*,*,#47698,.F.);
#66397=ORIENTED_EDGE('',*,*,#47783,.F.);
#66398=ORIENTED_EDGE('',*,*,#47431,.T.);
#66399=ORIENTED_EDGE('',*,*,#47782,.T.);
#66400=ORIENTED_EDGE('',*,*,#47535,.T.);
#66401=ORIENTED_EDGE('',*,*,#47739,.F.);
#66402=ORIENTED_EDGE('',*,*,#47784,.F.);
#66403=ORIENTED_EDGE('',*,*,#47376,.T.);
#66404=ORIENTED_EDGE('',*,*,#47578,.T.);
#66405=ORIENTED_EDGE('',*,*,#47378,.T.);
#66406=ORIENTED_EDGE('',*,*,#47785,.T.);
#66407=ORIENTED_EDGE('',*,*,#47737,.T.);
#66408=ORIENTED_EDGE('',*,*,#47738,.F.);
#66409=ORIENTED_EDGE('',*,*,#47785,.F.);
#66410=ORIENTED_EDGE('',*,*,#47377,.T.);
#66411=ORIENTED_EDGE('',*,*,#47784,.T.);
#66412=ORIENTED_EDGE('',*,*,#47577,.T.);
#66413=ORIENTED_EDGE('',*,*,#47736,.F.);
#66414=ORIENTED_EDGE('',*,*,#47786,.F.);
#66415=ORIENTED_EDGE('',*,*,#47380,.T.);
#66416=ORIENTED_EDGE('',*,*,#47572,.T.);
#66417=ORIENTED_EDGE('',*,*,#47382,.T.);
#66418=ORIENTED_EDGE('',*,*,#47787,.T.);
#66419=ORIENTED_EDGE('',*,*,#47734,.T.);
#66420=ORIENTED_EDGE('',*,*,#47735,.F.);
#66421=ORIENTED_EDGE('',*,*,#47787,.F.);
#66422=ORIENTED_EDGE('',*,*,#47381,.T.);
#66423=ORIENTED_EDGE('',*,*,#47786,.T.);
#66424=ORIENTED_EDGE('',*,*,#47576,.T.);
#66425=ORIENTED_EDGE('',*,*,#47730,.F.);
#66426=ORIENTED_EDGE('',*,*,#47788,.F.);
#66427=ORIENTED_EDGE('',*,*,#47388,.T.);
#66428=ORIENTED_EDGE('',*,*,#47562,.T.);
#66429=ORIENTED_EDGE('',*,*,#47390,.T.);
#66430=ORIENTED_EDGE('',*,*,#47789,.T.);
#66431=ORIENTED_EDGE('',*,*,#47728,.T.);
#66432=ORIENTED_EDGE('',*,*,#47729,.F.);
#66433=ORIENTED_EDGE('',*,*,#47789,.F.);
#66434=ORIENTED_EDGE('',*,*,#47389,.T.);
#66435=ORIENTED_EDGE('',*,*,#47788,.T.);
#66436=ORIENTED_EDGE('',*,*,#47571,.T.);
#66437=ORIENTED_EDGE('',*,*,#47733,.F.);
#66438=ORIENTED_EDGE('',*,*,#47790,.F.);
#66439=ORIENTED_EDGE('',*,*,#47384,.T.);
#66440=ORIENTED_EDGE('',*,*,#47574,.T.);
#66441=ORIENTED_EDGE('',*,*,#47386,.T.);
#66442=ORIENTED_EDGE('',*,*,#47791,.T.);
#66443=ORIENTED_EDGE('',*,*,#47731,.T.);
#66444=ORIENTED_EDGE('',*,*,#47732,.F.);
#66445=ORIENTED_EDGE('',*,*,#47791,.F.);
#66446=ORIENTED_EDGE('',*,*,#47385,.T.);
#66447=ORIENTED_EDGE('',*,*,#47790,.T.);
#66448=ORIENTED_EDGE('',*,*,#47567,.T.);
#66449=ORIENTED_EDGE('',*,*,#47717,.F.);
#66450=ORIENTED_EDGE('',*,*,#47792,.F.);
#66451=ORIENTED_EDGE('',*,*,#47406,.T.);
#66452=ORIENTED_EDGE('',*,*,#47568,.T.);
#66453=ORIENTED_EDGE('',*,*,#47408,.T.);
#66454=ORIENTED_EDGE('',*,*,#47793,.T.);
#66455=ORIENTED_EDGE('',*,*,#47715,.T.);
#66456=ORIENTED_EDGE('',*,*,#47716,.F.);
#66457=ORIENTED_EDGE('',*,*,#47793,.F.);
#66458=ORIENTED_EDGE('',*,*,#47407,.T.);
#66459=ORIENTED_EDGE('',*,*,#47792,.T.);
#66460=ORIENTED_EDGE('',*,*,#47565,.T.);
#66461=ORIENTED_EDGE('',*,*,#47719,.F.);
#66462=ORIENTED_EDGE('',*,*,#47794,.F.);
#66463=ORIENTED_EDGE('',*,*,#47403,.T.);
#66464=ORIENTED_EDGE('',*,*,#47718,.F.);
#66465=ORIENTED_EDGE('',*,*,#47368,.F.);
#66466=ORIENTED_EDGE('',*,*,#47404,.T.);
#66467=ORIENTED_EDGE('',*,*,#47794,.T.);
#66468=ORIENTED_EDGE('',*,*,#47560,.T.);
#66469=ORIENTED_EDGE('',*,*,#47721,.F.);
#66470=ORIENTED_EDGE('',*,*,#47795,.F.);
#66471=ORIENTED_EDGE('',*,*,#47400,.T.);
#66472=ORIENTED_EDGE('',*,*,#47720,.F.);
#66473=ORIENTED_EDGE('',*,*,#47364,.F.);
#66474=ORIENTED_EDGE('',*,*,#47401,.T.);
#66475=ORIENTED_EDGE('',*,*,#47795,.T.);
#66476=ORIENTED_EDGE('',*,*,#47561,.T.);
#66477=ORIENTED_EDGE('',*,*,#47727,.F.);
#66478=ORIENTED_EDGE('',*,*,#47796,.F.);
#66479=ORIENTED_EDGE('',*,*,#47392,.T.);
#66480=ORIENTED_EDGE('',*,*,#47556,.T.);
#66481=ORIENTED_EDGE('',*,*,#47394,.T.);
#66482=ORIENTED_EDGE('',*,*,#47797,.T.);
#66483=ORIENTED_EDGE('',*,*,#47725,.T.);
#66484=ORIENTED_EDGE('',*,*,#47726,.F.);
#66485=ORIENTED_EDGE('',*,*,#47797,.F.);
#66486=ORIENTED_EDGE('',*,*,#47393,.T.);
#66487=ORIENTED_EDGE('',*,*,#47796,.T.);
#66488=ORIENTED_EDGE('',*,*,#47555,.T.);
#66489=ORIENTED_EDGE('',*,*,#47724,.F.);
#66490=ORIENTED_EDGE('',*,*,#47798,.F.);
#66491=ORIENTED_EDGE('',*,*,#47396,.T.);
#66492=ORIENTED_EDGE('',*,*,#47558,.T.);
#66493=ORIENTED_EDGE('',*,*,#47398,.T.);
#66494=ORIENTED_EDGE('',*,*,#47799,.T.);
#66495=ORIENTED_EDGE('',*,*,#47722,.T.);
#66496=ORIENTED_EDGE('',*,*,#47723,.F.);
#66497=ORIENTED_EDGE('',*,*,#47799,.F.);
#66498=ORIENTED_EDGE('',*,*,#47397,.T.);
#66499=ORIENTED_EDGE('',*,*,#47798,.T.);
#66500=ORIENTED_EDGE('',*,*,#47551,.T.);
#66501=ORIENTED_EDGE('',*,*,#47649,.F.);
#66502=ORIENTED_EDGE('',*,*,#47800,.F.);
#66503=ORIENTED_EDGE('',*,*,#47496,.T.);
#66504=ORIENTED_EDGE('',*,*,#47553,.T.);
#66505=ORIENTED_EDGE('',*,*,#47498,.T.);
#66506=ORIENTED_EDGE('',*,*,#47801,.T.);
#66507=ORIENTED_EDGE('',*,*,#47647,.T.);
#66508=ORIENTED_EDGE('',*,*,#47648,.F.);
#66509=ORIENTED_EDGE('',*,*,#47801,.F.);
#66510=ORIENTED_EDGE('',*,*,#47497,.T.);
#66511=ORIENTED_EDGE('',*,*,#47800,.T.);
#66512=ORIENTED_EDGE('',*,*,#47552,.T.);
#66513=ORIENTED_EDGE('',*,*,#47646,.F.);
#66514=ORIENTED_EDGE('',*,*,#47802,.F.);
#66515=ORIENTED_EDGE('',*,*,#47500,.T.);
#66516=ORIENTED_EDGE('',*,*,#47543,.T.);
#66517=ORIENTED_EDGE('',*,*,#47502,.T.);
#66518=ORIENTED_EDGE('',*,*,#47803,.T.);
#66519=ORIENTED_EDGE('',*,*,#47644,.T.);
#66520=ORIENTED_EDGE('',*,*,#47645,.F.);
#66521=ORIENTED_EDGE('',*,*,#47803,.F.);
#66522=ORIENTED_EDGE('',*,*,#47501,.T.);
#66523=ORIENTED_EDGE('',*,*,#47802,.T.);
#66524=ORIENTED_EDGE('',*,*,#47549,.T.);
#66525=ORIENTED_EDGE('',*,*,#47494,.T.);
#66526=ORIENTED_EDGE('',*,*,#47804,.T.);
#66527=ORIENTED_EDGE('',*,*,#47650,.T.);
#66528=ORIENTED_EDGE('',*,*,#47651,.F.);
#66529=ORIENTED_EDGE('',*,*,#47804,.F.);
#66530=ORIENTED_EDGE('',*,*,#47493,.T.);
#66531=ORIENTED_EDGE('',*,*,#47362,.T.);
#66532=ORIENTED_EDGE('',*,*,#47547,.T.);
#66533=ORIENTED_EDGE('',*,*,#47491,.T.);
#66534=ORIENTED_EDGE('',*,*,#47805,.T.);
#66535=ORIENTED_EDGE('',*,*,#47652,.T.);
#66536=ORIENTED_EDGE('',*,*,#47653,.F.);
#66537=ORIENTED_EDGE('',*,*,#47805,.F.);
#66538=ORIENTED_EDGE('',*,*,#47490,.T.);
#66539=ORIENTED_EDGE('',*,*,#47358,.T.);
#66540=ORIENTED_EDGE('',*,*,#47542,.T.);
#66541=ORIENTED_EDGE('',*,*,#47643,.F.);
#66542=ORIENTED_EDGE('',*,*,#47806,.F.);
#66543=ORIENTED_EDGE('',*,*,#47504,.T.);
#66544=ORIENTED_EDGE('',*,*,#47540,.T.);
#66545=ORIENTED_EDGE('',*,*,#47506,.T.);
#66546=ORIENTED_EDGE('',*,*,#47807,.T.);
#66547=ORIENTED_EDGE('',*,*,#47641,.T.);
#66548=ORIENTED_EDGE('',*,*,#47642,.F.);
#66549=ORIENTED_EDGE('',*,*,#47807,.F.);
#66550=ORIENTED_EDGE('',*,*,#47505,.T.);
#66551=ORIENTED_EDGE('',*,*,#47806,.T.);
#66552=ORIENTED_EDGE('',*,*,#47539,.T.);
#66553=ORIENTED_EDGE('',*,*,#47640,.F.);
#66554=ORIENTED_EDGE('',*,*,#47808,.F.);
#66555=ORIENTED_EDGE('',*,*,#47508,.T.);
#66556=ORIENTED_EDGE('',*,*,#47537,.T.);
#66557=ORIENTED_EDGE('',*,*,#47510,.T.);
#66558=ORIENTED_EDGE('',*,*,#47809,.T.);
#66559=ORIENTED_EDGE('',*,*,#47638,.T.);
#66560=ORIENTED_EDGE('',*,*,#47639,.F.);
#66561=ORIENTED_EDGE('',*,*,#47809,.F.);
#66562=ORIENTED_EDGE('',*,*,#47509,.T.);
#66563=ORIENTED_EDGE('',*,*,#47808,.T.);
#66564=ORIENTED_EDGE('',*,*,#47536,.T.);
#66565=ORIENTED_EDGE('',*,*,#47637,.F.);
#66566=ORIENTED_EDGE('',*,*,#47810,.F.);
#66567=ORIENTED_EDGE('',*,*,#47512,.T.);
#66568=ORIENTED_EDGE('',*,*,#47531,.T.);
#66569=ORIENTED_EDGE('',*,*,#47514,.T.);
#66570=ORIENTED_EDGE('',*,*,#47811,.T.);
#66571=ORIENTED_EDGE('',*,*,#47635,.T.);
#66572=ORIENTED_EDGE('',*,*,#47636,.F.);
#66573=ORIENTED_EDGE('',*,*,#47811,.F.);
#66574=ORIENTED_EDGE('',*,*,#47513,.T.);
#66575=ORIENTED_EDGE('',*,*,#47810,.T.);
#66576=ORIENTED_EDGE('',*,*,#47530,.T.);
#66577=ORIENTED_EDGE('',*,*,#47634,.F.);
#66578=ORIENTED_EDGE('',*,*,#47812,.F.);
#66579=ORIENTED_EDGE('',*,*,#47372,.T.);
#66580=ORIENTED_EDGE('',*,*,#47533,.T.);
#66581=ORIENTED_EDGE('',*,*,#47374,.T.);
#66582=ORIENTED_EDGE('',*,*,#47813,.T.);
#66583=ORIENTED_EDGE('',*,*,#47740,.T.);
#66584=ORIENTED_EDGE('',*,*,#47741,.F.);
#66585=ORIENTED_EDGE('',*,*,#47813,.F.);
#66586=ORIENTED_EDGE('',*,*,#47373,.T.);
#66587=ORIENTED_EDGE('',*,*,#47812,.T.);
#66588=ORIENTED_EDGE('',*,*,#47317,.T.);
#66589=ORIENTED_EDGE('',*,*,#47316,.T.);
#66590=ORIENTED_EDGE('',*,*,#47337,.T.);
#66591=ORIENTED_EDGE('',*,*,#47333,.T.);
#66592=ORIENTED_EDGE('',*,*,#47349,.T.);
#66593=ORIENTED_EDGE('',*,*,#47312,.T.);
#66594=ORIENTED_EDGE('',*,*,#47814,.T.);
#66595=ORIENTED_EDGE('',*,*,#47815,.T.);
#66596=ORIENTED_EDGE('',*,*,#47348,.F.);
#66597=ORIENTED_EDGE('',*,*,#47816,.T.);
#66598=ORIENTED_EDGE('',*,*,#47817,.T.);
#66599=ORIENTED_EDGE('',*,*,#47818,.T.);
#66600=ORIENTED_EDGE('',*,*,#47814,.F.);
#66601=ORIENTED_EDGE('',*,*,#47819,.T.);
#66602=ORIENTED_EDGE('',*,*,#47820,.T.);
#66603=ORIENTED_EDGE('',*,*,#47821,.T.);
#66604=ORIENTED_EDGE('',*,*,#47817,.F.);
#66605=ORIENTED_EDGE('',*,*,#47822,.T.);
#66606=ORIENTED_EDGE('',*,*,#47823,.T.);
#66607=ORIENTED_EDGE('',*,*,#47824,.T.);
#66608=ORIENTED_EDGE('',*,*,#47820,.F.);
#66609=ORIENTED_EDGE('',*,*,#47825,.T.);
#66610=ORIENTED_EDGE('',*,*,#47826,.T.);
#66611=ORIENTED_EDGE('',*,*,#47827,.T.);
#66612=ORIENTED_EDGE('',*,*,#47823,.F.);
#66613=ORIENTED_EDGE('',*,*,#47828,.T.);
#66614=ORIENTED_EDGE('',*,*,#47829,.T.);
#66615=ORIENTED_EDGE('',*,*,#47325,.T.);
#66616=ORIENTED_EDGE('',*,*,#47826,.F.);
#66617=ORIENTED_EDGE('',*,*,#47830,.T.);
#66618=ORIENTED_EDGE('',*,*,#47346,.T.);
#66619=ORIENTED_EDGE('',*,*,#47831,.T.);
#66620=ORIENTED_EDGE('',*,*,#47829,.F.);
#66621=ORIENTED_EDGE('',*,*,#47832,.T.);
#66622=ORIENTED_EDGE('',*,*,#47816,.F.);
#66623=ORIENTED_EDGE('',*,*,#47347,.F.);
#66624=ORIENTED_EDGE('',*,*,#47832,.F.);
#66625=ORIENTED_EDGE('',*,*,#47830,.F.);
#66626=ORIENTED_EDGE('',*,*,#47828,.F.);
#66627=ORIENTED_EDGE('',*,*,#47825,.F.);
#66628=ORIENTED_EDGE('',*,*,#47822,.F.);
#66629=ORIENTED_EDGE('',*,*,#47819,.F.);
#66630=ORIENTED_EDGE('',*,*,#47833,.T.);
#66631=ORIENTED_EDGE('',*,*,#47834,.T.);
#66632=ORIENTED_EDGE('',*,*,#47835,.F.);
#66633=ORIENTED_EDGE('',*,*,#47836,.T.);
#66634=ORIENTED_EDGE('',*,*,#47342,.T.);
#66635=ORIENTED_EDGE('',*,*,#47837,.T.);
#66636=ORIENTED_EDGE('',*,*,#47833,.F.);
#66637=ORIENTED_EDGE('',*,*,#47838,.T.);
#66638=ORIENTED_EDGE('',*,*,#47839,.T.);
#66639=ORIENTED_EDGE('',*,*,#47840,.T.);
#66640=ORIENTED_EDGE('',*,*,#47344,.F.);
#66641=ORIENTED_EDGE('',*,*,#47841,.T.);
#66642=ORIENTED_EDGE('',*,*,#47842,.T.);
#66643=ORIENTED_EDGE('',*,*,#47321,.T.);
#66644=ORIENTED_EDGE('',*,*,#47839,.F.);
#66645=ORIENTED_EDGE('',*,*,#47843,.T.);
#66646=ORIENTED_EDGE('',*,*,#47844,.T.);
#66647=ORIENTED_EDGE('',*,*,#47845,.T.);
#66648=ORIENTED_EDGE('',*,*,#47842,.F.);
#66649=ORIENTED_EDGE('',*,*,#47846,.T.);
#66650=ORIENTED_EDGE('',*,*,#47847,.T.);
#66651=ORIENTED_EDGE('',*,*,#47848,.T.);
#66652=ORIENTED_EDGE('',*,*,#47844,.F.);
#66653=ORIENTED_EDGE('',*,*,#47849,.T.);
#66654=ORIENTED_EDGE('',*,*,#47835,.T.);
#66655=ORIENTED_EDGE('',*,*,#47850,.T.);
#66656=ORIENTED_EDGE('',*,*,#47847,.F.);
#66657=ORIENTED_EDGE('',*,*,#47851,.T.);
#66658=ORIENTED_EDGE('',*,*,#47836,.F.);
#66659=ORIENTED_EDGE('',*,*,#47851,.F.);
#66660=ORIENTED_EDGE('',*,*,#47849,.F.);
#66661=ORIENTED_EDGE('',*,*,#47846,.F.);
#66662=ORIENTED_EDGE('',*,*,#47843,.F.);
#66663=ORIENTED_EDGE('',*,*,#47841,.F.);
#66664=ORIENTED_EDGE('',*,*,#47343,.F.);
#66665=ORIENTED_EDGE('',*,*,#47838,.F.);
#66666=ORIENTED_EDGE('',*,*,#47852,.F.);
#66667=ORIENTED_EDGE('',*,*,#47345,.F.);
#66668=ORIENTED_EDGE('',*,*,#47853,.F.);
#66669=ORIENTED_EDGE('',*,*,#47520,.F.);
#66670=ORIENTED_EDGE('',*,*,#47853,.T.);
#66671=ORIENTED_EDGE('',*,*,#47815,.F.);
#66672=ORIENTED_EDGE('',*,*,#47854,.F.);
#66673=ORIENTED_EDGE('',*,*,#47521,.F.);
#66674=ORIENTED_EDGE('',*,*,#47852,.T.);
#66675=ORIENTED_EDGE('',*,*,#47519,.F.);
#66676=ORIENTED_EDGE('',*,*,#47326,.F.);
#66677=ORIENTED_EDGE('',*,*,#47831,.F.);
#66678=ORIENTED_EDGE('',*,*,#47854,.T.);
#66679=ORIENTED_EDGE('',*,*,#47818,.F.);
#66680=ORIENTED_EDGE('',*,*,#47855,.F.);
#66681=ORIENTED_EDGE('',*,*,#47522,.F.);
#66682=ORIENTED_EDGE('',*,*,#47855,.T.);
#66683=ORIENTED_EDGE('',*,*,#47821,.F.);
#66684=ORIENTED_EDGE('',*,*,#47856,.F.);
#66685=ORIENTED_EDGE('',*,*,#47516,.F.);
#66686=ORIENTED_EDGE('',*,*,#47328,.T.);
#66687=ORIENTED_EDGE('',*,*,#47518,.F.);
#66688=ORIENTED_EDGE('',*,*,#47857,.F.);
#66689=ORIENTED_EDGE('',*,*,#47827,.F.);
#66690=ORIENTED_EDGE('',*,*,#47856,.T.);
#66691=ORIENTED_EDGE('',*,*,#47824,.F.);
#66692=ORIENTED_EDGE('',*,*,#47857,.T.);
#66693=ORIENTED_EDGE('',*,*,#47517,.F.);
#66694=ORIENTED_EDGE('',*,*,#47858,.F.);
#66695=ORIENTED_EDGE('',*,*,#47848,.F.);
#66696=ORIENTED_EDGE('',*,*,#47859,.F.);
#66697=ORIENTED_EDGE('',*,*,#47527,.F.);
#66698=ORIENTED_EDGE('',*,*,#47859,.T.);
#66699=ORIENTED_EDGE('',*,*,#47850,.F.);
#66700=ORIENTED_EDGE('',*,*,#47860,.F.);
#66701=ORIENTED_EDGE('',*,*,#47528,.F.);
#66702=ORIENTED_EDGE('',*,*,#47858,.T.);
#66703=ORIENTED_EDGE('',*,*,#47526,.F.);
#66704=ORIENTED_EDGE('',*,*,#47322,.F.);
#66705=ORIENTED_EDGE('',*,*,#47845,.F.);
#66706=ORIENTED_EDGE('',*,*,#47860,.T.);
#66707=ORIENTED_EDGE('',*,*,#47834,.F.);
#66708=ORIENTED_EDGE('',*,*,#47861,.F.);
#66709=ORIENTED_EDGE('',*,*,#47529,.F.);
#66710=ORIENTED_EDGE('',*,*,#47861,.T.);
#66711=ORIENTED_EDGE('',*,*,#47837,.F.);
#66712=ORIENTED_EDGE('',*,*,#47862,.F.);
#66713=ORIENTED_EDGE('',*,*,#47523,.F.);
#66714=ORIENTED_EDGE('',*,*,#47324,.T.);
#66715=ORIENTED_EDGE('',*,*,#47525,.F.);
#66716=ORIENTED_EDGE('',*,*,#47863,.F.);
#66717=ORIENTED_EDGE('',*,*,#47840,.F.);
#66718=ORIENTED_EDGE('',*,*,#47862,.T.);
#66719=ORIENTED_EDGE('',*,*,#47341,.F.);
#66720=ORIENTED_EDGE('',*,*,#47863,.T.);
#66721=ORIENTED_EDGE('',*,*,#47524,.F.);
#66722=ORIENTED_EDGE('',*,*,#47301,.T.);
#66723=ORIENTED_EDGE('',*,*,#47298,.T.);
#87526=CYLINDRICAL_SURFACE('',#97483,1.5);
#87527=CYLINDRICAL_SURFACE('',#97484,1.5);
#87528=CYLINDRICAL_SURFACE('',#97487,9.);
#87529=CYLINDRICAL_SURFACE('',#97488,3.5);
#87530=CYLINDRICAL_SURFACE('',#97490,2.5);
#87531=CYLINDRICAL_SURFACE('',#97844,1.);
#87532=CYLINDRICAL_SURFACE('',#97847,1.);
#87533=CYLINDRICAL_SURFACE('',#97897,0.4);
#87534=CYLINDRICAL_SURFACE('',#97900,0.4);
#87535=CYLINDRICAL_SURFACE('',#97903,3.5);
#87536=CYLINDRICAL_SURFACE('',#97905,1.5);
#87537=CYLINDRICAL_SURFACE('',#97906,1.5);
#87538=CYLINDRICAL_SURFACE('',#97907,3.);
#87539=CYLINDRICAL_SURFACE('',#97909,3.7);
#87540=CYLINDRICAL_SURFACE('',#97912,3.7);
#87541=CYLINDRICAL_SURFACE('',#97915,3.7);
#87542=CYLINDRICAL_SURFACE('',#97918,3.7);
#87543=CYLINDRICAL_SURFACE('',#97921,1.5);
#87544=CYLINDRICAL_SURFACE('',#98077,9.75);
#87545=CYLINDRICAL_SURFACE('',#98079,9.75);
#87546=CYLINDRICAL_SURFACE('',#98081,9.75);
#87547=CYLINDRICAL_SURFACE('',#98083,9.75);
#87548=CYLINDRICAL_SURFACE('',#98085,9.75);
#87549=CYLINDRICAL_SURFACE('',#98087,9.75);
#87550=CYLINDRICAL_SURFACE('',#98089,9.75);
#87551=CYLINDRICAL_SURFACE('',#98091,9.75);
#87552=CYLINDRICAL_SURFACE('',#98093,9.75);
#87553=CYLINDRICAL_SURFACE('',#98095,9.75);
#87554=CYLINDRICAL_SURFACE('',#98097,9.75);
#87555=CYLINDRICAL_SURFACE('',#98099,9.75);
#87556=CYLINDRICAL_SURFACE('',#98101,9.75);
#87557=CYLINDRICAL_SURFACE('',#98103,9.75);
#87558=CYLINDRICAL_SURFACE('',#98105,9.75);
#87559=CYLINDRICAL_SURFACE('',#98107,9.75);
#87560=CYLINDRICAL_SURFACE('',#98109,9.75);
#87561=CYLINDRICAL_SURFACE('',#98111,9.75);
#87562=CYLINDRICAL_SURFACE('',#98113,9.75);
#87563=CYLINDRICAL_SURFACE('',#98115,9.75);
#87564=CYLINDRICAL_SURFACE('',#98117,9.75);
#87565=CYLINDRICAL_SURFACE('',#98119,9.75);
#87566=CYLINDRICAL_SURFACE('',#98121,9.75);
#87567=CYLINDRICAL_SURFACE('',#98123,9.75);
#87568=CYLINDRICAL_SURFACE('',#98125,9.75);
#87569=CYLINDRICAL_SURFACE('',#98127,9.75);
#87570=CYLINDRICAL_SURFACE('',#98129,9.75);
#87571=CYLINDRICAL_SURFACE('',#98131,9.75);
#87572=CYLINDRICAL_SURFACE('',#98133,9.75);
#87573=CYLINDRICAL_SURFACE('',#98135,9.75);
#87574=CYLINDRICAL_SURFACE('',#98137,9.75);
#87575=CYLINDRICAL_SURFACE('',#98139,9.75);
#87576=CYLINDRICAL_SURFACE('',#98141,9.75);
#87577=CYLINDRICAL_SURFACE('',#98143,9.75);
#87578=CYLINDRICAL_SURFACE('',#98145,9.75);
#87579=CYLINDRICAL_SURFACE('',#98147,9.75);
#87580=CYLINDRICAL_SURFACE('',#98258,9.75);
#87581=CYLINDRICAL_SURFACE('',#98259,3.7);
#87582=CYLINDRICAL_SURFACE('',#98260,3.7);
#87583=CYLINDRICAL_SURFACE('',#98261,8.624);
#87584=CYLINDRICAL_SURFACE('',#98262,3.7);
#87585=CYLINDRICAL_SURFACE('',#98263,3.7);
#87586=CYLINDRICAL_SURFACE('',#98264,8.624);
#87587=CYLINDRICAL_SURFACE('',#98265,3.7);
#87588=CYLINDRICAL_SURFACE('',#98266,3.7);
#87589=CYLINDRICAL_SURFACE('',#98267,8.624);
#87590=CYLINDRICAL_SURFACE('',#98268,3.7);
#87591=CYLINDRICAL_SURFACE('',#98269,3.7);
#87592=CYLINDRICAL_SURFACE('',#98270,8.624);
#87593=CYLINDRICAL_SURFACE('',#98271,3.7);
#87594=CYLINDRICAL_SURFACE('',#98272,3.7);
#87595=CYLINDRICAL_SURFACE('',#98273,8.624);
#87596=CYLINDRICAL_SURFACE('',#98274,3.7);
#87597=CYLINDRICAL_SURFACE('',#98275,3.7);
#87598=CYLINDRICAL_SURFACE('',#98276,8.624);
#87599=CYLINDRICAL_SURFACE('',#98277,3.7);
#87600=CYLINDRICAL_SURFACE('',#98278,3.7);
#87601=CYLINDRICAL_SURFACE('',#98279,8.624);
#87602=CYLINDRICAL_SURFACE('',#98280,3.7);
#87603=CYLINDRICAL_SURFACE('',#98281,3.7);
#87604=CYLINDRICAL_SURFACE('',#98282,8.624);
#87605=CYLINDRICAL_SURFACE('',#98283,3.7);
#87606=CYLINDRICAL_SURFACE('',#98284,3.7);
#87607=CYLINDRICAL_SURFACE('',#98285,8.624);
#87608=CYLINDRICAL_SURFACE('',#98286,3.7);
#87609=CYLINDRICAL_SURFACE('',#98287,3.7);
#87610=CYLINDRICAL_SURFACE('',#98288,8.624);
#87611=CYLINDRICAL_SURFACE('',#98289,3.7);
#87612=CYLINDRICAL_SURFACE('',#98290,3.7);
#87613=CYLINDRICAL_SURFACE('',#98291,8.624);
#87614=CYLINDRICAL_SURFACE('',#98292,3.7);
#87615=CYLINDRICAL_SURFACE('',#98293,3.7);
#87616=CYLINDRICAL_SURFACE('',#98294,8.624);
#87617=CYLINDRICAL_SURFACE('',#98295,3.7);
#87618=CYLINDRICAL_SURFACE('',#98296,3.7);
#87619=CYLINDRICAL_SURFACE('',#98297,8.624);
#87620=CYLINDRICAL_SURFACE('',#98298,3.7);
#87621=CYLINDRICAL_SURFACE('',#98299,3.7);
#87622=CYLINDRICAL_SURFACE('',#98300,8.624);
#87623=CYLINDRICAL_SURFACE('',#98301,3.7);
#87624=CYLINDRICAL_SURFACE('',#98302,3.7);
#87625=CYLINDRICAL_SURFACE('',#98303,8.624);
#87626=CYLINDRICAL_SURFACE('',#98304,3.7);
#87627=CYLINDRICAL_SURFACE('',#98305,3.7);
#87628=CYLINDRICAL_SURFACE('',#98306,8.624);
#87629=CYLINDRICAL_SURFACE('',#98307,3.7);
#87630=CYLINDRICAL_SURFACE('',#98308,3.7);
#87631=CYLINDRICAL_SURFACE('',#98309,8.624);
#87632=CYLINDRICAL_SURFACE('',#98310,3.7);
#87633=CYLINDRICAL_SURFACE('',#98311,3.7);
#87634=CYLINDRICAL_SURFACE('',#98312,8.624);
#87635=CYLINDRICAL_SURFACE('',#98313,3.7);
#87636=CYLINDRICAL_SURFACE('',#98314,3.7);
#87637=CYLINDRICAL_SURFACE('',#98315,8.624);
#87638=CYLINDRICAL_SURFACE('',#98316,3.7);
#87639=CYLINDRICAL_SURFACE('',#98317,3.7);
#87640=CYLINDRICAL_SURFACE('',#98318,8.624);
#87641=CYLINDRICAL_SURFACE('',#98319,3.7);
#87642=CYLINDRICAL_SURFACE('',#98320,3.7);
#87643=CYLINDRICAL_SURFACE('',#98321,8.624);
#87644=CYLINDRICAL_SURFACE('',#98322,3.7);
#87645=CYLINDRICAL_SURFACE('',#98323,3.7);
#87646=CYLINDRICAL_SURFACE('',#98324,8.624);
#87647=CYLINDRICAL_SURFACE('',#98325,3.7);
#87648=CYLINDRICAL_SURFACE('',#98326,3.7);
#87649=CYLINDRICAL_SURFACE('',#98327,8.624);
#87650=CYLINDRICAL_SURFACE('',#98328,3.7);
#87651=CYLINDRICAL_SURFACE('',#98329,3.7);
#87652=CYLINDRICAL_SURFACE('',#98330,8.624);
#87653=CYLINDRICAL_SURFACE('',#98331,3.7);
#87654=CYLINDRICAL_SURFACE('',#98332,3.7);
#87655=CYLINDRICAL_SURFACE('',#98333,8.624);
#87656=CYLINDRICAL_SURFACE('',#98334,3.7);
#87657=CYLINDRICAL_SURFACE('',#98335,8.624);
#87658=CYLINDRICAL_SURFACE('',#98336,3.7);
#87659=CYLINDRICAL_SURFACE('',#98337,8.624);
#87660=CYLINDRICAL_SURFACE('',#98338,3.7);
#87661=CYLINDRICAL_SURFACE('',#98339,3.7);
#87662=CYLINDRICAL_SURFACE('',#98340,8.624);
#87663=CYLINDRICAL_SURFACE('',#98341,3.7);
#87664=CYLINDRICAL_SURFACE('',#98342,3.7);
#87665=CYLINDRICAL_SURFACE('',#98343,8.624);
#87666=CYLINDRICAL_SURFACE('',#98344,3.7);
#87667=CYLINDRICAL_SURFACE('',#98345,3.7);
#87668=CYLINDRICAL_SURFACE('',#98346,8.624);
#87669=CYLINDRICAL_SURFACE('',#98347,3.7);
#87670=CYLINDRICAL_SURFACE('',#98348,3.7);
#87671=CYLINDRICAL_SURFACE('',#98349,8.624);
#87672=CYLINDRICAL_SURFACE('',#98350,3.7);
#87673=CYLINDRICAL_SURFACE('',#98351,8.624);
#87674=CYLINDRICAL_SURFACE('',#98352,3.7);
#87675=CYLINDRICAL_SURFACE('',#98353,8.624);
#87676=CYLINDRICAL_SURFACE('',#98354,3.7);
#87677=CYLINDRICAL_SURFACE('',#98355,3.7);
#87678=CYLINDRICAL_SURFACE('',#98356,8.624);
#87679=CYLINDRICAL_SURFACE('',#98357,3.7);
#87680=CYLINDRICAL_SURFACE('',#98358,3.7);
#87681=CYLINDRICAL_SURFACE('',#98359,8.624);
#87682=CYLINDRICAL_SURFACE('',#98360,3.7);
#87683=CYLINDRICAL_SURFACE('',#98361,3.7);
#87684=CYLINDRICAL_SURFACE('',#98362,8.624);
#87685=CYLINDRICAL_SURFACE('',#98363,3.7);
#87686=CYLINDRICAL_SURFACE('',#98364,3.7);
#87687=CYLINDRICAL_SURFACE('',#98365,8.624);
#87688=CYLINDRICAL_SURFACE('',#98371,0.4);
#87689=CYLINDRICAL_SURFACE('',#98374,5.);
#87690=CYLINDRICAL_SURFACE('',#98377,0.4);
#87691=CYLINDRICAL_SURFACE('',#98381,0.4);
#87692=CYLINDRICAL_SURFACE('',#98383,7.2);
#87693=CYLINDRICAL_SURFACE('',#98387,0.4);
#87694=CYLINDRICAL_SURFACE('',#98391,7.2);
#87695=CYLINDRICAL_SURFACE('',#98394,0.4);
#87696=CYLINDRICAL_SURFACE('',#98397,0.4);
#87697=CYLINDRICAL_SURFACE('',#98400,5.);
#87698=CYLINDRICAL_SURFACE('',#98407,0.2);
#87699=CYLINDRICAL_SURFACE('',#98414,0.2);
#87700=CYLINDRICAL_SURFACE('',#98422,0.2);
#87701=CYLINDRICAL_SURFACE('',#98425,0.2);
#89904=ADVANCED_FACE('',(#7440),#1698,.F.);
#89905=ADVANCED_FACE('',(#7441),#1699,.F.);
#89906=ADVANCED_FACE('',(#7442),#1700,.F.);
#89907=ADVANCED_FACE('',(#7443),#1701,.F.);
#89908=ADVANCED_FACE('',(#7444),#1702,.F.);
#89909=ADVANCED_FACE('',(#7445),#1703,.F.);
#89910=ADVANCED_FACE('',(#7446),#1704,.F.);
#89911=ADVANCED_FACE('',(#7447),#1705,.F.);
#89912=ADVANCED_FACE('',(#7448),#1706,.F.);
#89913=ADVANCED_FACE('',(#7449),#1707,.F.);
#89914=ADVANCED_FACE('',(#7450),#1708,.F.);
#89915=ADVANCED_FACE('',(#7451),#1709,.F.);
#89916=ADVANCED_FACE('',(#7452),#1710,.F.);
#89917=ADVANCED_FACE('',(#7453),#1711,.F.);
#89918=ADVANCED_FACE('',(#7454),#1712,.F.);
#89919=ADVANCED_FACE('',(#7455),#1713,.F.);
#89920=ADVANCED_FACE('',(#7456),#1714,.F.);
#89921=ADVANCED_FACE('',(#7457),#1715,.F.);
#89922=ADVANCED_FACE('',(#7458),#1716,.F.);
#89923=ADVANCED_FACE('',(#7459),#1717,.F.);
#89924=ADVANCED_FACE('',(#7460),#1718,.F.);
#89925=ADVANCED_FACE('',(#7461),#1719,.F.);
#89926=ADVANCED_FACE('',(#7462),#1720,.F.);
#89927=ADVANCED_FACE('',(#7463),#1721,.F.);
#89928=ADVANCED_FACE('',(#7464),#1722,.F.);
#89929=ADVANCED_FACE('',(#7465),#1723,.F.);
#89930=ADVANCED_FACE('',(#7466),#1724,.F.);
#89931=ADVANCED_FACE('',(#7467),#1725,.F.);
#89932=ADVANCED_FACE('',(#7468),#1726,.F.);
#89933=ADVANCED_FACE('',(#7469),#1727,.F.);
#89934=ADVANCED_FACE('',(#7470),#1728,.F.);
#89935=ADVANCED_FACE('',(#7471),#1729,.F.);
#89936=ADVANCED_FACE('',(#7472),#1730,.F.);
#89937=ADVANCED_FACE('',(#7473),#1731,.F.);
#89938=ADVANCED_FACE('',(#7474),#1732,.F.);
#89939=ADVANCED_FACE('',(#7475),#1733,.F.);
#89940=ADVANCED_FACE('',(#7476),#1734,.F.);
#89941=ADVANCED_FACE('',(#7477),#1735,.F.);
#89942=ADVANCED_FACE('',(#7478),#1736,.F.);
#89943=ADVANCED_FACE('',(#7479),#1737,.F.);
#89944=ADVANCED_FACE('',(#7480),#1738,.F.);
#89945=ADVANCED_FACE('',(#7481),#1739,.F.);
#89946=ADVANCED_FACE('',(#7482),#1740,.F.);
#89947=ADVANCED_FACE('',(#7483),#1741,.F.);
#89948=ADVANCED_FACE('',(#7484),#1742,.F.);
#89949=ADVANCED_FACE('',(#7485),#1743,.F.);
#89950=ADVANCED_FACE('',(#7486),#1744,.F.);
#89951=ADVANCED_FACE('',(#7487),#1745,.F.);
#89952=ADVANCED_FACE('',(#7488),#1746,.F.);
#89953=ADVANCED_FACE('',(#7489),#1747,.F.);
#89954=ADVANCED_FACE('',(#7490),#1748,.F.);
#89955=ADVANCED_FACE('',(#7491),#1749,.F.);
#89956=ADVANCED_FACE('',(#7492),#1750,.F.);
#89957=ADVANCED_FACE('',(#7493),#1751,.F.);
#89958=ADVANCED_FACE('',(#7494),#1752,.F.);
#89959=ADVANCED_FACE('',(#7495),#1753,.F.);
#89960=ADVANCED_FACE('',(#7496),#1754,.F.);
#89961=ADVANCED_FACE('',(#7497),#1755,.F.);
#89962=ADVANCED_FACE('',(#7498),#1756,.F.);
#89963=ADVANCED_FACE('',(#7499),#1757,.F.);
#89964=ADVANCED_FACE('',(#7500),#1758,.F.);
#89965=ADVANCED_FACE('',(#7501),#1759,.F.);
#89966=ADVANCED_FACE('',(#7502),#1760,.F.);
#89967=ADVANCED_FACE('',(#7503),#1761,.F.);
#89968=ADVANCED_FACE('',(#7504),#1762,.F.);
#89969=ADVANCED_FACE('',(#7505),#1763,.F.);
#89970=ADVANCED_FACE('',(#7506),#1764,.F.);
#89971=ADVANCED_FACE('',(#7507),#1765,.F.);
#89972=ADVANCED_FACE('',(#7508),#1766,.F.);
#89973=ADVANCED_FACE('',(#7509),#1767,.F.);
#89974=ADVANCED_FACE('',(#7510),#4712,.F.);
#89975=ADVANCED_FACE('',(#7511),#4713,.F.);
#89976=ADVANCED_FACE('',(#7512),#4714,.F.);
#89977=ADVANCED_FACE('',(#7513),#4715,.T.);
#89978=ADVANCED_FACE('',(#7514),#4716,.F.);
#89979=ADVANCED_FACE('',(#7515),#4717,.F.);
#89980=ADVANCED_FACE('',(#7516),#4718,.T.);
#89981=ADVANCED_FACE('',(#7517),#4719,.F.);
#89982=ADVANCED_FACE('',(#7518),#87526,.F.);
#89983=ADVANCED_FACE('',(#7519),#87527,.F.);
#89984=ADVANCED_FACE('',(#7520),#4720,.T.);
#89985=ADVANCED_FACE('',(#7521),#87528,.T.);
#89986=ADVANCED_FACE('',(#7522),#87529,.T.);
#89987=ADVANCED_FACE('',(#7523),#87530,.F.);
#89988=ADVANCED_FACE('',(#7524,#5170),#5591,.T.);
#89989=ADVANCED_FACE('',(#7525,#5171,#5172,#5173),#5592,.T.);
#89990=ADVANCED_FACE('',(#7526,#5174,#5175,#5176),#5593,.T.);
#89991=ADVANCED_FACE('',(#7527),#4721,.F.);
#89992=ADVANCED_FACE('',(#7528),#1768,.F.);
#89993=ADVANCED_FACE('',(#7529),#4722,.F.);
#89994=ADVANCED_FACE('',(#7530),#4723,.F.);
#89995=ADVANCED_FACE('',(#7531),#1769,.F.);
#89996=ADVANCED_FACE('',(#7532),#4724,.F.);
#89997=ADVANCED_FACE('',(#7533),#4725,.F.);
#89998=ADVANCED_FACE('',(#7534),#1770,.F.);
#89999=ADVANCED_FACE('',(#7535),#4726,.F.);
#90000=ADVANCED_FACE('',(#7536),#4727,.F.);
#90001=ADVANCED_FACE('',(#7537),#1771,.F.);
#90002=ADVANCED_FACE('',(#7538),#4728,.F.);
#90003=ADVANCED_FACE('',(#7539),#4729,.F.);
#90004=ADVANCED_FACE('',(#7540),#1772,.F.);
#90005=ADVANCED_FACE('',(#7541),#4730,.F.);
#90006=ADVANCED_FACE('',(#7542),#4731,.F.);
#90007=ADVANCED_FACE('',(#7543),#1773,.F.);
#90008=ADVANCED_FACE('',(#7544),#4732,.F.);
#90009=ADVANCED_FACE('',(#7545),#4733,.F.);
#90010=ADVANCED_FACE('',(#7546),#1774,.F.);
#90011=ADVANCED_FACE('',(#7547),#4734,.F.);
#90012=ADVANCED_FACE('',(#7548),#4735,.F.);
#90013=ADVANCED_FACE('',(#7549),#1775,.F.);
#90014=ADVANCED_FACE('',(#7550),#4736,.F.);
#90015=ADVANCED_FACE('',(#7551),#4737,.F.);
#90016=ADVANCED_FACE('',(#7552),#1776,.F.);
#90017=ADVANCED_FACE('',(#7553),#4738,.F.);
#90018=ADVANCED_FACE('',(#7554),#4739,.F.);
#90019=ADVANCED_FACE('',(#7555),#1777,.F.);
#90020=ADVANCED_FACE('',(#7556),#4740,.F.);
#90021=ADVANCED_FACE('',(#7557),#4741,.F.);
#90022=ADVANCED_FACE('',(#7558),#1778,.F.);
#90023=ADVANCED_FACE('',(#7559),#4742,.F.);
#90024=ADVANCED_FACE('',(#7560),#4743,.F.);
#90025=ADVANCED_FACE('',(#7561),#1779,.F.);
#90026=ADVANCED_FACE('',(#7562),#4744,.F.);
#90027=ADVANCED_FACE('',(#7563),#4745,.F.);
#90028=ADVANCED_FACE('',(#7564),#1780,.F.);
#90029=ADVANCED_FACE('',(#7565),#4746,.F.);
#90030=ADVANCED_FACE('',(#7566),#4747,.F.);
#90031=ADVANCED_FACE('',(#7567),#1781,.F.);
#90032=ADVANCED_FACE('',(#7568),#4748,.F.);
#90033=ADVANCED_FACE('',(#7569),#4749,.F.);
#90034=ADVANCED_FACE('',(#7570),#1782,.F.);
#90035=ADVANCED_FACE('',(#7571),#4750,.F.);
#90036=ADVANCED_FACE('',(#7572),#4751,.F.);
#90037=ADVANCED_FACE('',(#7573),#1783,.F.);
#90038=ADVANCED_FACE('',(#7574),#4752,.F.);
#90039=ADVANCED_FACE('',(#7575),#4753,.F.);
#90040=ADVANCED_FACE('',(#7576),#1784,.F.);
#90041=ADVANCED_FACE('',(#7577),#4754,.F.);
#90042=ADVANCED_FACE('',(#7578),#4755,.F.);
#90043=ADVANCED_FACE('',(#7579),#1785,.F.);
#90044=ADVANCED_FACE('',(#7580),#4756,.F.);
#90045=ADVANCED_FACE('',(#7581),#4757,.F.);
#90046=ADVANCED_FACE('',(#7582),#1786,.F.);
#90047=ADVANCED_FACE('',(#7583),#4758,.F.);
#90048=ADVANCED_FACE('',(#7584),#4759,.F.);
#90049=ADVANCED_FACE('',(#7585),#1787,.F.);
#90050=ADVANCED_FACE('',(#7586),#4760,.F.);
#90051=ADVANCED_FACE('',(#7587),#4761,.F.);
#90052=ADVANCED_FACE('',(#7588),#1788,.F.);
#90053=ADVANCED_FACE('',(#7589),#4762,.F.);
#90054=ADVANCED_FACE('',(#7590),#4763,.F.);
#90055=ADVANCED_FACE('',(#7591),#1789,.F.);
#90056=ADVANCED_FACE('',(#7592),#4764,.F.);
#90057=ADVANCED_FACE('',(#7593),#4765,.F.);
#90058=ADVANCED_FACE('',(#7594),#1790,.F.);
#90059=ADVANCED_FACE('',(#7595),#4766,.F.);
#90060=ADVANCED_FACE('',(#7596),#4767,.F.);
#90061=ADVANCED_FACE('',(#7597),#1791,.F.);
#90062=ADVANCED_FACE('',(#7598),#4768,.F.);
#90063=ADVANCED_FACE('',(#7599),#4769,.F.);
#90064=ADVANCED_FACE('',(#7600),#1792,.F.);
#90065=ADVANCED_FACE('',(#7601),#4770,.F.);
#90066=ADVANCED_FACE('',(#7602),#4771,.F.);
#90067=ADVANCED_FACE('',(#7603),#1793,.F.);
#90068=ADVANCED_FACE('',(#7604),#4772,.F.);
#90069=ADVANCED_FACE('',(#7605),#4773,.F.);
#90070=ADVANCED_FACE('',(#7606),#1794,.F.);
#90071=ADVANCED_FACE('',(#7607),#4774,.F.);
#90072=ADVANCED_FACE('',(#7608),#4775,.F.);
#90073=ADVANCED_FACE('',(#7609),#1795,.F.);
#90074=ADVANCED_FACE('',(#7610),#4776,.F.);
#90075=ADVANCED_FACE('',(#7611),#4777,.F.);
#90076=ADVANCED_FACE('',(#7612),#1796,.F.);
#90077=ADVANCED_FACE('',(#7613),#4778,.F.);
#90078=ADVANCED_FACE('',(#7614),#4779,.F.);
#90079=ADVANCED_FACE('',(#7615),#1797,.F.);
#90080=ADVANCED_FACE('',(#7616),#4780,.F.);
#90081=ADVANCED_FACE('',(#7617),#4781,.F.);
#90082=ADVANCED_FACE('',(#7618),#1798,.F.);
#90083=ADVANCED_FACE('',(#7619),#4782,.F.);
#90084=ADVANCED_FACE('',(#7620),#4783,.F.);
#90085=ADVANCED_FACE('',(#7621),#1799,.F.);
#90086=ADVANCED_FACE('',(#7622),#4784,.F.);
#90087=ADVANCED_FACE('',(#7623),#4785,.F.);
#90088=ADVANCED_FACE('',(#7624),#1800,.F.);
#90089=ADVANCED_FACE('',(#7625),#4786,.F.);
#90090=ADVANCED_FACE('',(#7626),#4787,.F.);
#90091=ADVANCED_FACE('',(#7627),#1801,.F.);
#90092=ADVANCED_FACE('',(#7628),#4788,.F.);
#90093=ADVANCED_FACE('',(#7629),#4789,.F.);
#90094=ADVANCED_FACE('',(#7630),#1802,.F.);
#90095=ADVANCED_FACE('',(#7631),#4790,.F.);
#90096=ADVANCED_FACE('',(#7632),#4791,.F.);
#90097=ADVANCED_FACE('',(#7633),#1803,.F.);
#90098=ADVANCED_FACE('',(#7634),#4792,.F.);
#90099=ADVANCED_FACE('',(#7635),#4793,.F.);
#90100=ADVANCED_FACE('',(#7636),#1804,.F.);
#90101=ADVANCED_FACE('',(#7637),#4794,.F.);
#90102=ADVANCED_FACE('',(#7638),#4795,.F.);
#90103=ADVANCED_FACE('',(#7639),#1805,.F.);
#90104=ADVANCED_FACE('',(#7640),#4796,.F.);
#90105=ADVANCED_FACE('',(#7641),#4797,.F.);
#90106=ADVANCED_FACE('',(#7642),#1806,.F.);
#90107=ADVANCED_FACE('',(#7643),#4798,.F.);
#90108=ADVANCED_FACE('',(#7644),#4799,.F.);
#90109=ADVANCED_FACE('',(#7645),#1807,.F.);
#90110=ADVANCED_FACE('',(#7646),#4800,.F.);
#90111=ADVANCED_FACE('',(#7647),#4801,.F.);
#90112=ADVANCED_FACE('',(#7648),#1808,.F.);
#90113=ADVANCED_FACE('',(#7649),#4802,.F.);
#90114=ADVANCED_FACE('',(#7650),#4803,.F.);
#90115=ADVANCED_FACE('',(#7651),#1809,.F.);
#90116=ADVANCED_FACE('',(#7652),#4804,.F.);
#90117=ADVANCED_FACE('',(#7653),#4805,.F.);
#90118=ADVANCED_FACE('',(#7654),#1810,.F.);
#90119=ADVANCED_FACE('',(#7655),#4806,.F.);
#90120=ADVANCED_FACE('',(#7656),#4807,.F.);
#90121=ADVANCED_FACE('',(#7657),#1811,.F.);
#90122=ADVANCED_FACE('',(#7658),#4808,.F.);
#90123=ADVANCED_FACE('',(#7659),#4809,.F.);
#90124=ADVANCED_FACE('',(#7660),#1812,.F.);
#90125=ADVANCED_FACE('',(#7661),#4810,.F.);
#90126=ADVANCED_FACE('',(#7662),#4811,.F.);
#90127=ADVANCED_FACE('',(#7663),#1813,.F.);
#90128=ADVANCED_FACE('',(#7664),#4812,.F.);
#90129=ADVANCED_FACE('',(#7665),#4813,.F.);
#90130=ADVANCED_FACE('',(#7666),#1814,.F.);
#90131=ADVANCED_FACE('',(#7667),#4814,.F.);
#90132=ADVANCED_FACE('',(#7668),#4815,.F.);
#90133=ADVANCED_FACE('',(#7669),#1815,.F.);
#90134=ADVANCED_FACE('',(#7670),#4816,.F.);
#90135=ADVANCED_FACE('',(#7671),#4817,.F.);
#90136=ADVANCED_FACE('',(#7672),#1816,.F.);
#90137=ADVANCED_FACE('',(#7673),#4818,.F.);
#90138=ADVANCED_FACE('',(#7674),#4819,.F.);
#90139=ADVANCED_FACE('',(#7675),#1817,.F.);
#90140=ADVANCED_FACE('',(#7676),#4820,.F.);
#90141=ADVANCED_FACE('',(#7677),#4821,.F.);
#90142=ADVANCED_FACE('',(#7678),#1818,.F.);
#90143=ADVANCED_FACE('',(#7679),#4822,.F.);
#90144=ADVANCED_FACE('',(#7680),#4823,.F.);
#90145=ADVANCED_FACE('',(#7681),#1819,.F.);
#90146=ADVANCED_FACE('',(#7682),#4824,.F.);
#90147=ADVANCED_FACE('',(#7683),#4825,.F.);
#90148=ADVANCED_FACE('',(#7684),#1820,.F.);
#90149=ADVANCED_FACE('',(#7685),#4826,.F.);
#90150=ADVANCED_FACE('',(#7686),#4827,.F.);
#90151=ADVANCED_FACE('',(#7687),#1821,.F.);
#90152=ADVANCED_FACE('',(#7688),#4828,.F.);
#90153=ADVANCED_FACE('',(#7689),#4829,.F.);
#90154=ADVANCED_FACE('',(#7690),#1822,.F.);
#90155=ADVANCED_FACE('',(#7691),#4830,.F.);
#90156=ADVANCED_FACE('',(#7692),#4831,.F.);
#90157=ADVANCED_FACE('',(#7693),#1823,.F.);
#90158=ADVANCED_FACE('',(#7694),#4832,.F.);
#90159=ADVANCED_FACE('',(#7695),#4833,.F.);
#90160=ADVANCED_FACE('',(#7696),#1824,.F.);
#90161=ADVANCED_FACE('',(#7697),#4834,.F.);
#90162=ADVANCED_FACE('',(#7698),#4835,.F.);
#90163=ADVANCED_FACE('',(#7699),#1825,.F.);
#90164=ADVANCED_FACE('',(#7700),#4836,.F.);
#90165=ADVANCED_FACE('',(#7701),#4837,.F.);
#90166=ADVANCED_FACE('',(#7702),#1826,.F.);
#90167=ADVANCED_FACE('',(#7703),#4838,.F.);
#90168=ADVANCED_FACE('',(#7704),#4839,.F.);
#90169=ADVANCED_FACE('',(#7705),#1827,.F.);
#90170=ADVANCED_FACE('',(#7706),#4840,.F.);
#90171=ADVANCED_FACE('',(#7707),#4841,.F.);
#90172=ADVANCED_FACE('',(#7708),#1828,.F.);
#90173=ADVANCED_FACE('',(#7709),#4842,.F.);
#90174=ADVANCED_FACE('',(#7710),#4843,.F.);
#90175=ADVANCED_FACE('',(#7711),#1829,.F.);
#90176=ADVANCED_FACE('',(#7712),#4844,.F.);
#90177=ADVANCED_FACE('',(#7713),#4845,.F.);
#90178=ADVANCED_FACE('',(#7714),#1830,.F.);
#90179=ADVANCED_FACE('',(#7715),#4846,.F.);
#90180=ADVANCED_FACE('',(#7716),#4847,.F.);
#90181=ADVANCED_FACE('',(#7717),#1831,.F.);
#90182=ADVANCED_FACE('',(#7718),#4848,.F.);
#90183=ADVANCED_FACE('',(#7719),#4849,.F.);
#90184=ADVANCED_FACE('',(#7720),#1832,.F.);
#90185=ADVANCED_FACE('',(#7721),#4850,.F.);
#90186=ADVANCED_FACE('',(#7722),#4851,.F.);
#90187=ADVANCED_FACE('',(#7723),#1833,.F.);
#90188=ADVANCED_FACE('',(#7724),#4852,.F.);
#90189=ADVANCED_FACE('',(#7725),#4853,.F.);
#90190=ADVANCED_FACE('',(#7726),#1834,.F.);
#90191=ADVANCED_FACE('',(#7727),#4854,.F.);
#90192=ADVANCED_FACE('',(#7728),#4855,.F.);
#90193=ADVANCED_FACE('',(#7729),#1835,.F.);
#90194=ADVANCED_FACE('',(#7730),#4856,.F.);
#90195=ADVANCED_FACE('',(#7731),#4857,.F.);
#90196=ADVANCED_FACE('',(#7732),#1836,.F.);
#90197=ADVANCED_FACE('',(#7733),#4858,.F.);
#90198=ADVANCED_FACE('',(#7734),#4859,.F.);
#90199=ADVANCED_FACE('',(#7735),#1837,.F.);
#90200=ADVANCED_FACE('',(#7736),#4860,.F.);
#90201=ADVANCED_FACE('',(#7737),#87531,.F.);
#90202=ADVANCED_FACE('',(#7738),#87532,.F.);
#90203=ADVANCED_FACE('',(#7739),#1838,.F.);
#90204=ADVANCED_FACE('',(#7740),#1839,.F.);
#90205=ADVANCED_FACE('',(#7741),#1840,.T.);
#90206=ADVANCED_FACE('',(#7742),#1841,.T.);
#90207=ADVANCED_FACE('',(#7743),#1842,.T.);
#90208=ADVANCED_FACE('',(#7744),#1843,.T.);
#90209=ADVANCED_FACE('',(#7745),#1844,.T.);
#90210=ADVANCED_FACE('',(#7746),#1845,.T.);
#90211=ADVANCED_FACE('',(#7747),#1846,.T.);
#90212=ADVANCED_FACE('',(#7748),#1847,.T.);
#90213=ADVANCED_FACE('',(#7749),#87533,.F.);
#90214=ADVANCED_FACE('',(#7750),#87534,.F.);
#90215=ADVANCED_FACE('',(#7751),#87535,.F.);
#90216=ADVANCED_FACE('',(#7752),#87536,.T.);
#90217=ADVANCED_FACE('',(#7753),#87537,.T.);
#90218=ADVANCED_FACE('',(#7754),#87538,.T.);
#90219=ADVANCED_FACE('',(#7755),#87539,.T.);
#90220=ADVANCED_FACE('',(#7756),#87540,.T.);
#90221=ADVANCED_FACE('',(#7757),#87541,.T.);
#90222=ADVANCED_FACE('',(#7758),#87542,.T.);
#90223=ADVANCED_FACE('',(#7759),#87543,.F.);
#90224=ADVANCED_FACE('',(#7760,#5177,#5178,#5179,#5180,#5181),#5594,.F.);
#90225=ADVANCED_FACE('',(#7761),#87544,.T.);
#90226=ADVANCED_FACE('',(#7762),#87545,.T.);
#90227=ADVANCED_FACE('',(#7763),#87546,.T.);
#90228=ADVANCED_FACE('',(#7764),#87547,.T.);
#90229=ADVANCED_FACE('',(#7765),#87548,.T.);
#90230=ADVANCED_FACE('',(#7766),#87549,.T.);
#90231=ADVANCED_FACE('',(#7767),#87550,.T.);
#90232=ADVANCED_FACE('',(#7768),#87551,.T.);
#90233=ADVANCED_FACE('',(#7769),#87552,.T.);
#90234=ADVANCED_FACE('',(#7770),#87553,.T.);
#90235=ADVANCED_FACE('',(#7771),#87554,.T.);
#90236=ADVANCED_FACE('',(#7772),#87555,.T.);
#90237=ADVANCED_FACE('',(#7773),#87556,.T.);
#90238=ADVANCED_FACE('',(#7774),#87557,.T.);
#90239=ADVANCED_FACE('',(#7775),#87558,.T.);
#90240=ADVANCED_FACE('',(#7776),#87559,.T.);
#90241=ADVANCED_FACE('',(#7777),#87560,.T.);
#90242=ADVANCED_FACE('',(#7778),#87561,.T.);
#90243=ADVANCED_FACE('',(#7779),#87562,.T.);
#90244=ADVANCED_FACE('',(#7780),#87563,.T.);
#90245=ADVANCED_FACE('',(#7781),#87564,.T.);
#90246=ADVANCED_FACE('',(#7782),#87565,.T.);
#90247=ADVANCED_FACE('',(#7783),#87566,.T.);
#90248=ADVANCED_FACE('',(#7784),#87567,.T.);
#90249=ADVANCED_FACE('',(#7785),#87568,.T.);
#90250=ADVANCED_FACE('',(#7786),#87569,.T.);
#90251=ADVANCED_FACE('',(#7787),#87570,.T.);
#90252=ADVANCED_FACE('',(#7788),#87571,.T.);
#90253=ADVANCED_FACE('',(#7789),#87572,.T.);
#90254=ADVANCED_FACE('',(#7790),#87573,.T.);
#90255=ADVANCED_FACE('',(#7791),#87574,.T.);
#90256=ADVANCED_FACE('',(#7792),#87575,.T.);
#90257=ADVANCED_FACE('',(#7793),#87576,.T.);
#90258=ADVANCED_FACE('',(#7794),#87577,.T.);
#90259=ADVANCED_FACE('',(#7795),#87578,.T.);
#90260=ADVANCED_FACE('',(#7796),#87579,.T.);
#90261=ADVANCED_FACE('',(#7797,#5182,#5183,#5184),#5595,.F.);
#90262=ADVANCED_FACE('',(#7798),#87580,.T.);
#90263=ADVANCED_FACE('',(#7799),#87581,.T.);
#90264=ADVANCED_FACE('',(#7800),#87582,.T.);
#90265=ADVANCED_FACE('',(#7801),#87583,.T.);
#90266=ADVANCED_FACE('',(#7802),#87584,.T.);
#90267=ADVANCED_FACE('',(#7803),#87585,.T.);
#90268=ADVANCED_FACE('',(#7804),#87586,.T.);
#90269=ADVANCED_FACE('',(#7805),#87587,.T.);
#90270=ADVANCED_FACE('',(#7806),#87588,.T.);
#90271=ADVANCED_FACE('',(#7807),#87589,.T.);
#90272=ADVANCED_FACE('',(#7808),#87590,.T.);
#90273=ADVANCED_FACE('',(#7809),#87591,.T.);
#90274=ADVANCED_FACE('',(#7810),#87592,.T.);
#90275=ADVANCED_FACE('',(#7811),#87593,.T.);
#90276=ADVANCED_FACE('',(#7812),#87594,.T.);
#90277=ADVANCED_FACE('',(#7813),#87595,.T.);
#90278=ADVANCED_FACE('',(#7814),#87596,.T.);
#90279=ADVANCED_FACE('',(#7815),#87597,.T.);
#90280=ADVANCED_FACE('',(#7816),#87598,.T.);
#90281=ADVANCED_FACE('',(#7817),#87599,.T.);
#90282=ADVANCED_FACE('',(#7818),#87600,.T.);
#90283=ADVANCED_FACE('',(#7819),#87601,.T.);
#90284=ADVANCED_FACE('',(#7820),#87602,.T.);
#90285=ADVANCED_FACE('',(#7821),#87603,.T.);
#90286=ADVANCED_FACE('',(#7822),#87604,.T.);
#90287=ADVANCED_FACE('',(#7823),#87605,.T.);
#90288=ADVANCED_FACE('',(#7824),#87606,.T.);
#90289=ADVANCED_FACE('',(#7825),#87607,.T.);
#90290=ADVANCED_FACE('',(#7826),#87608,.T.);
#90291=ADVANCED_FACE('',(#7827),#87609,.T.);
#90292=ADVANCED_FACE('',(#7828),#87610,.T.);
#90293=ADVANCED_FACE('',(#7829),#87611,.T.);
#90294=ADVANCED_FACE('',(#7830),#87612,.T.);
#90295=ADVANCED_FACE('',(#7831),#87613,.T.);
#90296=ADVANCED_FACE('',(#7832),#87614,.T.);
#90297=ADVANCED_FACE('',(#7833),#87615,.T.);
#90298=ADVANCED_FACE('',(#7834),#87616,.T.);
#90299=ADVANCED_FACE('',(#7835),#87617,.T.);
#90300=ADVANCED_FACE('',(#7836),#87618,.T.);
#90301=ADVANCED_FACE('',(#7837),#87619,.T.);
#90302=ADVANCED_FACE('',(#7838),#87620,.T.);
#90303=ADVANCED_FACE('',(#7839),#87621,.T.);
#90304=ADVANCED_FACE('',(#7840),#87622,.T.);
#90305=ADVANCED_FACE('',(#7841),#87623,.T.);
#90306=ADVANCED_FACE('',(#7842),#87624,.T.);
#90307=ADVANCED_FACE('',(#7843),#87625,.T.);
#90308=ADVANCED_FACE('',(#7844),#87626,.T.);
#90309=ADVANCED_FACE('',(#7845),#87627,.T.);
#90310=ADVANCED_FACE('',(#7846),#87628,.T.);
#90311=ADVANCED_FACE('',(#7847),#87629,.T.);
#90312=ADVANCED_FACE('',(#7848),#87630,.T.);
#90313=ADVANCED_FACE('',(#7849),#87631,.T.);
#90314=ADVANCED_FACE('',(#7850),#87632,.T.);
#90315=ADVANCED_FACE('',(#7851),#87633,.T.);
#90316=ADVANCED_FACE('',(#7852),#87634,.T.);
#90317=ADVANCED_FACE('',(#7853),#87635,.T.);
#90318=ADVANCED_FACE('',(#7854),#87636,.T.);
#90319=ADVANCED_FACE('',(#7855),#87637,.T.);
#90320=ADVANCED_FACE('',(#7856),#87638,.T.);
#90321=ADVANCED_FACE('',(#7857),#87639,.T.);
#90322=ADVANCED_FACE('',(#7858),#87640,.T.);
#90323=ADVANCED_FACE('',(#7859),#87641,.T.);
#90324=ADVANCED_FACE('',(#7860),#87642,.T.);
#90325=ADVANCED_FACE('',(#7861),#87643,.T.);
#90326=ADVANCED_FACE('',(#7862),#87644,.T.);
#90327=ADVANCED_FACE('',(#7863),#87645,.T.);
#90328=ADVANCED_FACE('',(#7864),#87646,.T.);
#90329=ADVANCED_FACE('',(#7865),#87647,.T.);
#90330=ADVANCED_FACE('',(#7866),#87648,.T.);
#90331=ADVANCED_FACE('',(#7867),#87649,.T.);
#90332=ADVANCED_FACE('',(#7868),#87650,.T.);
#90333=ADVANCED_FACE('',(#7869),#87651,.T.);
#90334=ADVANCED_FACE('',(#7870),#87652,.T.);
#90335=ADVANCED_FACE('',(#7871),#87653,.T.);
#90336=ADVANCED_FACE('',(#7872),#87654,.T.);
#90337=ADVANCED_FACE('',(#7873),#87655,.T.);
#90338=ADVANCED_FACE('',(#7874),#87656,.T.);
#90339=ADVANCED_FACE('',(#7875),#87657,.T.);
#90340=ADVANCED_FACE('',(#7876),#87658,.T.);
#90341=ADVANCED_FACE('',(#7877),#87659,.T.);
#90342=ADVANCED_FACE('',(#7878),#87660,.T.);
#90343=ADVANCED_FACE('',(#7879),#87661,.T.);
#90344=ADVANCED_FACE('',(#7880),#87662,.T.);
#90345=ADVANCED_FACE('',(#7881),#87663,.T.);
#90346=ADVANCED_FACE('',(#7882),#87664,.T.);
#90347=ADVANCED_FACE('',(#7883),#87665,.T.);
#90348=ADVANCED_FACE('',(#7884),#87666,.T.);
#90349=ADVANCED_FACE('',(#7885),#87667,.T.);
#90350=ADVANCED_FACE('',(#7886),#87668,.T.);
#90351=ADVANCED_FACE('',(#7887),#87669,.T.);
#90352=ADVANCED_FACE('',(#7888),#87670,.T.);
#90353=ADVANCED_FACE('',(#7889),#87671,.T.);
#90354=ADVANCED_FACE('',(#7890),#87672,.T.);
#90355=ADVANCED_FACE('',(#7891),#87673,.T.);
#90356=ADVANCED_FACE('',(#7892),#87674,.T.);
#90357=ADVANCED_FACE('',(#7893),#87675,.T.);
#90358=ADVANCED_FACE('',(#7894),#87676,.T.);
#90359=ADVANCED_FACE('',(#7895),#87677,.T.);
#90360=ADVANCED_FACE('',(#7896),#87678,.T.);
#90361=ADVANCED_FACE('',(#7897),#87679,.T.);
#90362=ADVANCED_FACE('',(#7898),#87680,.T.);
#90363=ADVANCED_FACE('',(#7899),#87681,.T.);
#90364=ADVANCED_FACE('',(#7900),#87682,.T.);
#90365=ADVANCED_FACE('',(#7901),#87683,.T.);
#90366=ADVANCED_FACE('',(#7902),#87684,.T.);
#90367=ADVANCED_FACE('',(#7903),#87685,.T.);
#90368=ADVANCED_FACE('',(#7904),#87686,.T.);
#90369=ADVANCED_FACE('',(#7905),#87687,.T.);
#90370=ADVANCED_FACE('',(#7906,#5185),#5596,.T.);
#90371=ADVANCED_FACE('',(#7907),#5597,.T.);
#90372=ADVANCED_FACE('',(#7908),#5598,.T.);
#90373=ADVANCED_FACE('',(#7909,#5186),#5599,.T.);
#90374=ADVANCED_FACE('',(#7910),#5600,.T.);
#90375=ADVANCED_FACE('',(#7911),#87688,.F.);
#90376=ADVANCED_FACE('',(#7912),#87689,.T.);
#90377=ADVANCED_FACE('',(#7913),#87690,.F.);
#90378=ADVANCED_FACE('',(#7914),#5601,.T.);
#90379=ADVANCED_FACE('',(#7915),#87691,.F.);
#90380=ADVANCED_FACE('',(#7916),#87692,.F.);
#90381=ADVANCED_FACE('',(#7917),#5602,.F.);
#90382=ADVANCED_FACE('',(#7918),#87693,.F.);
#90383=ADVANCED_FACE('',(#7919),#5603,.T.);
#90384=ADVANCED_FACE('',(#7920),#87694,.F.);
#90385=ADVANCED_FACE('',(#7921),#87695,.F.);
#90386=ADVANCED_FACE('',(#7922),#5604,.T.);
#90387=ADVANCED_FACE('',(#7923),#87696,.F.);
#90388=ADVANCED_FACE('',(#7924),#87697,.T.);
#90389=ADVANCED_FACE('',(#7925),#5605,.T.);
#90390=ADVANCED_FACE('',(#7926),#1848,.T.);
#90391=ADVANCED_FACE('',(#7927),#87698,.T.);
#90392=ADVANCED_FACE('',(#7928),#1849,.T.);
#90393=ADVANCED_FACE('',(#7929),#1850,.T.);
#90394=ADVANCED_FACE('',(#7930),#1851,.T.);
#90395=ADVANCED_FACE('',(#7931),#87699,.T.);
#90396=ADVANCED_FACE('',(#7932),#1852,.T.);
#90397=ADVANCED_FACE('',(#7933),#1853,.T.);
#90398=ADVANCED_FACE('',(#7934),#1854,.T.);
#90399=ADVANCED_FACE('',(#7935),#87700,.T.);
#90400=ADVANCED_FACE('',(#7936),#1855,.T.);
#90401=ADVANCED_FACE('',(#7937),#87701,.T.);
#90402=ADVANCED_FACE('',(#7938),#1856,.T.);
#90403=ADVANCED_FACE('',(#7939),#1857,.T.);
#90404=ADVANCED_FACE('',(#7940),#5606,.T.);
#90405=ADVANCED_FACE('',(#7941),#5607,.T.);
#94632=CLOSED_SHELL('',(#89904,#89905,#89906,#89907,#89908,#89909,#89910,
#89911,#89912,#89913,#89914,#89915,#89916,#89917,#89918,#89919,#89920,#89921,
#89922,#89923,#89924,#89925,#89926,#89927,#89928,#89929,#89930,#89931,#89932,
#89933,#89934,#89935,#89936,#89937,#89938,#89939,#89940,#89941,#89942,#89943,
#89944,#89945,#89946,#89947,#89948,#89949,#89950,#89951,#89952,#89953,#89954,
#89955,#89956,#89957,#89958,#89959,#89960,#89961,#89962,#89963,#89964,#89965,
#89966,#89967,#89968,#89969,#89970,#89971,#89972,#89973,#89974,#89975,#89976,
#89977,#89978,#89979,#89980,#89981,#89982,#89983,#89984,#89985,#89986,#89987,
#89988,#89989,#89990,#89991,#89992,#89993,#89994,#89995,#89996,#89997,#89998,
#89999,#90000,#90001,#90002,#90003,#90004,#90005,#90006,#90007,#90008,#90009,
#90010,#90011,#90012,#90013,#90014,#90015,#90016,#90017,#90018,#90019,#90020,
#90021,#90022,#90023,#90024,#90025,#90026,#90027,#90028,#90029,#90030,#90031,
#90032,#90033,#90034,#90035,#90036,#90037,#90038,#90039,#90040,#90041,#90042,
#90043,#90044,#90045,#90046,#90047,#90048,#90049,#90050,#90051,#90052,#90053,
#90054,#90055,#90056,#90057,#90058,#90059,#90060,#90061,#90062,#90063,#90064,
#90065,#90066,#90067,#90068,#90069,#90070,#90071,#90072,#90073,#90074,#90075,
#90076,#90077,#90078,#90079,#90080,#90081,#90082,#90083,#90084,#90085,#90086,
#90087,#90088,#90089,#90090,#90091,#90092,#90093,#90094,#90095,#90096,#90097,
#90098,#90099,#90100,#90101,#90102,#90103,#90104,#90105,#90106,#90107,#90108,
#90109,#90110,#90111,#90112,#90113,#90114,#90115,#90116,#90117,#90118,#90119,
#90120,#90121,#90122,#90123,#90124,#90125,#90126,#90127,#90128,#90129,#90130,
#90131,#90132,#90133,#90134,#90135,#90136,#90137,#90138,#90139,#90140,#90141,
#90142,#90143,#90144,#90145,#90146,#90147,#90148,#90149,#90150,#90151,#90152,
#90153,#90154,#90155,#90156,#90157,#90158,#90159,#90160,#90161,#90162,#90163,
#90164,#90165,#90166,#90167,#90168,#90169,#90170,#90171,#90172,#90173,#90174,
#90175,#90176,#90177,#90178,#90179,#90180,#90181,#90182,#90183,#90184,#90185,
#90186,#90187,#90188,#90189,#90190,#90191,#90192,#90193,#90194,#90195,#90196,
#90197,#90198,#90199,#90200));
#94633=CLOSED_SHELL('',(#90201,#90202,#90203,#90204,#90205,#90206,#90207,
#90208,#90209,#90210,#90211,#90212,#90213,#90214,#90215,#90216,#90217,#90218,
#90219,#90220,#90221,#90222,#90223,#90224,#90225,#90226,#90227,#90228,#90229,
#90230,#90231,#90232,#90233,#90234,#90235,#90236,#90237,#90238,#90239,#90240,
#90241,#90242,#90243,#90244,#90245,#90246,#90247,#90248,#90249,#90250,#90251,
#90252,#90253,#90254,#90255,#90256,#90257,#90258,#90259,#90260,#90261,#90262,
#90263,#90264,#90265,#90266,#90267,#90268,#90269,#90270,#90271,#90272,#90273,
#90274,#90275,#90276,#90277,#90278,#90279,#90280,#90281,#90282,#90283,#90284,
#90285,#90286,#90287,#90288,#90289,#90290,#90291,#90292,#90293,#90294,#90295,
#90296,#90297,#90298,#90299,#90300,#90301,#90302,#90303,#90304,#90305,#90306,
#90307,#90308,#90309,#90310,#90311,#90312,#90313,#90314,#90315,#90316,#90317,
#90318,#90319,#90320,#90321,#90322,#90323,#90324,#90325,#90326,#90327,#90328,
#90329,#90330,#90331,#90332,#90333,#90334,#90335,#90336,#90337,#90338,#90339,
#90340,#90341,#90342,#90343,#90344,#90345,#90346,#90347,#90348,#90349,#90350,
#90351,#90352,#90353,#90354,#90355,#90356,#90357,#90358,#90359,#90360,#90361,
#90362,#90363,#90364,#90365,#90366,#90367,#90368,#90369,#90370,#90371,#90372,
#90373,#90374,#90375,#90376,#90377,#90378,#90379,#90380,#90381,#90382,#90383,
#90384,#90385,#90386,#90387,#90388,#90389,#90390,#90391,#90392,#90393,#90394,
#90395,#90396,#90397,#90398,#90399,#90400,#90401,#90402,#90403,#90404,#90405));
#97243=AXIS2_PLACEMENT_3D('',#145873,#111496,#111497);
#97244=AXIS2_PLACEMENT_3D('',#145874,#111498,#111499);
#97245=AXIS2_PLACEMENT_3D('',#145888,#111500,#111501);
#97246=AXIS2_PLACEMENT_3D('',#145900,#111502,#111503);
#97247=AXIS2_PLACEMENT_3D('',#145901,#111504,#111505);
#97248=AXIS2_PLACEMENT_3D('',#145915,#111506,#111507);
#97249=AXIS2_PLACEMENT_3D('',#145927,#111508,#111509);
#97250=AXIS2_PLACEMENT_3D('',#145928,#111510,#111511);
#97251=AXIS2_PLACEMENT_3D('',#145942,#111512,#111513);
#97252=AXIS2_PLACEMENT_3D('',#145954,#111514,#111515);
#97253=AXIS2_PLACEMENT_3D('',#145955,#111516,#111517);
#97254=AXIS2_PLACEMENT_3D('',#145969,#111518,#111519);
#97255=AXIS2_PLACEMENT_3D('',#145981,#111520,#111521);
#97256=AXIS2_PLACEMENT_3D('',#145982,#111522,#111523);
#97257=AXIS2_PLACEMENT_3D('',#145996,#111524,#111525);
#97258=AXIS2_PLACEMENT_3D('',#146008,#111526,#111527);
#97259=AXIS2_PLACEMENT_3D('',#146009,#111528,#111529);
#97260=AXIS2_PLACEMENT_3D('',#146023,#111530,#111531);
#97261=AXIS2_PLACEMENT_3D('',#146035,#111532,#111533);
#97262=AXIS2_PLACEMENT_3D('',#146036,#111534,#111535);
#97263=AXIS2_PLACEMENT_3D('',#146050,#111536,#111537);
#97264=AXIS2_PLACEMENT_3D('',#146062,#111538,#111539);
#97265=AXIS2_PLACEMENT_3D('',#146063,#111540,#111541);
#97266=AXIS2_PLACEMENT_3D('',#146077,#111542,#111543);
#97267=AXIS2_PLACEMENT_3D('',#146089,#111544,#111545);
#97268=AXIS2_PLACEMENT_3D('',#146090,#111546,#111547);
#97269=AXIS2_PLACEMENT_3D('',#146104,#111548,#111549);
#97270=AXIS2_PLACEMENT_3D('',#146116,#111550,#111551);
#97271=AXIS2_PLACEMENT_3D('',#146117,#111552,#111553);
#97272=AXIS2_PLACEMENT_3D('',#146131,#111554,#111555);
#97273=AXIS2_PLACEMENT_3D('',#146143,#111556,#111557);
#97274=AXIS2_PLACEMENT_3D('',#146144,#111558,#111559);
#97275=AXIS2_PLACEMENT_3D('',#146158,#111560,#111561);
#97276=AXIS2_PLACEMENT_3D('',#146170,#111562,#111563);
#97277=AXIS2_PLACEMENT_3D('',#146171,#111564,#111565);
#97278=AXIS2_PLACEMENT_3D('',#146185,#111566,#111567);
#97279=AXIS2_PLACEMENT_3D('',#146197,#111568,#111569);
#97280=AXIS2_PLACEMENT_3D('',#146198,#111570,#111571);
#97281=AXIS2_PLACEMENT_3D('',#146212,#111572,#111573);
#97282=AXIS2_PLACEMENT_3D('',#146224,#111574,#111575);
#97283=AXIS2_PLACEMENT_3D('',#146225,#111576,#111577);
#97284=AXIS2_PLACEMENT_3D('',#146239,#111578,#111579);
#97285=AXIS2_PLACEMENT_3D('',#146251,#111580,#111581);
#97286=AXIS2_PLACEMENT_3D('',#146252,#111582,#111583);
#97287=AXIS2_PLACEMENT_3D('',#146266,#111584,#111585);
#97288=AXIS2_PLACEMENT_3D('',#146278,#111586,#111587);
#97289=AXIS2_PLACEMENT_3D('',#146279,#111588,#111589);
#97290=AXIS2_PLACEMENT_3D('',#146293,#111590,#111591);
#97291=AXIS2_PLACEMENT_3D('',#146305,#111592,#111593);
#97292=AXIS2_PLACEMENT_3D('',#146306,#111594,#111595);
#97293=AXIS2_PLACEMENT_3D('',#146320,#111596,#111597);
#97294=AXIS2_PLACEMENT_3D('',#146332,#111598,#111599);
#97295=AXIS2_PLACEMENT_3D('',#146333,#111600,#111601);
#97296=AXIS2_PLACEMENT_3D('',#146347,#111602,#111603);
#97297=AXIS2_PLACEMENT_3D('',#146359,#111604,#111605);
#97298=AXIS2_PLACEMENT_3D('',#146360,#111606,#111607);
#97299=AXIS2_PLACEMENT_3D('',#146374,#111608,#111609);
#97300=AXIS2_PLACEMENT_3D('',#146386,#111610,#111611);
#97301=AXIS2_PLACEMENT_3D('',#146387,#111612,#111613);
#97302=AXIS2_PLACEMENT_3D('',#146401,#111614,#111615);
#97303=AXIS2_PLACEMENT_3D('',#146413,#111616,#111617);
#97304=AXIS2_PLACEMENT_3D('',#146414,#111618,#111619);
#97305=AXIS2_PLACEMENT_3D('',#146428,#111620,#111621);
#97306=AXIS2_PLACEMENT_3D('',#146440,#111622,#111623);
#97307=AXIS2_PLACEMENT_3D('',#146441,#111624,#111625);
#97308=AXIS2_PLACEMENT_3D('',#146455,#111626,#111627);
#97309=AXIS2_PLACEMENT_3D('',#146467,#111628,#111629);
#97310=AXIS2_PLACEMENT_3D('',#146468,#111630,#111631);
#97311=AXIS2_PLACEMENT_3D('',#146482,#111632,#111633);
#97312=AXIS2_PLACEMENT_3D('',#146494,#111634,#111635);
#97313=AXIS2_PLACEMENT_3D('',#146495,#111636,#111637);
#97314=AXIS2_PLACEMENT_3D('',#146509,#111638,#111639);
#97315=AXIS2_PLACEMENT_3D('',#146521,#111640,#111641);
#97316=AXIS2_PLACEMENT_3D('',#146522,#111642,#111643);
#97317=AXIS2_PLACEMENT_3D('',#146536,#111644,#111645);
#97318=AXIS2_PLACEMENT_3D('',#146548,#111646,#111647);
#97319=AXIS2_PLACEMENT_3D('',#146549,#111648,#111649);
#97320=AXIS2_PLACEMENT_3D('',#146563,#111650,#111651);
#97321=AXIS2_PLACEMENT_3D('',#146575,#111652,#111653);
#97322=AXIS2_PLACEMENT_3D('',#146576,#111654,#111655);
#97323=AXIS2_PLACEMENT_3D('',#146590,#111656,#111657);
#97324=AXIS2_PLACEMENT_3D('',#146602,#111658,#111659);
#97325=AXIS2_PLACEMENT_3D('',#146603,#111660,#111661);
#97326=AXIS2_PLACEMENT_3D('',#146617,#111662,#111663);
#97327=AXIS2_PLACEMENT_3D('',#146629,#111664,#111665);
#97328=AXIS2_PLACEMENT_3D('',#146630,#111666,#111667);
#97329=AXIS2_PLACEMENT_3D('',#146644,#111668,#111669);
#97330=AXIS2_PLACEMENT_3D('',#146656,#111670,#111671);
#97331=AXIS2_PLACEMENT_3D('',#146657,#111672,#111673);
#97332=AXIS2_PLACEMENT_3D('',#146671,#111674,#111675);
#97333=AXIS2_PLACEMENT_3D('',#146683,#111676,#111677);
#97334=AXIS2_PLACEMENT_3D('',#146684,#111678,#111679);
#97335=AXIS2_PLACEMENT_3D('',#146698,#111680,#111681);
#97336=AXIS2_PLACEMENT_3D('',#146710,#111682,#111683);
#97337=AXIS2_PLACEMENT_3D('',#146711,#111684,#111685);
#97338=AXIS2_PLACEMENT_3D('',#146725,#111686,#111687);
#97339=AXIS2_PLACEMENT_3D('',#146737,#111688,#111689);
#97340=AXIS2_PLACEMENT_3D('',#146738,#111690,#111691);
#97341=AXIS2_PLACEMENT_3D('',#146752,#111692,#111693);
#97342=AXIS2_PLACEMENT_3D('',#146764,#111694,#111695);
#97343=AXIS2_PLACEMENT_3D('',#146765,#111696,#111697);
#97344=AXIS2_PLACEMENT_3D('',#146779,#111698,#111699);
#97345=AXIS2_PLACEMENT_3D('',#146791,#111700,#111701);
#97346=AXIS2_PLACEMENT_3D('',#146792,#111702,#111703);
#97347=AXIS2_PLACEMENT_3D('',#146806,#111704,#111705);
#97348=AXIS2_PLACEMENT_3D('',#146818,#111706,#111707);
#97349=AXIS2_PLACEMENT_3D('',#146819,#111708,#111709);
#97350=AXIS2_PLACEMENT_3D('',#146833,#111710,#111711);
#97351=AXIS2_PLACEMENT_3D('',#146845,#111712,#111713);
#97352=AXIS2_PLACEMENT_3D('',#146846,#111714,#111715);
#97353=AXIS2_PLACEMENT_3D('',#146860,#111716,#111717);
#97354=AXIS2_PLACEMENT_3D('',#146872,#111718,#111719);
#97355=AXIS2_PLACEMENT_3D('',#146873,#111720,#111721);
#97356=AXIS2_PLACEMENT_3D('',#146887,#111722,#111723);
#97357=AXIS2_PLACEMENT_3D('',#146899,#111724,#111725);
#97358=AXIS2_PLACEMENT_3D('',#146900,#111726,#111727);
#97359=AXIS2_PLACEMENT_3D('',#146914,#111728,#111729);
#97360=AXIS2_PLACEMENT_3D('',#146926,#111730,#111731);
#97361=AXIS2_PLACEMENT_3D('',#146927,#111732,#111733);
#97362=AXIS2_PLACEMENT_3D('',#146941,#111734,#111735);
#97363=AXIS2_PLACEMENT_3D('',#146953,#111736,#111737);
#97364=AXIS2_PLACEMENT_3D('',#146954,#111738,#111739);
#97365=AXIS2_PLACEMENT_3D('',#146968,#111740,#111741);
#97366=AXIS2_PLACEMENT_3D('',#146980,#111742,#111743);
#97367=AXIS2_PLACEMENT_3D('',#146981,#111744,#111745);
#97368=AXIS2_PLACEMENT_3D('',#146995,#111746,#111747);
#97369=AXIS2_PLACEMENT_3D('',#147007,#111748,#111749);
#97370=AXIS2_PLACEMENT_3D('',#147008,#111750,#111751);
#97371=AXIS2_PLACEMENT_3D('',#147022,#111752,#111753);
#97372=AXIS2_PLACEMENT_3D('',#147034,#111754,#111755);
#97373=AXIS2_PLACEMENT_3D('',#147035,#111756,#111757);
#97374=AXIS2_PLACEMENT_3D('',#147049,#111758,#111759);
#97375=AXIS2_PLACEMENT_3D('',#147061,#111760,#111761);
#97376=AXIS2_PLACEMENT_3D('',#147062,#111762,#111763);
#97377=AXIS2_PLACEMENT_3D('',#147076,#111764,#111765);
#97378=AXIS2_PLACEMENT_3D('',#147088,#111766,#111767);
#97379=AXIS2_PLACEMENT_3D('',#147089,#111768,#111769);
#97380=AXIS2_PLACEMENT_3D('',#147103,#111770,#111771);
#97381=AXIS2_PLACEMENT_3D('',#147115,#111772,#111773);
#97382=AXIS2_PLACEMENT_3D('',#147116,#111774,#111775);
#97383=AXIS2_PLACEMENT_3D('',#147130,#111776,#111777);
#97384=AXIS2_PLACEMENT_3D('',#147142,#111778,#111779);
#97385=AXIS2_PLACEMENT_3D('',#147143,#111780,#111781);
#97386=AXIS2_PLACEMENT_3D('',#147157,#111782,#111783);
#97387=AXIS2_PLACEMENT_3D('',#147169,#111784,#111785);
#97388=AXIS2_PLACEMENT_3D('',#147170,#111786,#111787);
#97389=AXIS2_PLACEMENT_3D('',#147184,#111788,#111789);
#97390=AXIS2_PLACEMENT_3D('',#147196,#111790,#111791);
#97391=AXIS2_PLACEMENT_3D('',#147197,#111792,#111793);
#97392=AXIS2_PLACEMENT_3D('',#147211,#111794,#111795);
#97393=AXIS2_PLACEMENT_3D('',#147223,#111796,#111797);
#97394=AXIS2_PLACEMENT_3D('',#147224,#111798,#111799);
#97395=AXIS2_PLACEMENT_3D('',#147238,#111800,#111801);
#97396=AXIS2_PLACEMENT_3D('',#147250,#111802,#111803);
#97397=AXIS2_PLACEMENT_3D('',#147251,#111804,#111805);
#97398=AXIS2_PLACEMENT_3D('',#147265,#111806,#111807);
#97399=AXIS2_PLACEMENT_3D('',#147277,#111808,#111809);
#97400=AXIS2_PLACEMENT_3D('',#147278,#111810,#111811);
#97401=AXIS2_PLACEMENT_3D('',#147292,#111812,#111813);
#97402=AXIS2_PLACEMENT_3D('',#147304,#111814,#111815);
#97403=AXIS2_PLACEMENT_3D('',#147305,#111816,#111817);
#97404=AXIS2_PLACEMENT_3D('',#147319,#111818,#111819);
#97405=AXIS2_PLACEMENT_3D('',#147331,#111820,#111821);
#97406=AXIS2_PLACEMENT_3D('',#147332,#111822,#111823);
#97407=AXIS2_PLACEMENT_3D('',#147346,#111824,#111825);
#97408=AXIS2_PLACEMENT_3D('',#147358,#111826,#111827);
#97409=AXIS2_PLACEMENT_3D('',#147359,#111828,#111829);
#97410=AXIS2_PLACEMENT_3D('',#147373,#111830,#111831);
#97411=AXIS2_PLACEMENT_3D('',#147385,#111832,#111833);
#97412=AXIS2_PLACEMENT_3D('',#147386,#111834,#111835);
#97413=AXIS2_PLACEMENT_3D('',#147400,#111836,#111837);
#97414=AXIS2_PLACEMENT_3D('',#147412,#111838,#111839);
#97415=AXIS2_PLACEMENT_3D('',#147413,#111840,#111841);
#97416=AXIS2_PLACEMENT_3D('',#147427,#111842,#111843);
#97417=AXIS2_PLACEMENT_3D('',#147439,#111844,#111845);
#97418=AXIS2_PLACEMENT_3D('',#147440,#111846,#111847);
#97419=AXIS2_PLACEMENT_3D('',#147454,#111848,#111849);
#97420=AXIS2_PLACEMENT_3D('',#147466,#111850,#111851);
#97421=AXIS2_PLACEMENT_3D('',#147467,#111852,#111853);
#97422=AXIS2_PLACEMENT_3D('',#147481,#111854,#111855);
#97423=AXIS2_PLACEMENT_3D('',#147493,#111856,#111857);
#97424=AXIS2_PLACEMENT_3D('',#147494,#111858,#111859);
#97425=AXIS2_PLACEMENT_3D('',#147508,#111860,#111861);
#97426=AXIS2_PLACEMENT_3D('',#147520,#111862,#111863);
#97427=AXIS2_PLACEMENT_3D('',#147521,#111864,#111865);
#97428=AXIS2_PLACEMENT_3D('',#147535,#111866,#111867);
#97429=AXIS2_PLACEMENT_3D('',#147547,#111868,#111869);
#97430=AXIS2_PLACEMENT_3D('',#147548,#111870,#111871);
#97431=AXIS2_PLACEMENT_3D('',#147562,#111872,#111873);
#97432=AXIS2_PLACEMENT_3D('',#147574,#111874,#111875);
#97433=AXIS2_PLACEMENT_3D('',#147575,#111876,#111877);
#97434=AXIS2_PLACEMENT_3D('',#147589,#111878,#111879);
#97435=AXIS2_PLACEMENT_3D('',#147601,#111880,#111881);
#97436=AXIS2_PLACEMENT_3D('',#147602,#111882,#111883);
#97437=AXIS2_PLACEMENT_3D('',#147616,#111884,#111885);
#97438=AXIS2_PLACEMENT_3D('',#147628,#111886,#111887);
#97439=AXIS2_PLACEMENT_3D('',#147629,#111888,#111889);
#97440=AXIS2_PLACEMENT_3D('',#147643,#111890,#111891);
#97441=AXIS2_PLACEMENT_3D('',#147655,#111892,#111893);
#97442=AXIS2_PLACEMENT_3D('',#147656,#111894,#111895);
#97443=AXIS2_PLACEMENT_3D('',#147670,#111896,#111897);
#97444=AXIS2_PLACEMENT_3D('',#147682,#111898,#111899);
#97445=AXIS2_PLACEMENT_3D('',#147683,#111900,#111901);
#97446=AXIS2_PLACEMENT_3D('',#147697,#111902,#111903);
#97447=AXIS2_PLACEMENT_3D('',#147709,#111904,#111905);
#97448=AXIS2_PLACEMENT_3D('',#147710,#111906,#111907);
#97449=AXIS2_PLACEMENT_3D('',#147724,#111908,#111909);
#97450=AXIS2_PLACEMENT_3D('',#147736,#111910,#111911);
#97451=AXIS2_PLACEMENT_3D('',#147737,#111912,#111913);
#97452=AXIS2_PLACEMENT_3D('',#147751,#111914,#111915);
#97453=AXIS2_PLACEMENT_3D('',#147763,#111916,#111917);
#97454=AXIS2_PLACEMENT_3D('',#147764,#111918,#111919);
#97455=AXIS2_PLACEMENT_3D('',#147767,#111920,#111921);
#97456=AXIS2_PLACEMENT_3D('',#147770,#111923,#111924);
#97457=AXIS2_PLACEMENT_3D('',#147771,#111925,#111926);
#97458=AXIS2_PLACEMENT_3D('',#147772,#111927,#111928);
#97459=AXIS2_PLACEMENT_3D('',#147775,#111929,#111930);
#97460=AXIS2_PLACEMENT_3D('',#147778,#111932,#111933);
#97461=AXIS2_PLACEMENT_3D('',#147779,#111934,#111935);
#97462=AXIS2_PLACEMENT_3D('',#147780,#111936,#111937);
#97463=AXIS2_PLACEMENT_3D('',#147783,#111938,#111939);
#97464=AXIS2_PLACEMENT_3D('',#147786,#111941,#111942);
#97465=AXIS2_PLACEMENT_3D('',#147787,#111943,#111944);
#97466=AXIS2_PLACEMENT_3D('',#147788,#111945,#111946);
#97467=AXIS2_PLACEMENT_3D('',#147791,#111947,#111948);
#97468=AXIS2_PLACEMENT_3D('',#147794,#111950,#111951);
#97469=AXIS2_PLACEMENT_3D('',#147795,#111952,#111953);
#97470=AXIS2_PLACEMENT_3D('',#147796,#111954,#111955);
#97471=AXIS2_PLACEMENT_3D('',#147798,#111956,#111957);
#97472=AXIS2_PLACEMENT_3D('',#147801,#111959,#111960);
#97473=AXIS2_PLACEMENT_3D('',#147802,#111961,#111962);
#97474=AXIS2_PLACEMENT_3D('',#147804,#111963,#111964);
#97475=AXIS2_PLACEMENT_3D('',#147807,#111966,#111967);
#97476=AXIS2_PLACEMENT_3D('',#147808,#111968,#111969);
#97477=AXIS2_PLACEMENT_3D('',#147811,#111970,#111971);
#97478=AXIS2_PLACEMENT_3D('',#147814,#111973,#111974);
#97479=AXIS2_PLACEMENT_3D('',#147815,#111975,#111976);
#97480=AXIS2_PLACEMENT_3D('',#147816,#111977,#111978);
#97481=AXIS2_PLACEMENT_3D('',#147818,#111979,#111980);
#97482=AXIS2_PLACEMENT_3D('',#147821,#111982,#111983);
#97483=AXIS2_PLACEMENT_3D('',#147822,#111984,#111985);
#97484=AXIS2_PLACEMENT_3D('',#147824,#111987,#111988);
#97485=AXIS2_PLACEMENT_3D('',#147826,#111990,#111991);
#97486=AXIS2_PLACEMENT_3D('',#148786,#111993,#111994);
#97487=AXIS2_PLACEMENT_3D('',#149722,#111995,#111996);
#97488=AXIS2_PLACEMENT_3D('',#152036,#111998,#111999);
#97489=AXIS2_PLACEMENT_3D('',#152039,#112001,#112002);
#97490=AXIS2_PLACEMENT_3D('',#152040,#112003,#112004);
#97491=AXIS2_PLACEMENT_3D('',#152042,#112006,#112007);
#97492=AXIS2_PLACEMENT_3D('',#152043,#112008,#112009);
#97493=AXIS2_PLACEMENT_3D('',#152044,#112010,#112011);
#97494=AXIS2_PLACEMENT_3D('',#152045,#112012,#112013);
#97495=AXIS2_PLACEMENT_3D('',#152046,#112014,#112015);
#97496=AXIS2_PLACEMENT_3D('',#152047,#112016,#112017);
#97497=AXIS2_PLACEMENT_3D('',#152048,#112018,#112019);
#97498=AXIS2_PLACEMENT_3D('',#152049,#112020,#112021);
#97499=AXIS2_PLACEMENT_3D('',#152050,#112022,#112023);
#97500=AXIS2_PLACEMENT_3D('',#152051,#112024,#112025);
#97501=AXIS2_PLACEMENT_3D('',#152052,#112026,#112027);
#97502=AXIS2_PLACEMENT_3D('',#152053,#112028,#112029);
#97503=AXIS2_PLACEMENT_3D('',#152054,#112030,#112031);
#97504=AXIS2_PLACEMENT_3D('',#152055,#112032,#112033);
#97505=AXIS2_PLACEMENT_3D('',#152056,#112034,#112035);
#97506=AXIS2_PLACEMENT_3D('',#152057,#112036,#112037);
#97507=AXIS2_PLACEMENT_3D('',#152058,#112038,#112039);
#97508=AXIS2_PLACEMENT_3D('',#152059,#112040,#112041);
#97509=AXIS2_PLACEMENT_3D('',#152060,#112042,#112043);
#97510=AXIS2_PLACEMENT_3D('',#152061,#112044,#112045);
#97511=AXIS2_PLACEMENT_3D('',#152062,#112046,#112047);
#97512=AXIS2_PLACEMENT_3D('',#152063,#112048,#112049);
#97513=AXIS2_PLACEMENT_3D('',#152064,#112050,#112051);
#97514=AXIS2_PLACEMENT_3D('',#152065,#112052,#112053);
#97515=AXIS2_PLACEMENT_3D('',#152066,#112054,#112055);
#97516=AXIS2_PLACEMENT_3D('',#152067,#112056,#112057);
#97517=AXIS2_PLACEMENT_3D('',#152068,#112058,#112059);
#97518=AXIS2_PLACEMENT_3D('',#152069,#112060,#112061);
#97519=AXIS2_PLACEMENT_3D('',#152070,#112062,#112063);
#97520=AXIS2_PLACEMENT_3D('',#152071,#112064,#112065);
#97521=AXIS2_PLACEMENT_3D('',#152072,#112066,#112067);
#97522=AXIS2_PLACEMENT_3D('',#152073,#112068,#112069);
#97523=AXIS2_PLACEMENT_3D('',#152074,#112070,#112071);
#97524=AXIS2_PLACEMENT_3D('',#152075,#112072,#112073);
#97525=AXIS2_PLACEMENT_3D('',#152076,#112074,#112075);
#97526=AXIS2_PLACEMENT_3D('',#152077,#112076,#112077);
#97527=AXIS2_PLACEMENT_3D('',#152078,#112078,#112079);
#97528=AXIS2_PLACEMENT_3D('',#152079,#112080,#112081);
#97529=AXIS2_PLACEMENT_3D('',#152080,#112082,#112083);
#97530=AXIS2_PLACEMENT_3D('',#152081,#112084,#112085);
#97531=AXIS2_PLACEMENT_3D('',#152082,#112086,#112087);
#97532=AXIS2_PLACEMENT_3D('',#152083,#112088,#112089);
#97533=AXIS2_PLACEMENT_3D('',#152084,#112090,#112091);
#97534=AXIS2_PLACEMENT_3D('',#152085,#112092,#112093);
#97535=AXIS2_PLACEMENT_3D('',#152086,#112094,#112095);
#97536=AXIS2_PLACEMENT_3D('',#152087,#112096,#112097);
#97537=AXIS2_PLACEMENT_3D('',#152088,#112098,#112099);
#97538=AXIS2_PLACEMENT_3D('',#152089,#112100,#112101);
#97539=AXIS2_PLACEMENT_3D('',#152090,#112102,#112103);
#97540=AXIS2_PLACEMENT_3D('',#152091,#112104,#112105);
#97541=AXIS2_PLACEMENT_3D('',#152092,#112106,#112107);
#97542=AXIS2_PLACEMENT_3D('',#152093,#112108,#112109);
#97543=AXIS2_PLACEMENT_3D('',#152094,#112110,#112111);
#97544=AXIS2_PLACEMENT_3D('',#152095,#112112,#112113);
#97545=AXIS2_PLACEMENT_3D('',#152096,#112114,#112115);
#97546=AXIS2_PLACEMENT_3D('',#152097,#112116,#112117);
#97547=AXIS2_PLACEMENT_3D('',#152098,#112118,#112119);
#97548=AXIS2_PLACEMENT_3D('',#152099,#112120,#112121);
#97549=AXIS2_PLACEMENT_3D('',#152100,#112122,#112123);
#97550=AXIS2_PLACEMENT_3D('',#152101,#112124,#112125);
#97551=AXIS2_PLACEMENT_3D('',#152102,#112126,#112127);
#97552=AXIS2_PLACEMENT_3D('',#152103,#112128,#112129);
#97553=AXIS2_PLACEMENT_3D('',#152104,#112130,#112131);
#97554=AXIS2_PLACEMENT_3D('',#152105,#112132,#112133);
#97555=AXIS2_PLACEMENT_3D('',#152106,#112134,#112135);
#97556=AXIS2_PLACEMENT_3D('',#152107,#112136,#112137);
#97557=AXIS2_PLACEMENT_3D('',#152108,#112138,#112139);
#97558=AXIS2_PLACEMENT_3D('',#152109,#112140,#112141);
#97559=AXIS2_PLACEMENT_3D('',#152110,#112142,#112143);
#97560=AXIS2_PLACEMENT_3D('',#152111,#112144,#112145);
#97561=AXIS2_PLACEMENT_3D('',#152112,#112146,#112147);
#97562=AXIS2_PLACEMENT_3D('',#152113,#112148,#112149);
#97563=AXIS2_PLACEMENT_3D('',#152114,#112150,#112151);
#97564=AXIS2_PLACEMENT_3D('',#152115,#112152,#112153);
#97565=AXIS2_PLACEMENT_3D('',#152116,#112154,#112155);
#97566=AXIS2_PLACEMENT_3D('',#152117,#112156,#112157);
#97567=AXIS2_PLACEMENT_3D('',#152118,#112158,#112159);
#97568=AXIS2_PLACEMENT_3D('',#152119,#112160,#112161);
#97569=AXIS2_PLACEMENT_3D('',#152120,#112162,#112163);
#97570=AXIS2_PLACEMENT_3D('',#152121,#112164,#112165);
#97571=AXIS2_PLACEMENT_3D('',#152122,#112166,#112167);
#97572=AXIS2_PLACEMENT_3D('',#152123,#112168,#112169);
#97573=AXIS2_PLACEMENT_3D('',#152124,#112170,#112171);
#97574=AXIS2_PLACEMENT_3D('',#152125,#112172,#112173);
#97575=AXIS2_PLACEMENT_3D('',#152126,#112174,#112175);
#97576=AXIS2_PLACEMENT_3D('',#152127,#112176,#112177);
#97577=AXIS2_PLACEMENT_3D('',#152128,#112178,#112179);
#97578=AXIS2_PLACEMENT_3D('',#152129,#112180,#112181);
#97579=AXIS2_PLACEMENT_3D('',#152130,#112182,#112183);
#97580=AXIS2_PLACEMENT_3D('',#152131,#112184,#112185);
#97581=AXIS2_PLACEMENT_3D('',#152132,#112186,#112187);
#97582=AXIS2_PLACEMENT_3D('',#152133,#112188,#112189);
#97583=AXIS2_PLACEMENT_3D('',#152134,#112190,#112191);
#97584=AXIS2_PLACEMENT_3D('',#152135,#112192,#112193);
#97585=AXIS2_PLACEMENT_3D('',#152136,#112194,#112195);
#97586=AXIS2_PLACEMENT_3D('',#152137,#112196,#112197);
#97587=AXIS2_PLACEMENT_3D('',#152138,#112198,#112199);
#97588=AXIS2_PLACEMENT_3D('',#152139,#112200,#112201);
#97589=AXIS2_PLACEMENT_3D('',#152140,#112202,#112203);
#97590=AXIS2_PLACEMENT_3D('',#152141,#112204,#112205);
#97591=AXIS2_PLACEMENT_3D('',#152142,#112206,#112207);
#97592=AXIS2_PLACEMENT_3D('',#152143,#112208,#112209);
#97593=AXIS2_PLACEMENT_3D('',#152144,#112210,#112211);
#97594=AXIS2_PLACEMENT_3D('',#152145,#112212,#112213);
#97595=AXIS2_PLACEMENT_3D('',#152146,#112214,#112215);
#97596=AXIS2_PLACEMENT_3D('',#152147,#112216,#112217);
#97597=AXIS2_PLACEMENT_3D('',#152148,#112218,#112219);
#97598=AXIS2_PLACEMENT_3D('',#152149,#112220,#112221);
#97599=AXIS2_PLACEMENT_3D('',#152150,#112222,#112223);
#97600=AXIS2_PLACEMENT_3D('',#152151,#112224,#112225);
#97601=AXIS2_PLACEMENT_3D('',#152152,#112226,#112227);
#97602=AXIS2_PLACEMENT_3D('',#152153,#112228,#112229);
#97603=AXIS2_PLACEMENT_3D('',#152154,#112230,#112231);
#97604=AXIS2_PLACEMENT_3D('',#152155,#112232,#112233);
#97605=AXIS2_PLACEMENT_3D('',#152156,#112234,#112235);
#97606=AXIS2_PLACEMENT_3D('',#152157,#112236,#112237);
#97607=AXIS2_PLACEMENT_3D('',#152158,#112238,#112239);
#97608=AXIS2_PLACEMENT_3D('',#152159,#112240,#112241);
#97609=AXIS2_PLACEMENT_3D('',#152160,#112242,#112243);
#97610=AXIS2_PLACEMENT_3D('',#152161,#112244,#112245);
#97611=AXIS2_PLACEMENT_3D('',#152162,#112246,#112247);
#97612=AXIS2_PLACEMENT_3D('',#152163,#112248,#112249);
#97613=AXIS2_PLACEMENT_3D('',#152164,#112250,#112251);
#97614=AXIS2_PLACEMENT_3D('',#152165,#112252,#112253);
#97615=AXIS2_PLACEMENT_3D('',#152166,#112254,#112255);
#97616=AXIS2_PLACEMENT_3D('',#152167,#112256,#112257);
#97617=AXIS2_PLACEMENT_3D('',#152168,#112258,#112259);
#97618=AXIS2_PLACEMENT_3D('',#152169,#112260,#112261);
#97619=AXIS2_PLACEMENT_3D('',#152170,#112262,#112263);
#97620=AXIS2_PLACEMENT_3D('',#152171,#112264,#112265);
#97621=AXIS2_PLACEMENT_3D('',#152172,#112266,#112267);
#97622=AXIS2_PLACEMENT_3D('',#152173,#112268,#112269);
#97623=AXIS2_PLACEMENT_3D('',#152174,#112270,#112271);
#97624=AXIS2_PLACEMENT_3D('',#152175,#112272,#112273);
#97625=AXIS2_PLACEMENT_3D('',#152176,#112274,#112275);
#97626=AXIS2_PLACEMENT_3D('',#152177,#112276,#112277);
#97627=AXIS2_PLACEMENT_3D('',#152178,#112278,#112279);
#97628=AXIS2_PLACEMENT_3D('',#152179,#112280,#112281);
#97629=AXIS2_PLACEMENT_3D('',#152180,#112282,#112283);
#97630=AXIS2_PLACEMENT_3D('',#152181,#112284,#112285);
#97631=AXIS2_PLACEMENT_3D('',#152182,#112286,#112287);
#97632=AXIS2_PLACEMENT_3D('',#152183,#112288,#112289);
#97633=AXIS2_PLACEMENT_3D('',#152184,#112290,#112291);
#97634=AXIS2_PLACEMENT_3D('',#152185,#112292,#112293);
#97635=AXIS2_PLACEMENT_3D('',#152186,#112294,#112295);
#97636=AXIS2_PLACEMENT_3D('',#152187,#112296,#112297);
#97637=AXIS2_PLACEMENT_3D('',#152188,#112298,#112299);
#97638=AXIS2_PLACEMENT_3D('',#152189,#112300,#112301);
#97639=AXIS2_PLACEMENT_3D('',#152190,#112302,#112303);
#97640=AXIS2_PLACEMENT_3D('',#152191,#112304,#112305);
#97641=AXIS2_PLACEMENT_3D('',#152192,#112306,#112307);
#97642=AXIS2_PLACEMENT_3D('',#152193,#112308,#112309);
#97643=AXIS2_PLACEMENT_3D('',#152194,#112310,#112311);
#97644=AXIS2_PLACEMENT_3D('',#152195,#112312,#112313);
#97645=AXIS2_PLACEMENT_3D('',#152196,#112314,#112315);
#97646=AXIS2_PLACEMENT_3D('',#152197,#112316,#112317);
#97647=AXIS2_PLACEMENT_3D('',#152198,#112318,#112319);
#97648=AXIS2_PLACEMENT_3D('',#152199,#112320,#112321);
#97649=AXIS2_PLACEMENT_3D('',#152200,#112322,#112323);
#97650=AXIS2_PLACEMENT_3D('',#152201,#112324,#112325);
#97651=AXIS2_PLACEMENT_3D('',#152202,#112326,#112327);
#97652=AXIS2_PLACEMENT_3D('',#152203,#112328,#112329);
#97653=AXIS2_PLACEMENT_3D('',#152204,#112330,#112331);
#97654=AXIS2_PLACEMENT_3D('',#152205,#112332,#112333);
#97655=AXIS2_PLACEMENT_3D('',#152206,#112334,#112335);
#97656=AXIS2_PLACEMENT_3D('',#152207,#112336,#112337);
#97657=AXIS2_PLACEMENT_3D('',#152208,#112338,#112339);
#97658=AXIS2_PLACEMENT_3D('',#152209,#112340,#112341);
#97659=AXIS2_PLACEMENT_3D('',#152210,#112342,#112343);
#97660=AXIS2_PLACEMENT_3D('',#152211,#112344,#112345);
#97661=AXIS2_PLACEMENT_3D('',#152212,#112346,#112347);
#97662=AXIS2_PLACEMENT_3D('',#152213,#112348,#112349);
#97663=AXIS2_PLACEMENT_3D('',#152214,#112350,#112351);
#97664=AXIS2_PLACEMENT_3D('',#152215,#112352,#112353);
#97665=AXIS2_PLACEMENT_3D('',#152216,#112354,#112355);
#97666=AXIS2_PLACEMENT_3D('',#152217,#112356,#112357);
#97667=AXIS2_PLACEMENT_3D('',#152218,#112358,#112359);
#97668=AXIS2_PLACEMENT_3D('',#152219,#112360,#112361);
#97669=AXIS2_PLACEMENT_3D('',#152220,#112362,#112363);
#97670=AXIS2_PLACEMENT_3D('',#152221,#112364,#112365);
#97671=AXIS2_PLACEMENT_3D('',#152222,#112366,#112367);
#97672=AXIS2_PLACEMENT_3D('',#152223,#112368,#112369);
#97673=AXIS2_PLACEMENT_3D('',#152224,#112370,#112371);
#97674=AXIS2_PLACEMENT_3D('',#152225,#112372,#112373);
#97675=AXIS2_PLACEMENT_3D('',#152226,#112374,#112375);
#97676=AXIS2_PLACEMENT_3D('',#152227,#112376,#112377);
#97677=AXIS2_PLACEMENT_3D('',#152228,#112378,#112379);
#97678=AXIS2_PLACEMENT_3D('',#152229,#112380,#112381);
#97679=AXIS2_PLACEMENT_3D('',#152230,#112382,#112383);
#97680=AXIS2_PLACEMENT_3D('',#152231,#112384,#112385);
#97681=AXIS2_PLACEMENT_3D('',#152232,#112386,#112387);
#97682=AXIS2_PLACEMENT_3D('',#152233,#112388,#112389);
#97683=AXIS2_PLACEMENT_3D('',#152234,#112390,#112391);
#97684=AXIS2_PLACEMENT_3D('',#152235,#112392,#112393);
#97685=AXIS2_PLACEMENT_3D('',#152236,#112394,#112395);
#97686=AXIS2_PLACEMENT_3D('',#152237,#112396,#112397);
#97687=AXIS2_PLACEMENT_3D('',#152238,#112398,#112399);
#97688=AXIS2_PLACEMENT_3D('',#152239,#112400,#112401);
#97689=AXIS2_PLACEMENT_3D('',#152240,#112402,#112403);
#97690=AXIS2_PLACEMENT_3D('',#152241,#112404,#112405);
#97691=AXIS2_PLACEMENT_3D('',#152242,#112406,#112407);
#97692=AXIS2_PLACEMENT_3D('',#152243,#112408,#112409);
#97693=AXIS2_PLACEMENT_3D('',#152244,#112410,#112411);
#97694=AXIS2_PLACEMENT_3D('',#152245,#112412,#112413);
#97695=AXIS2_PLACEMENT_3D('',#152246,#112414,#112415);
#97696=AXIS2_PLACEMENT_3D('',#152247,#112416,#112417);
#97697=AXIS2_PLACEMENT_3D('',#152248,#112418,#112419);
#97698=AXIS2_PLACEMENT_3D('',#152249,#112420,#112421);
#97699=AXIS2_PLACEMENT_3D('',#152250,#112422,#112423);
#97700=AXIS2_PLACEMENT_3D('',#152251,#112424,#112425);
#97701=AXIS2_PLACEMENT_3D('',#152252,#112426,#112427);
#97702=AXIS2_PLACEMENT_3D('',#152253,#112428,#112429);
#97703=AXIS2_PLACEMENT_3D('',#152254,#112430,#112431);
#97704=AXIS2_PLACEMENT_3D('',#152255,#112432,#112433);
#97705=AXIS2_PLACEMENT_3D('',#152256,#112434,#112435);
#97706=AXIS2_PLACEMENT_3D('',#152257,#112436,#112437);
#97707=AXIS2_PLACEMENT_3D('',#152258,#112438,#112439);
#97708=AXIS2_PLACEMENT_3D('',#152259,#112440,#112441);
#97709=AXIS2_PLACEMENT_3D('',#152260,#112442,#112443);
#97710=AXIS2_PLACEMENT_3D('',#152261,#112444,#112445);
#97711=AXIS2_PLACEMENT_3D('',#152262,#112446,#112447);
#97712=AXIS2_PLACEMENT_3D('',#152263,#112448,#112449);
#97713=AXIS2_PLACEMENT_3D('',#152264,#112450,#112451);
#97714=AXIS2_PLACEMENT_3D('',#152265,#112452,#112453);
#97715=AXIS2_PLACEMENT_3D('',#152266,#112454,#112455);
#97716=AXIS2_PLACEMENT_3D('',#152267,#112456,#112457);
#97717=AXIS2_PLACEMENT_3D('',#152268,#112458,#112459);
#97718=AXIS2_PLACEMENT_3D('',#152269,#112460,#112461);
#97719=AXIS2_PLACEMENT_3D('',#152270,#112462,#112463);
#97720=AXIS2_PLACEMENT_3D('',#152271,#112464,#112465);
#97721=AXIS2_PLACEMENT_3D('',#152272,#112466,#112467);
#97722=AXIS2_PLACEMENT_3D('',#152273,#112468,#112469);
#97723=AXIS2_PLACEMENT_3D('',#152274,#112470,#112471);
#97724=AXIS2_PLACEMENT_3D('',#152275,#112472,#112473);
#97725=AXIS2_PLACEMENT_3D('',#152276,#112474,#112475);
#97726=AXIS2_PLACEMENT_3D('',#152277,#112476,#112477);
#97727=AXIS2_PLACEMENT_3D('',#152278,#112478,#112479);
#97728=AXIS2_PLACEMENT_3D('',#152279,#112480,#112481);
#97729=AXIS2_PLACEMENT_3D('',#152280,#112482,#112483);
#97730=AXIS2_PLACEMENT_3D('',#152281,#112484,#112485);
#97731=AXIS2_PLACEMENT_3D('',#152282,#112486,#112487);
#97732=AXIS2_PLACEMENT_3D('',#152283,#112488,#112489);
#97733=AXIS2_PLACEMENT_3D('',#152284,#112490,#112491);
#97734=AXIS2_PLACEMENT_3D('',#152285,#112492,#112493);
#97735=AXIS2_PLACEMENT_3D('',#152286,#112494,#112495);
#97736=AXIS2_PLACEMENT_3D('',#152287,#112496,#112497);
#97737=AXIS2_PLACEMENT_3D('',#152288,#112498,#112499);
#97738=AXIS2_PLACEMENT_3D('',#152289,#112500,#112501);
#97739=AXIS2_PLACEMENT_3D('',#152290,#112502,#112503);
#97740=AXIS2_PLACEMENT_3D('',#152291,#112504,#112505);
#97741=AXIS2_PLACEMENT_3D('',#152292,#112506,#112507);
#97742=AXIS2_PLACEMENT_3D('',#152293,#112508,#112509);
#97743=AXIS2_PLACEMENT_3D('',#152294,#112510,#112511);
#97744=AXIS2_PLACEMENT_3D('',#152295,#112512,#112513);
#97745=AXIS2_PLACEMENT_3D('',#152296,#112514,#112515);
#97746=AXIS2_PLACEMENT_3D('',#152297,#112516,#112517);
#97747=AXIS2_PLACEMENT_3D('',#152298,#112518,#112519);
#97748=AXIS2_PLACEMENT_3D('',#152299,#112520,#112521);
#97749=AXIS2_PLACEMENT_3D('',#152300,#112522,#112523);
#97750=AXIS2_PLACEMENT_3D('',#152301,#112524,#112525);
#97751=AXIS2_PLACEMENT_3D('',#152302,#112526,#112527);
#97752=AXIS2_PLACEMENT_3D('',#152303,#112528,#112529);
#97753=AXIS2_PLACEMENT_3D('',#152304,#112530,#112531);
#97754=AXIS2_PLACEMENT_3D('',#152305,#112532,#112533);
#97755=AXIS2_PLACEMENT_3D('',#152306,#112534,#112535);
#97756=AXIS2_PLACEMENT_3D('',#152307,#112536,#112537);
#97757=AXIS2_PLACEMENT_3D('',#152308,#112538,#112539);
#97758=AXIS2_PLACEMENT_3D('',#152309,#112540,#112541);
#97759=AXIS2_PLACEMENT_3D('',#152310,#112542,#112543);
#97760=AXIS2_PLACEMENT_3D('',#152311,#112544,#112545);
#97761=AXIS2_PLACEMENT_3D('',#152312,#112546,#112547);
#97762=AXIS2_PLACEMENT_3D('',#152313,#112548,#112549);
#97763=AXIS2_PLACEMENT_3D('',#152314,#112550,#112551);
#97764=AXIS2_PLACEMENT_3D('',#152315,#112552,#112553);
#97765=AXIS2_PLACEMENT_3D('',#152316,#112554,#112555);
#97766=AXIS2_PLACEMENT_3D('',#152317,#112556,#112557);
#97767=AXIS2_PLACEMENT_3D('',#152318,#112558,#112559);
#97768=AXIS2_PLACEMENT_3D('',#152319,#112560,#112561);
#97769=AXIS2_PLACEMENT_3D('',#152320,#112562,#112563);
#97770=AXIS2_PLACEMENT_3D('',#152321,#112564,#112565);
#97771=AXIS2_PLACEMENT_3D('',#152322,#112566,#112567);
#97772=AXIS2_PLACEMENT_3D('',#152323,#112568,#112569);
#97773=AXIS2_PLACEMENT_3D('',#152324,#112570,#112571);
#97774=AXIS2_PLACEMENT_3D('',#152325,#112572,#112573);
#97775=AXIS2_PLACEMENT_3D('',#152326,#112574,#112575);
#97776=AXIS2_PLACEMENT_3D('',#152327,#112576,#112577);
#97777=AXIS2_PLACEMENT_3D('',#152328,#112578,#112579);
#97778=AXIS2_PLACEMENT_3D('',#152329,#112580,#112581);
#97779=AXIS2_PLACEMENT_3D('',#152330,#112582,#112583);
#97780=AXIS2_PLACEMENT_3D('',#152331,#112584,#112585);
#97781=AXIS2_PLACEMENT_3D('',#152332,#112586,#112587);
#97782=AXIS2_PLACEMENT_3D('',#152333,#112588,#112589);
#97783=AXIS2_PLACEMENT_3D('',#152334,#112590,#112591);
#97784=AXIS2_PLACEMENT_3D('',#152335,#112592,#112593);
#97785=AXIS2_PLACEMENT_3D('',#152336,#112594,#112595);
#97786=AXIS2_PLACEMENT_3D('',#152337,#112596,#112597);
#97787=AXIS2_PLACEMENT_3D('',#152338,#112598,#112599);
#97788=AXIS2_PLACEMENT_3D('',#152339,#112600,#112601);
#97789=AXIS2_PLACEMENT_3D('',#152340,#112602,#112603);
#97790=AXIS2_PLACEMENT_3D('',#152341,#112604,#112605);
#97791=AXIS2_PLACEMENT_3D('',#152342,#112606,#112607);
#97792=AXIS2_PLACEMENT_3D('',#152343,#112608,#112609);
#97793=AXIS2_PLACEMENT_3D('',#152344,#112610,#112611);
#97794=AXIS2_PLACEMENT_3D('',#152345,#112612,#112613);
#97795=AXIS2_PLACEMENT_3D('',#152346,#112614,#112615);
#97796=AXIS2_PLACEMENT_3D('',#152347,#112616,#112617);
#97797=AXIS2_PLACEMENT_3D('',#152348,#112618,#112619);
#97798=AXIS2_PLACEMENT_3D('',#152349,#112620,#112621);
#97799=AXIS2_PLACEMENT_3D('',#152350,#112622,#112623);
#97800=AXIS2_PLACEMENT_3D('',#152351,#112624,#112625);
#97801=AXIS2_PLACEMENT_3D('',#152352,#112626,#112627);
#97802=AXIS2_PLACEMENT_3D('',#152353,#112628,#112629);
#97803=AXIS2_PLACEMENT_3D('',#152354,#112630,#112631);
#97804=AXIS2_PLACEMENT_3D('',#152355,#112632,#112633);
#97805=AXIS2_PLACEMENT_3D('',#152356,#112634,#112635);
#97806=AXIS2_PLACEMENT_3D('',#152357,#112636,#112637);
#97807=AXIS2_PLACEMENT_3D('',#152358,#112638,#112639);
#97808=AXIS2_PLACEMENT_3D('',#152359,#112640,#112641);
#97809=AXIS2_PLACEMENT_3D('',#152360,#112642,#112643);
#97810=AXIS2_PLACEMENT_3D('',#152361,#112644,#112645);
#97811=AXIS2_PLACEMENT_3D('',#152362,#112646,#112647);
#97812=AXIS2_PLACEMENT_3D('',#152363,#112648,#112649);
#97813=AXIS2_PLACEMENT_3D('',#152364,#112650,#112651);
#97814=AXIS2_PLACEMENT_3D('',#152365,#112652,#112653);
#97815=AXIS2_PLACEMENT_3D('',#152366,#112654,#112655);
#97816=AXIS2_PLACEMENT_3D('',#152367,#112656,#112657);
#97817=AXIS2_PLACEMENT_3D('',#152368,#112658,#112659);
#97818=AXIS2_PLACEMENT_3D('',#152369,#112660,#112661);
#97819=AXIS2_PLACEMENT_3D('',#152370,#112662,#112663);
#97820=AXIS2_PLACEMENT_3D('',#152371,#112664,#112665);
#97821=AXIS2_PLACEMENT_3D('',#152372,#112666,#112667);
#97822=AXIS2_PLACEMENT_3D('',#152373,#112668,#112669);
#97823=AXIS2_PLACEMENT_3D('',#152374,#112670,#112671);
#97824=AXIS2_PLACEMENT_3D('',#152375,#112672,#112673);
#97825=AXIS2_PLACEMENT_3D('',#152376,#112674,#112675);
#97826=AXIS2_PLACEMENT_3D('',#152377,#112676,#112677);
#97827=AXIS2_PLACEMENT_3D('',#152378,#112678,#112679);
#97828=AXIS2_PLACEMENT_3D('',#152379,#112680,#112681);
#97829=AXIS2_PLACEMENT_3D('',#152380,#112682,#112683);
#97830=AXIS2_PLACEMENT_3D('',#152381,#112684,#112685);
#97831=AXIS2_PLACEMENT_3D('',#152382,#112686,#112687);
#97832=AXIS2_PLACEMENT_3D('',#152383,#112688,#112689);
#97833=AXIS2_PLACEMENT_3D('',#152384,#112690,#112691);
#97834=AXIS2_PLACEMENT_3D('',#152385,#112692,#112693);
#97835=AXIS2_PLACEMENT_3D('',#152386,#112694,#112695);
#97836=AXIS2_PLACEMENT_3D('',#152387,#112696,#112697);
#97837=AXIS2_PLACEMENT_3D('',#152388,#112698,#112699);
#97838=AXIS2_PLACEMENT_3D('',#152389,#112700,#112701);
#97839=AXIS2_PLACEMENT_3D('',#152390,#112702,#112703);
#97840=AXIS2_PLACEMENT_3D('',#152391,#112704,#112705);
#97841=AXIS2_PLACEMENT_3D('',#152392,#112706,#112707);
#97842=AXIS2_PLACEMENT_3D('',#152393,#112708,#112709);
#97843=AXIS2_PLACEMENT_3D('',#152394,#112710,#112711);
#97844=AXIS2_PLACEMENT_3D('',#152395,#112712,#112713);
#97845=AXIS2_PLACEMENT_3D('',#152397,#112714,#112715);
#97846=AXIS2_PLACEMENT_3D('',#152400,#112717,#112718);
#97847=AXIS2_PLACEMENT_3D('',#152401,#112719,#112720);
#97848=AXIS2_PLACEMENT_3D('',#152403,#112721,#112722);
#97849=AXIS2_PLACEMENT_3D('',#152406,#112724,#112725);
#97850=AXIS2_PLACEMENT_3D('',#152407,#112726,#112727);
#97851=AXIS2_PLACEMENT_3D('',#152409,#112728,#112729);
#97852=AXIS2_PLACEMENT_3D('',#152411,#112730,#112731);
#97853=AXIS2_PLACEMENT_3D('',#152412,#112732,#112733);
#97854=AXIS2_PLACEMENT_3D('',#152413,#112734,#112735);
#97855=AXIS2_PLACEMENT_3D('',#152415,#112736,#112737);
#97856=AXIS2_PLACEMENT_3D('',#152417,#112738,#112739);
#97857=AXIS2_PLACEMENT_3D('',#152418,#112740,#112741);
#97858=AXIS2_PLACEMENT_3D('',#152419,#112742,#112743);
#97859=AXIS2_PLACEMENT_3D('',#152422,#112744,#112745);
#97860=AXIS2_PLACEMENT_3D('',#152424,#112746,#112747);
#97861=AXIS2_PLACEMENT_3D('',#152425,#112748,#112749);
#97862=AXIS2_PLACEMENT_3D('',#152426,#112750,#112751);
#97863=AXIS2_PLACEMENT_3D('',#152427,#112752,#112753);
#97864=AXIS2_PLACEMENT_3D('',#152429,#112754,#112755);
#97865=AXIS2_PLACEMENT_3D('',#152431,#112756,#112757);
#97866=AXIS2_PLACEMENT_3D('',#152432,#112758,#112759);
#97867=AXIS2_PLACEMENT_3D('',#152433,#112760,#112761);
#97868=AXIS2_PLACEMENT_3D('',#152435,#112762,#112763);
#97869=AXIS2_PLACEMENT_3D('',#152437,#112764,#112765);
#97870=AXIS2_PLACEMENT_3D('',#152439,#112766,#112767);
#97871=AXIS2_PLACEMENT_3D('',#152440,#112768,#112769);
#97872=AXIS2_PLACEMENT_3D('',#152441,#112770,#112771);
#97873=AXIS2_PLACEMENT_3D('',#152444,#112772,#112773);
#97874=AXIS2_PLACEMENT_3D('',#152446,#112774,#112775);
#97875=AXIS2_PLACEMENT_3D('',#152448,#112776,#112777);
#97876=AXIS2_PLACEMENT_3D('',#152449,#112778,#112779);
#97877=AXIS2_PLACEMENT_3D('',#152450,#112780,#112781);
#97878=AXIS2_PLACEMENT_3D('',#152453,#112782,#112783);
#97879=AXIS2_PLACEMENT_3D('',#152455,#112784,#112785);
#97880=AXIS2_PLACEMENT_3D('',#152457,#112786,#112787);
#97881=AXIS2_PLACEMENT_3D('',#152458,#112788,#112789);
#97882=AXIS2_PLACEMENT_3D('',#152459,#112790,#112791);
#97883=AXIS2_PLACEMENT_3D('',#152461,#112792,#112793);
#97884=AXIS2_PLACEMENT_3D('',#152463,#112794,#112795);
#97885=AXIS2_PLACEMENT_3D('',#152465,#112796,#112797);
#97886=AXIS2_PLACEMENT_3D('',#152466,#112798,#112799);
#97887=AXIS2_PLACEMENT_3D('',#152467,#112800,#112801);
#97888=AXIS2_PLACEMENT_3D('',#152469,#112802,#112803);
#97889=AXIS2_PLACEMENT_3D('',#152471,#112804,#112805);
#97890=AXIS2_PLACEMENT_3D('',#152473,#112806,#112807);
#97891=AXIS2_PLACEMENT_3D('',#152474,#112808,#112809);
#97892=AXIS2_PLACEMENT_3D('',#152475,#112810,#112811);
#97893=AXIS2_PLACEMENT_3D('',#152477,#112812,#112813);
#97894=AXIS2_PLACEMENT_3D('',#152479,#112814,#112815);
#97895=AXIS2_PLACEMENT_3D('',#152481,#112816,#112817);
#97896=AXIS2_PLACEMENT_3D('',#152482,#112818,#112819);
#97897=AXIS2_PLACEMENT_3D('',#152483,#112820,#112821);
#97898=AXIS2_PLACEMENT_3D('',#152486,#112822,#112823);
#97899=AXIS2_PLACEMENT_3D('',#152490,#112825,#112826);
#97900=AXIS2_PLACEMENT_3D('',#152492,#112828,#112829);
#97901=AXIS2_PLACEMENT_3D('',#152495,#112830,#112831);
#97902=AXIS2_PLACEMENT_3D('',#152499,#112833,#112834);
#97903=AXIS2_PLACEMENT_3D('',#152501,#112836,#112837);
#97904=AXIS2_PLACEMENT_3D('',#152503,#112838,#112839);
#97905=AXIS2_PLACEMENT_3D('',#152505,#112841,#112842);
#97906=AXIS2_PLACEMENT_3D('',#152507,#112844,#112845);
#97907=AXIS2_PLACEMENT_3D('',#152509,#112847,#112848);
#97908=AXIS2_PLACEMENT_3D('',#152511,#112849,#112850);
#97909=AXIS2_PLACEMENT_3D('',#152513,#112852,#112853);
#97910=AXIS2_PLACEMENT_3D('',#152516,#112854,#112855);
#97911=AXIS2_PLACEMENT_3D('',#152520,#112857,#112858);
#97912=AXIS2_PLACEMENT_3D('',#152522,#112860,#112861);
#97913=AXIS2_PLACEMENT_3D('',#152525,#112862,#112863);
#97914=AXIS2_PLACEMENT_3D('',#152529,#112865,#112866);
#97915=AXIS2_PLACEMENT_3D('',#152531,#112868,#112869);
#97916=AXIS2_PLACEMENT_3D('',#152534,#112870,#112871);
#97917=AXIS2_PLACEMENT_3D('',#152538,#112873,#112874);
#97918=AXIS2_PLACEMENT_3D('',#152540,#112876,#112877);
#97919=AXIS2_PLACEMENT_3D('',#152543,#112878,#112879);
#97920=AXIS2_PLACEMENT_3D('',#152547,#112881,#112882);
#97921=AXIS2_PLACEMENT_3D('',#152549,#112884,#112885);
#97922=AXIS2_PLACEMENT_3D('',#152551,#112887,#112888);
#97923=AXIS2_PLACEMENT_3D('',#152554,#112889,#112890);
#97924=AXIS2_PLACEMENT_3D('',#152556,#112891,#112892);
#97925=AXIS2_PLACEMENT_3D('',#152558,#112893,#112894);
#97926=AXIS2_PLACEMENT_3D('',#152560,#112895,#112896);
#97927=AXIS2_PLACEMENT_3D('',#152562,#112897,#112898);
#97928=AXIS2_PLACEMENT_3D('',#152564,#112899,#112900);
#97929=AXIS2_PLACEMENT_3D('',#152566,#112901,#112902);
#97930=AXIS2_PLACEMENT_3D('',#152568,#112903,#112904);
#97931=AXIS2_PLACEMENT_3D('',#152570,#112905,#112906);
#97932=AXIS2_PLACEMENT_3D('',#152572,#112907,#112908);
#97933=AXIS2_PLACEMENT_3D('',#152574,#112909,#112910);
#97934=AXIS2_PLACEMENT_3D('',#152576,#112911,#112912);
#97935=AXIS2_PLACEMENT_3D('',#152578,#112913,#112914);
#97936=AXIS2_PLACEMENT_3D('',#152580,#112915,#112916);
#97937=AXIS2_PLACEMENT_3D('',#152582,#112917,#112918);
#97938=AXIS2_PLACEMENT_3D('',#152584,#112919,#112920);
#97939=AXIS2_PLACEMENT_3D('',#152586,#112921,#112922);
#97940=AXIS2_PLACEMENT_3D('',#152588,#112923,#112924);
#97941=AXIS2_PLACEMENT_3D('',#152590,#112925,#112926);
#97942=AXIS2_PLACEMENT_3D('',#152592,#112927,#112928);
#97943=AXIS2_PLACEMENT_3D('',#152594,#112929,#112930);
#97944=AXIS2_PLACEMENT_3D('',#152596,#112931,#112932);
#97945=AXIS2_PLACEMENT_3D('',#152598,#112933,#112934);
#97946=AXIS2_PLACEMENT_3D('',#152600,#112935,#112936);
#97947=AXIS2_PLACEMENT_3D('',#152602,#112937,#112938);
#97948=AXIS2_PLACEMENT_3D('',#152604,#112939,#112940);
#97949=AXIS2_PLACEMENT_3D('',#152606,#112941,#112942);
#97950=AXIS2_PLACEMENT_3D('',#152608,#112943,#112944);
#97951=AXIS2_PLACEMENT_3D('',#152610,#112945,#112946);
#97952=AXIS2_PLACEMENT_3D('',#152611,#112947,#112948);
#97953=AXIS2_PLACEMENT_3D('',#152613,#112949,#112950);
#97954=AXIS2_PLACEMENT_3D('',#152615,#112951,#112952);
#97955=AXIS2_PLACEMENT_3D('',#152616,#112953,#112954);
#97956=AXIS2_PLACEMENT_3D('',#152618,#112955,#112956);
#97957=AXIS2_PLACEMENT_3D('',#152620,#112957,#112958);
#97958=AXIS2_PLACEMENT_3D('',#152622,#112959,#112960);
#97959=AXIS2_PLACEMENT_3D('',#152624,#112961,#112962);
#97960=AXIS2_PLACEMENT_3D('',#152626,#112963,#112964);
#97961=AXIS2_PLACEMENT_3D('',#152628,#112965,#112966);
#97962=AXIS2_PLACEMENT_3D('',#152630,#112967,#112968);
#97963=AXIS2_PLACEMENT_3D('',#152632,#112969,#112970);
#97964=AXIS2_PLACEMENT_3D('',#152634,#112971,#112972);
#97965=AXIS2_PLACEMENT_3D('',#152636,#112973,#112974);
#97966=AXIS2_PLACEMENT_3D('',#152638,#112975,#112976);
#97967=AXIS2_PLACEMENT_3D('',#152640,#112977,#112978);
#97968=AXIS2_PLACEMENT_3D('',#152642,#112979,#112980);
#97969=AXIS2_PLACEMENT_3D('',#152644,#112981,#112982);
#97970=AXIS2_PLACEMENT_3D('',#152646,#112983,#112984);
#97971=AXIS2_PLACEMENT_3D('',#152648,#112985,#112986);
#97972=AXIS2_PLACEMENT_3D('',#152650,#112987,#112988);
#97973=AXIS2_PLACEMENT_3D('',#152652,#112989,#112990);
#97974=AXIS2_PLACEMENT_3D('',#152654,#112991,#112992);
#97975=AXIS2_PLACEMENT_3D('',#152656,#112993,#112994);
#97976=AXIS2_PLACEMENT_3D('',#152658,#112995,#112996);
#97977=AXIS2_PLACEMENT_3D('',#152660,#112997,#112998);
#97978=AXIS2_PLACEMENT_3D('',#152662,#112999,#113000);
#97979=AXIS2_PLACEMENT_3D('',#152664,#113001,#113002);
#97980=AXIS2_PLACEMENT_3D('',#152666,#113003,#113004);
#97981=AXIS2_PLACEMENT_3D('',#152668,#113005,#113006);
#97982=AXIS2_PLACEMENT_3D('',#152670,#113007,#113008);
#97983=AXIS2_PLACEMENT_3D('',#152672,#113009,#113010);
#97984=AXIS2_PLACEMENT_3D('',#152674,#113011,#113012);
#97985=AXIS2_PLACEMENT_3D('',#152676,#113013,#113014);
#97986=AXIS2_PLACEMENT_3D('',#152678,#113015,#113016);
#97987=AXIS2_PLACEMENT_3D('',#152680,#113017,#113018);
#97988=AXIS2_PLACEMENT_3D('',#152682,#113019,#113020);
#97989=AXIS2_PLACEMENT_3D('',#152684,#113021,#113022);
#97990=AXIS2_PLACEMENT_3D('',#152686,#113023,#113024);
#97991=AXIS2_PLACEMENT_3D('',#152688,#113025,#113026);
#97992=AXIS2_PLACEMENT_3D('',#152690,#113027,#113028);
#97993=AXIS2_PLACEMENT_3D('',#152692,#113029,#113030);
#97994=AXIS2_PLACEMENT_3D('',#152694,#113031,#113032);
#97995=AXIS2_PLACEMENT_3D('',#152696,#113033,#113034);
#97996=AXIS2_PLACEMENT_3D('',#152698,#113035,#113036);
#97997=AXIS2_PLACEMENT_3D('',#152700,#113037,#113038);
#97998=AXIS2_PLACEMENT_3D('',#152702,#113039,#113040);
#97999=AXIS2_PLACEMENT_3D('',#152704,#113041,#113042);
#98000=AXIS2_PLACEMENT_3D('',#152706,#113043,#113044);
#98001=AXIS2_PLACEMENT_3D('',#152708,#113045,#113046);
#98002=AXIS2_PLACEMENT_3D('',#152710,#113047,#113048);
#98003=AXIS2_PLACEMENT_3D('',#152712,#113049,#113050);
#98004=AXIS2_PLACEMENT_3D('',#152714,#113051,#113052);
#98005=AXIS2_PLACEMENT_3D('',#152716,#113053,#113054);
#98006=AXIS2_PLACEMENT_3D('',#152718,#113055,#113056);
#98007=AXIS2_PLACEMENT_3D('',#152720,#113057,#113058);
#98008=AXIS2_PLACEMENT_3D('',#152722,#113059,#113060);
#98009=AXIS2_PLACEMENT_3D('',#152724,#113061,#113062);
#98010=AXIS2_PLACEMENT_3D('',#152726,#113063,#113064);
#98011=AXIS2_PLACEMENT_3D('',#152728,#113065,#113066);
#98012=AXIS2_PLACEMENT_3D('',#152730,#113067,#113068);
#98013=AXIS2_PLACEMENT_3D('',#152732,#113069,#113070);
#98014=AXIS2_PLACEMENT_3D('',#152734,#113071,#113072);
#98015=AXIS2_PLACEMENT_3D('',#152736,#113073,#113074);
#98016=AXIS2_PLACEMENT_3D('',#152738,#113075,#113076);
#98017=AXIS2_PLACEMENT_3D('',#152740,#113077,#113078);
#98018=AXIS2_PLACEMENT_3D('',#152742,#113079,#113080);
#98019=AXIS2_PLACEMENT_3D('',#152744,#113081,#113082);
#98020=AXIS2_PLACEMENT_3D('',#152746,#113083,#113084);
#98021=AXIS2_PLACEMENT_3D('',#152748,#113085,#113086);
#98022=AXIS2_PLACEMENT_3D('',#152750,#113087,#113088);
#98023=AXIS2_PLACEMENT_3D('',#152752,#113089,#113090);
#98024=AXIS2_PLACEMENT_3D('',#152754,#113091,#113092);
#98025=AXIS2_PLACEMENT_3D('',#152756,#113093,#113094);
#98026=AXIS2_PLACEMENT_3D('',#152758,#113095,#113096);
#98027=AXIS2_PLACEMENT_3D('',#152760,#113097,#113098);
#98028=AXIS2_PLACEMENT_3D('',#152762,#113099,#113100);
#98029=AXIS2_PLACEMENT_3D('',#152764,#113101,#113102);
#98030=AXIS2_PLACEMENT_3D('',#152766,#113103,#113104);
#98031=AXIS2_PLACEMENT_3D('',#152768,#113105,#113106);
#98032=AXIS2_PLACEMENT_3D('',#152770,#113107,#113108);
#98033=AXIS2_PLACEMENT_3D('',#152772,#113109,#113110);
#98034=AXIS2_PLACEMENT_3D('',#152774,#113111,#113112);
#98035=AXIS2_PLACEMENT_3D('',#152776,#113113,#113114);
#98036=AXIS2_PLACEMENT_3D('',#152778,#113115,#113116);
#98037=AXIS2_PLACEMENT_3D('',#152780,#113117,#113118);
#98038=AXIS2_PLACEMENT_3D('',#152782,#113119,#113120);
#98039=AXIS2_PLACEMENT_3D('',#152784,#113121,#113122);
#98040=AXIS2_PLACEMENT_3D('',#152785,#113123,#113124);
#98041=AXIS2_PLACEMENT_3D('',#152787,#113125,#113126);
#98042=AXIS2_PLACEMENT_3D('',#152789,#113127,#113128);
#98043=AXIS2_PLACEMENT_3D('',#152790,#113129,#113130);
#98044=AXIS2_PLACEMENT_3D('',#152792,#113131,#113132);
#98045=AXIS2_PLACEMENT_3D('',#152794,#113133,#113134);
#98046=AXIS2_PLACEMENT_3D('',#152796,#113135,#113136);
#98047=AXIS2_PLACEMENT_3D('',#152798,#113137,#113138);
#98048=AXIS2_PLACEMENT_3D('',#152800,#113139,#113140);
#98049=AXIS2_PLACEMENT_3D('',#152802,#113141,#113142);
#98050=AXIS2_PLACEMENT_3D('',#152804,#113143,#113144);
#98051=AXIS2_PLACEMENT_3D('',#152806,#113145,#113146);
#98052=AXIS2_PLACEMENT_3D('',#152808,#113147,#113148);
#98053=AXIS2_PLACEMENT_3D('',#152810,#113149,#113150);
#98054=AXIS2_PLACEMENT_3D('',#152812,#113151,#113152);
#98055=AXIS2_PLACEMENT_3D('',#152814,#113153,#113154);
#98056=AXIS2_PLACEMENT_3D('',#152816,#113155,#113156);
#98057=AXIS2_PLACEMENT_3D('',#152818,#113157,#113158);
#98058=AXIS2_PLACEMENT_3D('',#152820,#113159,#113160);
#98059=AXIS2_PLACEMENT_3D('',#152822,#113161,#113162);
#98060=AXIS2_PLACEMENT_3D('',#152824,#113163,#113164);
#98061=AXIS2_PLACEMENT_3D('',#152826,#113165,#113166);
#98062=AXIS2_PLACEMENT_3D('',#152828,#113167,#113168);
#98063=AXIS2_PLACEMENT_3D('',#152830,#113169,#113170);
#98064=AXIS2_PLACEMENT_3D('',#152832,#113171,#113172);
#98065=AXIS2_PLACEMENT_3D('',#152834,#113173,#113174);
#98066=AXIS2_PLACEMENT_3D('',#152835,#113175,#113176);
#98067=AXIS2_PLACEMENT_3D('',#152838,#113177,#113178);
#98068=AXIS2_PLACEMENT_3D('',#152840,#113179,#113180);
#98069=AXIS2_PLACEMENT_3D('',#152843,#113182,#113183);
#98070=AXIS2_PLACEMENT_3D('',#152845,#113184,#113185);
#98071=AXIS2_PLACEMENT_3D('',#152848,#113187,#113188);
#98072=AXIS2_PLACEMENT_3D('',#152853,#113190,#113191);
#98073=AXIS2_PLACEMENT_3D('',#152854,#113192,#113193);
#98074=AXIS2_PLACEMENT_3D('',#152858,#113195,#113196);
#98075=AXIS2_PLACEMENT_3D('',#152860,#113197,#113198);
#98076=AXIS2_PLACEMENT_3D('',#152861,#113199,#113200);
#98077=AXIS2_PLACEMENT_3D('',#152862,#113201,#113202);
#98078=AXIS2_PLACEMENT_3D('',#152867,#113205,#113206);
#98079=AXIS2_PLACEMENT_3D('',#152868,#113207,#113208);
#98080=AXIS2_PLACEMENT_3D('',#152872,#113210,#113211);
#98081=AXIS2_PLACEMENT_3D('',#152874,#113213,#113214);
#98082=AXIS2_PLACEMENT_3D('',#152879,#113217,#113218);
#98083=AXIS2_PLACEMENT_3D('',#152880,#113219,#113220);
#98084=AXIS2_PLACEMENT_3D('',#152885,#113223,#113224);
#98085=AXIS2_PLACEMENT_3D('',#152886,#113225,#113226);
#98086=AXIS2_PLACEMENT_3D('',#152891,#113229,#113230);
#98087=AXIS2_PLACEMENT_3D('',#152892,#113231,#113232);
#98088=AXIS2_PLACEMENT_3D('',#152895,#113234,#113235);
#98089=AXIS2_PLACEMENT_3D('',#152896,#113236,#113237);
#98090=AXIS2_PLACEMENT_3D('',#152899,#113239,#113240);
#98091=AXIS2_PLACEMENT_3D('',#152900,#113241,#113242);
#98092=AXIS2_PLACEMENT_3D('',#152904,#113244,#113245);
#98093=AXIS2_PLACEMENT_3D('',#152906,#113247,#113248);
#98094=AXIS2_PLACEMENT_3D('',#152911,#113251,#113252);
#98095=AXIS2_PLACEMENT_3D('',#152912,#113253,#113254);
#98096=AXIS2_PLACEMENT_3D('',#152917,#113257,#113258);
#98097=AXIS2_PLACEMENT_3D('',#152918,#113259,#113260);
#98098=AXIS2_PLACEMENT_3D('',#152922,#113262,#113263);
#98099=AXIS2_PLACEMENT_3D('',#152924,#113265,#113266);
#98100=AXIS2_PLACEMENT_3D('',#152929,#113269,#113270);
#98101=AXIS2_PLACEMENT_3D('',#152930,#113271,#113272);
#98102=AXIS2_PLACEMENT_3D('',#152932,#113273,#113274);
#98103=AXIS2_PLACEMENT_3D('',#152934,#113276,#113277);
#98104=AXIS2_PLACEMENT_3D('',#152936,#113278,#113279);
#98105=AXIS2_PLACEMENT_3D('',#152938,#113281,#113282);
#98106=AXIS2_PLACEMENT_3D('',#152942,#113284,#113285);
#98107=AXIS2_PLACEMENT_3D('',#152944,#113287,#113288);
#98108=AXIS2_PLACEMENT_3D('',#152949,#113291,#113292);
#98109=AXIS2_PLACEMENT_3D('',#152950,#113293,#113294);
#98110=AXIS2_PLACEMENT_3D('',#152954,#113296,#113297);
#98111=AXIS2_PLACEMENT_3D('',#152956,#113299,#113300);
#98112=AXIS2_PLACEMENT_3D('',#152961,#113303,#113304);
#98113=AXIS2_PLACEMENT_3D('',#152962,#113305,#113306);
#98114=AXIS2_PLACEMENT_3D('',#152967,#113309,#113310);
#98115=AXIS2_PLACEMENT_3D('',#152968,#113311,#113312);
#98116=AXIS2_PLACEMENT_3D('',#152972,#113314,#113315);
#98117=AXIS2_PLACEMENT_3D('',#152974,#113317,#113318);
#98118=AXIS2_PLACEMENT_3D('',#152979,#113321,#113322);
#98119=AXIS2_PLACEMENT_3D('',#152980,#113323,#113324);
#98120=AXIS2_PLACEMENT_3D('',#152984,#113326,#113327);
#98121=AXIS2_PLACEMENT_3D('',#152986,#113329,#113330);
#98122=AXIS2_PLACEMENT_3D('',#152990,#113332,#113333);
#98123=AXIS2_PLACEMENT_3D('',#152992,#113335,#113336);
#98124=AXIS2_PLACEMENT_3D('',#152996,#113338,#113339);
#98125=AXIS2_PLACEMENT_3D('',#152998,#113341,#113342);
#98126=AXIS2_PLACEMENT_3D('',#153003,#113345,#113346);
#98127=AXIS2_PLACEMENT_3D('',#153004,#113347,#113348);
#98128=AXIS2_PLACEMENT_3D('',#153008,#113350,#113351);
#98129=AXIS2_PLACEMENT_3D('',#153010,#113353,#113354);
#98130=AXIS2_PLACEMENT_3D('',#153015,#113357,#113358);
#98131=AXIS2_PLACEMENT_3D('',#153016,#113359,#113360);
#98132=AXIS2_PLACEMENT_3D('',#153021,#113363,#113364);
#98133=AXIS2_PLACEMENT_3D('',#153022,#113365,#113366);
#98134=AXIS2_PLACEMENT_3D('',#153026,#113368,#113369);
#98135=AXIS2_PLACEMENT_3D('',#153028,#113371,#113372);
#98136=AXIS2_PLACEMENT_3D('',#153033,#113375,#113376);
#98137=AXIS2_PLACEMENT_3D('',#153034,#113377,#113378);
#98138=AXIS2_PLACEMENT_3D('',#153038,#113380,#113381);
#98139=AXIS2_PLACEMENT_3D('',#153040,#113383,#113384);
#98140=AXIS2_PLACEMENT_3D('',#153044,#113386,#113387);
#98141=AXIS2_PLACEMENT_3D('',#153046,#113389,#113390);
#98142=AXIS2_PLACEMENT_3D('',#153050,#113392,#113393);
#98143=AXIS2_PLACEMENT_3D('',#153052,#113395,#113396);
#98144=AXIS2_PLACEMENT_3D('',#153057,#113399,#113400);
#98145=AXIS2_PLACEMENT_3D('',#153058,#113401,#113402);
#98146=AXIS2_PLACEMENT_3D('',#153063,#113405,#113406);
#98147=AXIS2_PLACEMENT_3D('',#153064,#113407,#113408);
#98148=AXIS2_PLACEMENT_3D('',#153069,#113411,#113412);
#98149=AXIS2_PLACEMENT_3D('',#153070,#113413,#113414);
#98150=AXIS2_PLACEMENT_3D('',#153072,#113415,#113416);
#98151=AXIS2_PLACEMENT_3D('',#153074,#113417,#113418);
#98152=AXIS2_PLACEMENT_3D('',#153076,#113419,#113420);
#98153=AXIS2_PLACEMENT_3D('',#153077,#113421,#113422);
#98154=AXIS2_PLACEMENT_3D('',#153079,#113423,#113424);
#98155=AXIS2_PLACEMENT_3D('',#153081,#113425,#113426);
#98156=AXIS2_PLACEMENT_3D('',#153082,#113427,#113428);
#98157=AXIS2_PLACEMENT_3D('',#153084,#113429,#113430);
#98158=AXIS2_PLACEMENT_3D('',#153086,#113431,#113432);
#98159=AXIS2_PLACEMENT_3D('',#153087,#113433,#113434);
#98160=AXIS2_PLACEMENT_3D('',#153089,#113435,#113436);
#98161=AXIS2_PLACEMENT_3D('',#153091,#113437,#113438);
#98162=AXIS2_PLACEMENT_3D('',#153092,#113439,#113440);
#98163=AXIS2_PLACEMENT_3D('',#153094,#113441,#113442);
#98164=AXIS2_PLACEMENT_3D('',#153096,#113443,#113444);
#98165=AXIS2_PLACEMENT_3D('',#153097,#113445,#113446);
#98166=AXIS2_PLACEMENT_3D('',#153099,#113447,#113448);
#98167=AXIS2_PLACEMENT_3D('',#153100,#113449,#113450);
#98168=AXIS2_PLACEMENT_3D('',#153102,#113451,#113452);
#98169=AXIS2_PLACEMENT_3D('',#153103,#113453,#113454);
#98170=AXIS2_PLACEMENT_3D('',#153105,#113455,#113456);
#98171=AXIS2_PLACEMENT_3D('',#153107,#113457,#113458);
#98172=AXIS2_PLACEMENT_3D('',#153109,#113459,#113460);
#98173=AXIS2_PLACEMENT_3D('',#153111,#113461,#113462);
#98174=AXIS2_PLACEMENT_3D('',#153113,#113463,#113464);
#98175=AXIS2_PLACEMENT_3D('',#153115,#113465,#113466);
#98176=AXIS2_PLACEMENT_3D('',#153116,#113467,#113468);
#98177=AXIS2_PLACEMENT_3D('',#153118,#113469,#113470);
#98178=AXIS2_PLACEMENT_3D('',#153120,#113471,#113472);
#98179=AXIS2_PLACEMENT_3D('',#153121,#113473,#113474);
#98180=AXIS2_PLACEMENT_3D('',#153123,#113475,#113476);
#98181=AXIS2_PLACEMENT_3D('',#153125,#113477,#113478);
#98182=AXIS2_PLACEMENT_3D('',#153126,#113479,#113480);
#98183=AXIS2_PLACEMENT_3D('',#153128,#113481,#113482);
#98184=AXIS2_PLACEMENT_3D('',#153130,#113483,#113484);
#98185=AXIS2_PLACEMENT_3D('',#153131,#113485,#113486);
#98186=AXIS2_PLACEMENT_3D('',#153133,#113487,#113488);
#98187=AXIS2_PLACEMENT_3D('',#153135,#113489,#113490);
#98188=AXIS2_PLACEMENT_3D('',#153136,#113491,#113492);
#98189=AXIS2_PLACEMENT_3D('',#153138,#113493,#113494);
#98190=AXIS2_PLACEMENT_3D('',#153140,#113495,#113496);
#98191=AXIS2_PLACEMENT_3D('',#153141,#113497,#113498);
#98192=AXIS2_PLACEMENT_3D('',#153143,#113499,#113500);
#98193=AXIS2_PLACEMENT_3D('',#153145,#113501,#113502);
#98194=AXIS2_PLACEMENT_3D('',#153146,#113503,#113504);
#98195=AXIS2_PLACEMENT_3D('',#153148,#113505,#113506);
#98196=AXIS2_PLACEMENT_3D('',#153150,#113507,#113508);
#98197=AXIS2_PLACEMENT_3D('',#153151,#113509,#113510);
#98198=AXIS2_PLACEMENT_3D('',#153153,#113511,#113512);
#98199=AXIS2_PLACEMENT_3D('',#153155,#113513,#113514);
#98200=AXIS2_PLACEMENT_3D('',#153156,#113515,#113516);
#98201=AXIS2_PLACEMENT_3D('',#153158,#113517,#113518);
#98202=AXIS2_PLACEMENT_3D('',#153160,#113519,#113520);
#98203=AXIS2_PLACEMENT_3D('',#153161,#113521,#113522);
#98204=AXIS2_PLACEMENT_3D('',#153163,#113523,#113524);
#98205=AXIS2_PLACEMENT_3D('',#153165,#113525,#113526);
#98206=AXIS2_PLACEMENT_3D('',#153166,#113527,#113528);
#98207=AXIS2_PLACEMENT_3D('',#153168,#113529,#113530);
#98208=AXIS2_PLACEMENT_3D('',#153170,#113531,#113532);
#98209=AXIS2_PLACEMENT_3D('',#153171,#113533,#113534);
#98210=AXIS2_PLACEMENT_3D('',#153173,#113535,#113536);
#98211=AXIS2_PLACEMENT_3D('',#153175,#113537,#113538);
#98212=AXIS2_PLACEMENT_3D('',#153176,#113539,#113540);
#98213=AXIS2_PLACEMENT_3D('',#153178,#113541,#113542);
#98214=AXIS2_PLACEMENT_3D('',#153180,#113543,#113544);
#98215=AXIS2_PLACEMENT_3D('',#153181,#113545,#113546);
#98216=AXIS2_PLACEMENT_3D('',#153183,#113547,#113548);
#98217=AXIS2_PLACEMENT_3D('',#153185,#113549,#113550);
#98218=AXIS2_PLACEMENT_3D('',#153186,#113551,#113552);
#98219=AXIS2_PLACEMENT_3D('',#153188,#113553,#113554);
#98220=AXIS2_PLACEMENT_3D('',#153190,#113555,#113556);
#98221=AXIS2_PLACEMENT_3D('',#153191,#113557,#113558);
#98222=AXIS2_PLACEMENT_3D('',#153193,#113559,#113560);
#98223=AXIS2_PLACEMENT_3D('',#153195,#113561,#113562);
#98224=AXIS2_PLACEMENT_3D('',#153196,#113563,#113564);
#98225=AXIS2_PLACEMENT_3D('',#153198,#113565,#113566);
#98226=AXIS2_PLACEMENT_3D('',#153200,#113567,#113568);
#98227=AXIS2_PLACEMENT_3D('',#153201,#113569,#113570);
#98228=AXIS2_PLACEMENT_3D('',#153203,#113571,#113572);
#98229=AXIS2_PLACEMENT_3D('',#153205,#113573,#113574);
#98230=AXIS2_PLACEMENT_3D('',#153206,#113575,#113576);
#98231=AXIS2_PLACEMENT_3D('',#153208,#113577,#113578);
#98232=AXIS2_PLACEMENT_3D('',#153210,#113579,#113580);
#98233=AXIS2_PLACEMENT_3D('',#153211,#113581,#113582);
#98234=AXIS2_PLACEMENT_3D('',#153213,#113583,#113584);
#98235=AXIS2_PLACEMENT_3D('',#153214,#113585,#113586);
#98236=AXIS2_PLACEMENT_3D('',#153216,#113587,#113588);
#98237=AXIS2_PLACEMENT_3D('',#153217,#113589,#113590);
#98238=AXIS2_PLACEMENT_3D('',#153219,#113591,#113592);
#98239=AXIS2_PLACEMENT_3D('',#153221,#113593,#113594);
#98240=AXIS2_PLACEMENT_3D('',#153222,#113595,#113596);
#98241=AXIS2_PLACEMENT_3D('',#153224,#113597,#113598);
#98242=AXIS2_PLACEMENT_3D('',#153226,#113599,#113600);
#98243=AXIS2_PLACEMENT_3D('',#153227,#113601,#113602);
#98244=AXIS2_PLACEMENT_3D('',#153229,#113603,#113604);
#98245=AXIS2_PLACEMENT_3D('',#153231,#113605,#113606);
#98246=AXIS2_PLACEMENT_3D('',#153232,#113607,#113608);
#98247=AXIS2_PLACEMENT_3D('',#153234,#113609,#113610);
#98248=AXIS2_PLACEMENT_3D('',#153236,#113611,#113612);
#98249=AXIS2_PLACEMENT_3D('',#153237,#113613,#113614);
#98250=AXIS2_PLACEMENT_3D('',#153239,#113615,#113616);
#98251=AXIS2_PLACEMENT_3D('',#153241,#113617,#113618);
#98252=AXIS2_PLACEMENT_3D('',#153242,#113619,#113620);
#98253=AXIS2_PLACEMENT_3D('',#153244,#113621,#113622);
#98254=AXIS2_PLACEMENT_3D('',#153246,#113623,#113624);
#98255=AXIS2_PLACEMENT_3D('',#153247,#113625,#113626);
#98256=AXIS2_PLACEMENT_3D('',#153249,#113627,#113628);
#98257=AXIS2_PLACEMENT_3D('',#153250,#113629,#113630);
#98258=AXIS2_PLACEMENT_3D('',#153251,#113631,#113632);
#98259=AXIS2_PLACEMENT_3D('',#153254,#113635,#113636);
#98260=AXIS2_PLACEMENT_3D('',#153256,#113638,#113639);
#98261=AXIS2_PLACEMENT_3D('',#153258,#113641,#113642);
#98262=AXIS2_PLACEMENT_3D('',#153259,#113643,#113644);
#98263=AXIS2_PLACEMENT_3D('',#153261,#113646,#113647);
#98264=AXIS2_PLACEMENT_3D('',#153263,#113649,#113650);
#98265=AXIS2_PLACEMENT_3D('',#153264,#113651,#113652);
#98266=AXIS2_PLACEMENT_3D('',#153266,#113654,#113655);
#98267=AXIS2_PLACEMENT_3D('',#153268,#113657,#113658);
#98268=AXIS2_PLACEMENT_3D('',#153269,#113659,#113660);
#98269=AXIS2_PLACEMENT_3D('',#153271,#113662,#113663);
#98270=AXIS2_PLACEMENT_3D('',#153273,#113665,#113666);
#98271=AXIS2_PLACEMENT_3D('',#153274,#113667,#113668);
#98272=AXIS2_PLACEMENT_3D('',#153276,#113670,#113671);
#98273=AXIS2_PLACEMENT_3D('',#153278,#113673,#113674);
#98274=AXIS2_PLACEMENT_3D('',#153279,#113675,#113676);
#98275=AXIS2_PLACEMENT_3D('',#153281,#113678,#113679);
#98276=AXIS2_PLACEMENT_3D('',#153283,#113681,#113682);
#98277=AXIS2_PLACEMENT_3D('',#153284,#113683,#113684);
#98278=AXIS2_PLACEMENT_3D('',#153286,#113686,#113687);
#98279=AXIS2_PLACEMENT_3D('',#153288,#113689,#113690);
#98280=AXIS2_PLACEMENT_3D('',#153289,#113691,#113692);
#98281=AXIS2_PLACEMENT_3D('',#153291,#113694,#113695);
#98282=AXIS2_PLACEMENT_3D('',#153293,#113697,#113698);
#98283=AXIS2_PLACEMENT_3D('',#153294,#113699,#113700);
#98284=AXIS2_PLACEMENT_3D('',#153296,#113702,#113703);
#98285=AXIS2_PLACEMENT_3D('',#153298,#113705,#113706);
#98286=AXIS2_PLACEMENT_3D('',#153299,#113707,#113708);
#98287=AXIS2_PLACEMENT_3D('',#153301,#113710,#113711);
#98288=AXIS2_PLACEMENT_3D('',#153303,#113713,#113714);
#98289=AXIS2_PLACEMENT_3D('',#153304,#113715,#113716);
#98290=AXIS2_PLACEMENT_3D('',#153306,#113718,#113719);
#98291=AXIS2_PLACEMENT_3D('',#153308,#113721,#113722);
#98292=AXIS2_PLACEMENT_3D('',#153309,#113723,#113724);
#98293=AXIS2_PLACEMENT_3D('',#153311,#113726,#113727);
#98294=AXIS2_PLACEMENT_3D('',#153313,#113729,#113730);
#98295=AXIS2_PLACEMENT_3D('',#153314,#113731,#113732);
#98296=AXIS2_PLACEMENT_3D('',#153316,#113734,#113735);
#98297=AXIS2_PLACEMENT_3D('',#153318,#113737,#113738);
#98298=AXIS2_PLACEMENT_3D('',#153319,#113739,#113740);
#98299=AXIS2_PLACEMENT_3D('',#153321,#113742,#113743);
#98300=AXIS2_PLACEMENT_3D('',#153323,#113745,#113746);
#98301=AXIS2_PLACEMENT_3D('',#153324,#113747,#113748);
#98302=AXIS2_PLACEMENT_3D('',#153326,#113750,#113751);
#98303=AXIS2_PLACEMENT_3D('',#153328,#113753,#113754);
#98304=AXIS2_PLACEMENT_3D('',#153329,#113755,#113756);
#98305=AXIS2_PLACEMENT_3D('',#153331,#113758,#113759);
#98306=AXIS2_PLACEMENT_3D('',#153333,#113761,#113762);
#98307=AXIS2_PLACEMENT_3D('',#153334,#113763,#113764);
#98308=AXIS2_PLACEMENT_3D('',#153336,#113766,#113767);
#98309=AXIS2_PLACEMENT_3D('',#153338,#113769,#113770);
#98310=AXIS2_PLACEMENT_3D('',#153339,#113771,#113772);
#98311=AXIS2_PLACEMENT_3D('',#153341,#113774,#113775);
#98312=AXIS2_PLACEMENT_3D('',#153343,#113777,#113778);
#98313=AXIS2_PLACEMENT_3D('',#153344,#113779,#113780);
#98314=AXIS2_PLACEMENT_3D('',#153346,#113782,#113783);
#98315=AXIS2_PLACEMENT_3D('',#153348,#113785,#113786);
#98316=AXIS2_PLACEMENT_3D('',#153349,#113787,#113788);
#98317=AXIS2_PLACEMENT_3D('',#153351,#113790,#113791);
#98318=AXIS2_PLACEMENT_3D('',#153353,#113793,#113794);
#98319=AXIS2_PLACEMENT_3D('',#153354,#113795,#113796);
#98320=AXIS2_PLACEMENT_3D('',#153356,#113798,#113799);
#98321=AXIS2_PLACEMENT_3D('',#153358,#113801,#113802);
#98322=AXIS2_PLACEMENT_3D('',#153359,#113803,#113804);
#98323=AXIS2_PLACEMENT_3D('',#153361,#113806,#113807);
#98324=AXIS2_PLACEMENT_3D('',#153363,#113809,#113810);
#98325=AXIS2_PLACEMENT_3D('',#153364,#113811,#113812);
#98326=AXIS2_PLACEMENT_3D('',#153366,#113814,#113815);
#98327=AXIS2_PLACEMENT_3D('',#153368,#113817,#113818);
#98328=AXIS2_PLACEMENT_3D('',#153369,#113819,#113820);
#98329=AXIS2_PLACEMENT_3D('',#153371,#113822,#113823);
#98330=AXIS2_PLACEMENT_3D('',#153373,#113825,#113826);
#98331=AXIS2_PLACEMENT_3D('',#153374,#113827,#113828);
#98332=AXIS2_PLACEMENT_3D('',#153376,#113830,#113831);
#98333=AXIS2_PLACEMENT_3D('',#153378,#113833,#113834);
#98334=AXIS2_PLACEMENT_3D('',#153379,#113835,#113836);
#98335=AXIS2_PLACEMENT_3D('',#153381,#113838,#113839);
#98336=AXIS2_PLACEMENT_3D('',#153382,#113840,#113841);
#98337=AXIS2_PLACEMENT_3D('',#153384,#113843,#113844);
#98338=AXIS2_PLACEMENT_3D('',#153385,#113845,#113846);
#98339=AXIS2_PLACEMENT_3D('',#153387,#113848,#113849);
#98340=AXIS2_PLACEMENT_3D('',#153389,#113851,#113852);
#98341=AXIS2_PLACEMENT_3D('',#153390,#113853,#113854);
#98342=AXIS2_PLACEMENT_3D('',#153392,#113856,#113857);
#98343=AXIS2_PLACEMENT_3D('',#153394,#113859,#113860);
#98344=AXIS2_PLACEMENT_3D('',#153395,#113861,#113862);
#98345=AXIS2_PLACEMENT_3D('',#153397,#113864,#113865);
#98346=AXIS2_PLACEMENT_3D('',#153399,#113867,#113868);
#98347=AXIS2_PLACEMENT_3D('',#153400,#113869,#113870);
#98348=AXIS2_PLACEMENT_3D('',#153402,#113872,#113873);
#98349=AXIS2_PLACEMENT_3D('',#153404,#113875,#113876);
#98350=AXIS2_PLACEMENT_3D('',#153405,#113877,#113878);
#98351=AXIS2_PLACEMENT_3D('',#153407,#113880,#113881);
#98352=AXIS2_PLACEMENT_3D('',#153408,#113882,#113883);
#98353=AXIS2_PLACEMENT_3D('',#153410,#113885,#113886);
#98354=AXIS2_PLACEMENT_3D('',#153411,#113887,#113888);
#98355=AXIS2_PLACEMENT_3D('',#153413,#113890,#113891);
#98356=AXIS2_PLACEMENT_3D('',#153415,#113893,#113894);
#98357=AXIS2_PLACEMENT_3D('',#153416,#113895,#113896);
#98358=AXIS2_PLACEMENT_3D('',#153418,#113898,#113899);
#98359=AXIS2_PLACEMENT_3D('',#153420,#113901,#113902);
#98360=AXIS2_PLACEMENT_3D('',#153421,#113903,#113904);
#98361=AXIS2_PLACEMENT_3D('',#153423,#113906,#113907);
#98362=AXIS2_PLACEMENT_3D('',#153425,#113909,#113910);
#98363=AXIS2_PLACEMENT_3D('',#153426,#113911,#113912);
#98364=AXIS2_PLACEMENT_3D('',#153428,#113914,#113915);
#98365=AXIS2_PLACEMENT_3D('',#153430,#113917,#113918);
#98366=AXIS2_PLACEMENT_3D('',#153431,#113919,#113920);
#98367=AXIS2_PLACEMENT_3D('',#153432,#113921,#113922);
#98368=AXIS2_PLACEMENT_3D('',#153433,#113923,#113924);
#98369=AXIS2_PLACEMENT_3D('',#153434,#113925,#113926);
#98370=AXIS2_PLACEMENT_3D('',#153435,#113927,#113928);
#98371=AXIS2_PLACEMENT_3D('',#153441,#113932,#113933);
#98372=AXIS2_PLACEMENT_3D('',#153445,#113935,#113936);
#98373=AXIS2_PLACEMENT_3D('',#153446,#113937,#113938);
#98374=AXIS2_PLACEMENT_3D('',#153447,#113939,#113940);
#98375=AXIS2_PLACEMENT_3D('',#153451,#113942,#113943);
#98376=AXIS2_PLACEMENT_3D('',#153452,#113944,#113945);
#98377=AXIS2_PLACEMENT_3D('',#153453,#113946,#113947);
#98378=AXIS2_PLACEMENT_3D('',#153457,#113949,#113950);
#98379=AXIS2_PLACEMENT_3D('',#153458,#113951,#113952);
#98380=AXIS2_PLACEMENT_3D('',#153459,#113953,#113954);
#98381=AXIS2_PLACEMENT_3D('',#153464,#113958,#113959);
#98382=AXIS2_PLACEMENT_3D('',#153467,#113961,#113962);
#98383=AXIS2_PLACEMENT_3D('',#153468,#113963,#113964);
#98384=AXIS2_PLACEMENT_3D('',#153469,#113965,#113966);
#98385=AXIS2_PLACEMENT_3D('',#153470,#113967,#113968);
#98386=AXIS2_PLACEMENT_3D('',#153471,#113969,#113970);
#98387=AXIS2_PLACEMENT_3D('',#153472,#113971,#113972);
#98388=AXIS2_PLACEMENT_3D('',#153477,#113974,#113975);
#98389=AXIS2_PLACEMENT_3D('',#153480,#113977,#113978);
#98390=AXIS2_PLACEMENT_3D('',#153481,#113979,#113980);
#98391=AXIS2_PLACEMENT_3D('',#153484,#113983,#113984);
#98392=AXIS2_PLACEMENT_3D('',#153487,#113986,#113987);
#98393=AXIS2_PLACEMENT_3D('',#153488,#113988,#113989);
#98394=AXIS2_PLACEMENT_3D('',#153489,#113990,#113991);
#98395=AXIS2_PLACEMENT_3D('',#153492,#113993,#113994);
#98396=AXIS2_PLACEMENT_3D('',#153493,#113995,#113996);
#98397=AXIS2_PLACEMENT_3D('',#153499,#114000,#114001);
#98398=AXIS2_PLACEMENT_3D('',#153503,#114003,#114004);
#98399=AXIS2_PLACEMENT_3D('',#153504,#114005,#114006);
#98400=AXIS2_PLACEMENT_3D('',#153505,#114007,#114008);
#98401=AXIS2_PLACEMENT_3D('',#153506,#114009,#114010);
#98402=AXIS2_PLACEMENT_3D('',#153507,#114011,#114012);
#98403=AXIS2_PLACEMENT_3D('',#153508,#114013,#114014);
#98404=AXIS2_PLACEMENT_3D('',#153509,#114015,#114016);
#98405=AXIS2_PLACEMENT_3D('',#153510,#114017,#114018);
#98406=AXIS2_PLACEMENT_3D('',#153511,#114019,#114020);
#98407=AXIS2_PLACEMENT_3D('',#153512,#114021,#114022);
#98408=AXIS2_PLACEMENT_3D('',#153513,#114023,#114024);
#98409=AXIS2_PLACEMENT_3D('',#153514,#114025,#114026);
#98410=AXIS2_PLACEMENT_3D('',#153515,#114027,#114028);
#98411=AXIS2_PLACEMENT_3D('',#153516,#114029,#114030);
#98412=AXIS2_PLACEMENT_3D('',#153517,#114031,#114032);
#98413=AXIS2_PLACEMENT_3D('',#153518,#114033,#114034);
#98414=AXIS2_PLACEMENT_3D('',#153519,#114035,#114036);
#98415=AXIS2_PLACEMENT_3D('',#153520,#114037,#114038);
#98416=AXIS2_PLACEMENT_3D('',#153521,#114039,#114040);
#98417=AXIS2_PLACEMENT_3D('',#153522,#114041,#114042);
#98418=AXIS2_PLACEMENT_3D('',#153523,#114043,#114044);
#98419=AXIS2_PLACEMENT_3D('',#153524,#114045,#114046);
#98420=AXIS2_PLACEMENT_3D('',#153525,#114047,#114048);
#98421=AXIS2_PLACEMENT_3D('',#153526,#114049,#114050);
#98422=AXIS2_PLACEMENT_3D('',#153527,#114051,#114052);
#98423=AXIS2_PLACEMENT_3D('',#153528,#114053,#114054);
#98424=AXIS2_PLACEMENT_3D('',#153529,#114055,#114056);
#98425=AXIS2_PLACEMENT_3D('',#153530,#114057,#114058);
#98426=AXIS2_PLACEMENT_3D('',#153531,#114059,#114060);
#98427=AXIS2_PLACEMENT_3D('',#153532,#114061,#114062);
#98428=AXIS2_PLACEMENT_3D('',#153533,#114063,#114064);
#98429=AXIS2_PLACEMENT_3D('',#153534,#114065,#114066);
#98430=AXIS2_PLACEMENT_3D('',#153535,#114067,#114068);
#98431=AXIS2_PLACEMENT_3D('',#153536,#114069,#114070);
#111496=DIRECTION('axis',(0.,0.,1.));
#111497=DIRECTION('refdir',(1.,0.,0.));
#111498=DIRECTION('center_axis',(-3.85185988875507E-34,1.,0.));
#111499=DIRECTION('ref_axis',(1.,0.,0.));
#111500=DIRECTION('center_axis',(-3.85185988875507E-34,1.,0.));
#111501=DIRECTION('ref_axis',(0.,0.,1.));
#111502=DIRECTION('center_axis',(-3.85185988875507E-34,1.,0.));
#111503=DIRECTION('ref_axis',(0.,0.,1.));
#111504=DIRECTION('center_axis',(-3.85185988875507E-34,1.,0.));
#111505=DIRECTION('ref_axis',(1.,0.,0.));
#111506=DIRECTION('center_axis',(-3.85185988875507E-34,1.,0.));
#111507=DIRECTION('ref_axis',(0.,0.,1.));
#111508=DIRECTION('center_axis',(-3.85185988875507E-34,1.,0.));
#111509=DIRECTION('ref_axis',(0.,0.,1.));
#111510=DIRECTION('center_axis',(-3.85185988875507E-34,1.,0.));
#111511=DIRECTION('ref_axis',(1.,0.,0.));
#111512=DIRECTION('center_axis',(-3.85185988875507E-34,1.,0.));
#111513=DIRECTION('ref_axis',(0.,0.,1.));
#111514=DIRECTION('center_axis',(-3.85185988875507E-34,1.,0.));
#111515=DIRECTION('ref_axis',(0.,0.,1.));
#111516=DIRECTION('center_axis',(-3.85185988875507E-34,1.,0.));
#111517=DIRECTION('ref_axis',(1.,0.,0.));
#111518=DIRECTION('center_axis',(-3.85185988875507E-34,1.,0.));
#111519=DIRECTION('ref_axis',(0.,0.,1.));
#111520=DIRECTION('center_axis',(-3.85185988875507E-34,1.,0.));
#111521=DIRECTION('ref_axis',(0.,0.,1.));
#111522=DIRECTION('center_axis',(-3.85185988875507E-34,1.,0.));
#111523=DIRECTION('ref_axis',(1.,0.,0.));
#111524=DIRECTION('center_axis',(-3.85185988875507E-34,1.,0.));
#111525=DIRECTION('ref_axis',(0.,0.,1.));
#111526=DIRECTION('center_axis',(-3.85185988875507E-34,1.,0.));
#111527=DIRECTION('ref_axis',(0.,0.,1.));
#111528=DIRECTION('center_axis',(-3.85185988875507E-34,1.,0.));
#111529=DIRECTION('ref_axis',(1.,0.,0.));
#111530=DIRECTION('center_axis',(-3.85185988875507E-34,1.,0.));
#111531=DIRECTION('ref_axis',(0.,0.,1.));
#111532=DIRECTION('center_axis',(-3.85185988875507E-34,1.,0.));
#111533=DIRECTION('ref_axis',(0.,0.,1.));
#111534=DIRECTION('center_axis',(-3.85185988875507E-34,1.,0.));
#111535=DIRECTION('ref_axis',(1.,0.,0.));
#111536=DIRECTION('center_axis',(-3.85185988875507E-34,1.,0.));
#111537=DIRECTION('ref_axis',(0.,0.,1.));
#111538=DIRECTION('center_axis',(-3.85185988875507E-34,1.,0.));
#111539=DIRECTION('ref_axis',(0.,0.,1.));
#111540=DIRECTION('center_axis',(-3.85185988875507E-34,1.,0.));
#111541=DIRECTION('ref_axis',(1.,0.,0.));
#111542=DIRECTION('center_axis',(-3.85185988875507E-34,1.,0.));
#111543=DIRECTION('ref_axis',(0.,0.,1.));
#111544=DIRECTION('center_axis',(-3.85185988875507E-34,1.,0.));
#111545=DIRECTION('ref_axis',(0.,0.,1.));
#111546=DIRECTION('center_axis',(-3.85185988875507E-34,1.,0.));
#111547=DIRECTION('ref_axis',(1.,0.,0.));
#111548=DIRECTION('center_axis',(-3.85185988875507E-34,1.,0.));
#111549=DIRECTION('ref_axis',(0.,0.,1.));
#111550=DIRECTION('center_axis',(-3.85185988875507E-34,1.,0.));
#111551=DIRECTION('ref_axis',(0.,0.,1.));
#111552=DIRECTION('center_axis',(-3.85185988875507E-34,1.,0.));
#111553=DIRECTION('ref_axis',(1.,0.,0.));
#111554=DIRECTION('center_axis',(-3.85185988875507E-34,1.,0.));
#111555=DIRECTION('ref_axis',(0.,0.,1.));
#111556=DIRECTION('center_axis',(-3.85185988875507E-34,1.,0.));
#111557=DIRECTION('ref_axis',(0.,0.,1.));
#111558=DIRECTION('center_axis',(-3.85185988875507E-34,1.,0.));
#111559=DIRECTION('ref_axis',(1.,0.,0.));
#111560=DIRECTION('center_axis',(-3.85185988875507E-34,1.,0.));
#111561=DIRECTION('ref_axis',(0.,0.,1.));
#111562=DIRECTION('center_axis',(-3.85185988875507E-34,1.,0.));
#111563=DIRECTION('ref_axis',(0.,0.,1.));
#111564=DIRECTION('center_axis',(-3.85185988875507E-34,1.,0.));
#111565=DIRECTION('ref_axis',(1.,0.,0.));
#111566=DIRECTION('center_axis',(-3.85185988875507E-34,1.,0.));
#111567=DIRECTION('ref_axis',(0.,0.,1.));
#111568=DIRECTION('center_axis',(-3.85185988875507E-34,1.,0.));
#111569=DIRECTION('ref_axis',(0.,0.,1.));
#111570=DIRECTION('center_axis',(-3.85185988875507E-34,1.,0.));
#111571=DIRECTION('ref_axis',(1.,0.,0.));
#111572=DIRECTION('center_axis',(-3.85185988875507E-34,1.,0.));
#111573=DIRECTION('ref_axis',(0.,0.,1.));
#111574=DIRECTION('center_axis',(-3.85185988875507E-34,1.,0.));
#111575=DIRECTION('ref_axis',(0.,0.,1.));
#111576=DIRECTION('center_axis',(-3.85185988875507E-34,1.,0.));
#111577=DIRECTION('ref_axis',(1.,0.,0.));
#111578=DIRECTION('center_axis',(-3.85185988875507E-34,1.,0.));
#111579=DIRECTION('ref_axis',(0.,0.,1.));
#111580=DIRECTION('center_axis',(-3.85185988875507E-34,1.,0.));
#111581=DIRECTION('ref_axis',(0.,0.,1.));
#111582=DIRECTION('center_axis',(-3.85185988875507E-34,1.,0.));
#111583=DIRECTION('ref_axis',(1.,0.,0.));
#111584=DIRECTION('center_axis',(-3.85185988875507E-34,1.,0.));
#111585=DIRECTION('ref_axis',(0.,0.,1.));
#111586=DIRECTION('center_axis',(-3.85185988875507E-34,1.,0.));
#111587=DIRECTION('ref_axis',(0.,0.,1.));
#111588=DIRECTION('center_axis',(-3.85185988875507E-34,1.,0.));
#111589=DIRECTION('ref_axis',(1.,0.,0.));
#111590=DIRECTION('center_axis',(-3.85185988875507E-34,1.,0.));
#111591=DIRECTION('ref_axis',(0.,0.,1.));
#111592=DIRECTION('center_axis',(-3.85185988875507E-34,1.,0.));
#111593=DIRECTION('ref_axis',(0.,0.,1.));
#111594=DIRECTION('center_axis',(-3.85185988875507E-34,1.,0.));
#111595=DIRECTION('ref_axis',(1.,0.,0.));
#111596=DIRECTION('center_axis',(-3.85185988875507E-34,1.,0.));
#111597=DIRECTION('ref_axis',(0.,0.,1.));
#111598=DIRECTION('center_axis',(-3.85185988875507E-34,1.,0.));
#111599=DIRECTION('ref_axis',(0.,0.,1.));
#111600=DIRECTION('center_axis',(-3.85185988875507E-34,1.,0.));
#111601=DIRECTION('ref_axis',(1.,0.,0.));
#111602=DIRECTION('center_axis',(-3.85185988875507E-34,1.,0.));
#111603=DIRECTION('ref_axis',(0.,0.,1.));
#111604=DIRECTION('center_axis',(-3.85185988875507E-34,1.,0.));
#111605=DIRECTION('ref_axis',(0.,0.,1.));
#111606=DIRECTION('center_axis',(-3.85185988875507E-34,1.,0.));
#111607=DIRECTION('ref_axis',(1.,0.,0.));
#111608=DIRECTION('center_axis',(-3.85185988875507E-34,1.,0.));
#111609=DIRECTION('ref_axis',(0.,0.,1.));
#111610=DIRECTION('center_axis',(-3.85185988875507E-34,1.,0.));
#111611=DIRECTION('ref_axis',(0.,0.,1.));
#111612=DIRECTION('center_axis',(-3.85185988875507E-34,1.,0.));
#111613=DIRECTION('ref_axis',(1.,0.,0.));
#111614=DIRECTION('center_axis',(-3.85185988875507E-34,1.,0.));
#111615=DIRECTION('ref_axis',(0.,0.,1.));
#111616=DIRECTION('center_axis',(-3.85185988875507E-34,1.,0.));
#111617=DIRECTION('ref_axis',(0.,0.,1.));
#111618=DIRECTION('center_axis',(-3.85185988875507E-34,1.,0.));
#111619=DIRECTION('ref_axis',(1.,0.,0.));
#111620=DIRECTION('center_axis',(-3.85185988875507E-34,1.,0.));
#111621=DIRECTION('ref_axis',(0.,0.,1.));
#111622=DIRECTION('center_axis',(-3.85185988875507E-34,1.,0.));
#111623=DIRECTION('ref_axis',(0.,0.,1.));
#111624=DIRECTION('center_axis',(-3.85185988875507E-34,1.,0.));
#111625=DIRECTION('ref_axis',(1.,0.,0.));
#111626=DIRECTION('center_axis',(-3.85185988875507E-34,1.,0.));
#111627=DIRECTION('ref_axis',(0.,0.,1.));
#111628=DIRECTION('center_axis',(-3.85185988875507E-34,1.,0.));
#111629=DIRECTION('ref_axis',(0.,0.,1.));
#111630=DIRECTION('center_axis',(-3.85185988875507E-34,1.,0.));
#111631=DIRECTION('ref_axis',(1.,0.,0.));
#111632=DIRECTION('center_axis',(-3.85185988875507E-34,1.,0.));
#111633=DIRECTION('ref_axis',(0.,0.,1.));
#111634=DIRECTION('center_axis',(-3.85185988875507E-34,1.,0.));
#111635=DIRECTION('ref_axis',(0.,0.,1.));
#111636=DIRECTION('center_axis',(-3.85185988875507E-34,1.,0.));
#111637=DIRECTION('ref_axis',(1.,0.,0.));
#111638=DIRECTION('center_axis',(-3.85185988875507E-34,1.,0.));
#111639=DIRECTION('ref_axis',(0.,0.,1.));
#111640=DIRECTION('center_axis',(-3.85185988875507E-34,1.,0.));
#111641=DIRECTION('ref_axis',(0.,0.,1.));
#111642=DIRECTION('center_axis',(-3.85185988875507E-34,1.,0.));
#111643=DIRECTION('ref_axis',(1.,0.,0.));
#111644=DIRECTION('center_axis',(-3.85185988875507E-34,1.,0.));
#111645=DIRECTION('ref_axis',(0.,0.,1.));
#111646=DIRECTION('center_axis',(-3.85185988875507E-34,1.,0.));
#111647=DIRECTION('ref_axis',(0.,0.,1.));
#111648=DIRECTION('center_axis',(-3.85185988875507E-34,1.,0.));
#111649=DIRECTION('ref_axis',(1.,0.,0.));
#111650=DIRECTION('center_axis',(-3.85185988875507E-34,1.,0.));
#111651=DIRECTION('ref_axis',(0.,0.,1.));
#111652=DIRECTION('center_axis',(-3.85185988875507E-34,1.,0.));
#111653=DIRECTION('ref_axis',(0.,0.,1.));
#111654=DIRECTION('center_axis',(-3.85185988875507E-34,1.,0.));
#111655=DIRECTION('ref_axis',(1.,0.,0.));
#111656=DIRECTION('center_axis',(-3.85185988875507E-34,1.,0.));
#111657=DIRECTION('ref_axis',(0.,0.,1.));
#111658=DIRECTION('center_axis',(-3.85185988875507E-34,1.,0.));
#111659=DIRECTION('ref_axis',(0.,0.,1.));
#111660=DIRECTION('center_axis',(-3.85185988875507E-34,1.,0.));
#111661=DIRECTION('ref_axis',(1.,0.,0.));
#111662=DIRECTION('center_axis',(-3.85185988875507E-34,1.,0.));
#111663=DIRECTION('ref_axis',(0.,0.,1.));
#111664=DIRECTION('center_axis',(-3.85185988875507E-34,1.,0.));
#111665=DIRECTION('ref_axis',(0.,0.,1.));
#111666=DIRECTION('center_axis',(-3.85185988875507E-34,1.,0.));
#111667=DIRECTION('ref_axis',(1.,0.,0.));
#111668=DIRECTION('center_axis',(-3.85185988875507E-34,1.,0.));
#111669=DIRECTION('ref_axis',(0.,0.,1.));
#111670=DIRECTION('center_axis',(-3.85185988875507E-34,1.,0.));
#111671=DIRECTION('ref_axis',(0.,0.,1.));
#111672=DIRECTION('center_axis',(-3.85185988875507E-34,1.,0.));
#111673=DIRECTION('ref_axis',(1.,0.,0.));
#111674=DIRECTION('center_axis',(-3.85185988875507E-34,1.,0.));
#111675=DIRECTION('ref_axis',(0.,0.,1.));
#111676=DIRECTION('center_axis',(-3.85185988875507E-34,1.,0.));
#111677=DIRECTION('ref_axis',(0.,0.,1.));
#111678=DIRECTION('center_axis',(-3.85185988875507E-34,1.,0.));
#111679=DIRECTION('ref_axis',(1.,0.,0.));
#111680=DIRECTION('center_axis',(-3.85185988875507E-34,1.,0.));
#111681=DIRECTION('ref_axis',(0.,0.,1.));
#111682=DIRECTION('center_axis',(-3.85185988875507E-34,1.,0.));
#111683=DIRECTION('ref_axis',(0.,0.,1.));
#111684=DIRECTION('center_axis',(-3.85185988875507E-34,1.,0.));
#111685=DIRECTION('ref_axis',(1.,0.,0.));
#111686=DIRECTION('center_axis',(-3.85185988875507E-34,1.,0.));
#111687=DIRECTION('ref_axis',(0.,0.,1.));
#111688=DIRECTION('center_axis',(-3.85185988875507E-34,1.,0.));
#111689=DIRECTION('ref_axis',(0.,0.,1.));
#111690=DIRECTION('center_axis',(-3.85185988875507E-34,1.,0.));
#111691=DIRECTION('ref_axis',(1.,0.,0.));
#111692=DIRECTION('center_axis',(-3.85185988875507E-34,1.,0.));
#111693=DIRECTION('ref_axis',(0.,0.,1.));
#111694=DIRECTION('center_axis',(-3.85185988875507E-34,1.,0.));
#111695=DIRECTION('ref_axis',(0.,0.,1.));
#111696=DIRECTION('center_axis',(-3.85185988875507E-34,1.,0.));
#111697=DIRECTION('ref_axis',(1.,0.,0.));
#111698=DIRECTION('center_axis',(-3.85185988875507E-34,1.,0.));
#111699=DIRECTION('ref_axis',(0.,0.,1.));
#111700=DIRECTION('center_axis',(-3.85185988875507E-34,1.,0.));
#111701=DIRECTION('ref_axis',(0.,0.,1.));
#111702=DIRECTION('center_axis',(-3.85185988875507E-34,1.,0.));
#111703=DIRECTION('ref_axis',(1.,0.,0.));
#111704=DIRECTION('center_axis',(-3.85185988875507E-34,1.,0.));
#111705=DIRECTION('ref_axis',(0.,0.,1.));
#111706=DIRECTION('center_axis',(-3.85185988875507E-34,1.,0.));
#111707=DIRECTION('ref_axis',(0.,0.,1.));
#111708=DIRECTION('center_axis',(-3.85185988875507E-34,1.,0.));
#111709=DIRECTION('ref_axis',(1.,0.,0.));
#111710=DIRECTION('center_axis',(-3.85185988875507E-34,1.,0.));
#111711=DIRECTION('ref_axis',(0.,0.,1.));
#111712=DIRECTION('center_axis',(-3.85185988875507E-34,1.,0.));
#111713=DIRECTION('ref_axis',(0.,0.,1.));
#111714=DIRECTION('center_axis',(-3.85185988875507E-34,1.,0.));
#111715=DIRECTION('ref_axis',(1.,0.,0.));
#111716=DIRECTION('center_axis',(-3.85185988875507E-34,1.,0.));
#111717=DIRECTION('ref_axis',(0.,0.,1.));
#111718=DIRECTION('center_axis',(-3.85185988875507E-34,1.,0.));
#111719=DIRECTION('ref_axis',(0.,0.,1.));
#111720=DIRECTION('center_axis',(-3.85185988875507E-34,1.,0.));
#111721=DIRECTION('ref_axis',(1.,0.,0.));
#111722=DIRECTION('center_axis',(-3.85185988875507E-34,1.,0.));
#111723=DIRECTION('ref_axis',(0.,0.,1.));
#111724=DIRECTION('center_axis',(-3.85185988875507E-34,1.,0.));
#111725=DIRECTION('ref_axis',(0.,0.,1.));
#111726=DIRECTION('center_axis',(-3.85185988875507E-34,1.,0.));
#111727=DIRECTION('ref_axis',(1.,0.,0.));
#111728=DIRECTION('center_axis',(-3.85185988875507E-34,1.,0.));
#111729=DIRECTION('ref_axis',(0.,0.,1.));
#111730=DIRECTION('center_axis',(-3.85185988875507E-34,1.,0.));
#111731=DIRECTION('ref_axis',(0.,0.,1.));
#111732=DIRECTION('center_axis',(-3.85185988875507E-34,1.,0.));
#111733=DIRECTION('ref_axis',(1.,0.,0.));
#111734=DIRECTION('center_axis',(-3.85185988875507E-34,1.,0.));
#111735=DIRECTION('ref_axis',(0.,0.,1.));
#111736=DIRECTION('center_axis',(-3.85185988875507E-34,1.,0.));
#111737=DIRECTION('ref_axis',(0.,0.,1.));
#111738=DIRECTION('center_axis',(-3.85185988875507E-34,1.,0.));
#111739=DIRECTION('ref_axis',(1.,0.,0.));
#111740=DIRECTION('center_axis',(-3.85185988875507E-34,1.,0.));
#111741=DIRECTION('ref_axis',(0.,0.,1.));
#111742=DIRECTION('center_axis',(-3.85185988875507E-34,1.,0.));
#111743=DIRECTION('ref_axis',(0.,0.,1.));
#111744=DIRECTION('center_axis',(-3.85185988875507E-34,1.,0.));
#111745=DIRECTION('ref_axis',(1.,0.,0.));
#111746=DIRECTION('center_axis',(-3.85185988875507E-34,1.,0.));
#111747=DIRECTION('ref_axis',(0.,0.,1.));
#111748=DIRECTION('center_axis',(-3.85185988875507E-34,1.,0.));
#111749=DIRECTION('ref_axis',(0.,0.,1.));
#111750=DIRECTION('center_axis',(-3.85185988875507E-34,1.,0.));
#111751=DIRECTION('ref_axis',(1.,0.,0.));
#111752=DIRECTION('center_axis',(-3.85185988875507E-34,1.,0.));
#111753=DIRECTION('ref_axis',(0.,0.,1.));
#111754=DIRECTION('center_axis',(-3.85185988875507E-34,1.,0.));
#111755=DIRECTION('ref_axis',(0.,0.,1.));
#111756=DIRECTION('center_axis',(-3.85185988875507E-34,1.,0.));
#111757=DIRECTION('ref_axis',(1.,0.,0.));
#111758=DIRECTION('center_axis',(-3.85185988875507E-34,1.,0.));
#111759=DIRECTION('ref_axis',(0.,0.,1.));
#111760=DIRECTION('center_axis',(-3.85185988875507E-34,1.,0.));
#111761=DIRECTION('ref_axis',(0.,0.,1.));
#111762=DIRECTION('center_axis',(-3.85185988875507E-34,1.,0.));
#111763=DIRECTION('ref_axis',(1.,0.,0.));
#111764=DIRECTION('center_axis',(-3.85185988875507E-34,1.,0.));
#111765=DIRECTION('ref_axis',(0.,0.,1.));
#111766=DIRECTION('center_axis',(-3.85185988875507E-34,1.,0.));
#111767=DIRECTION('ref_axis',(0.,0.,1.));
#111768=DIRECTION('center_axis',(-3.85185988875507E-34,1.,0.));
#111769=DIRECTION('ref_axis',(1.,0.,0.));
#111770=DIRECTION('center_axis',(-3.85185988875507E-34,1.,0.));
#111771=DIRECTION('ref_axis',(0.,0.,1.));
#111772=DIRECTION('center_axis',(-3.85185988875507E-34,1.,0.));
#111773=DIRECTION('ref_axis',(0.,0.,1.));
#111774=DIRECTION('center_axis',(-3.85185988875507E-34,1.,0.));
#111775=DIRECTION('ref_axis',(1.,0.,0.));
#111776=DIRECTION('center_axis',(-3.85185988875507E-34,1.,0.));
#111777=DIRECTION('ref_axis',(0.,0.,1.));
#111778=DIRECTION('center_axis',(-3.85185988875507E-34,1.,0.));
#111779=DIRECTION('ref_axis',(0.,0.,1.));
#111780=DIRECTION('center_axis',(-3.85185988875507E-34,1.,0.));
#111781=DIRECTION('ref_axis',(1.,0.,0.));
#111782=DIRECTION('center_axis',(-3.85185988875507E-34,1.,0.));
#111783=DIRECTION('ref_axis',(0.,0.,1.));
#111784=DIRECTION('center_axis',(-3.85185988875507E-34,1.,0.));
#111785=DIRECTION('ref_axis',(0.,0.,1.));
#111786=DIRECTION('center_axis',(-3.85185988875507E-34,1.,0.));
#111787=DIRECTION('ref_axis',(1.,0.,0.));
#111788=DIRECTION('center_axis',(-3.85185988875507E-34,1.,0.));
#111789=DIRECTION('ref_axis',(0.,0.,1.));
#111790=DIRECTION('center_axis',(-3.85185988875507E-34,1.,0.));
#111791=DIRECTION('ref_axis',(0.,0.,1.));
#111792=DIRECTION('center_axis',(-3.85185988875507E-34,1.,0.));
#111793=DIRECTION('ref_axis',(1.,0.,0.));
#111794=DIRECTION('center_axis',(-3.85185988875507E-34,1.,0.));
#111795=DIRECTION('ref_axis',(0.,0.,1.));
#111796=DIRECTION('center_axis',(-3.85185988875507E-34,1.,0.));
#111797=DIRECTION('ref_axis',(0.,0.,1.));
#111798=DIRECTION('center_axis',(-3.85185988875507E-34,1.,0.));
#111799=DIRECTION('ref_axis',(1.,0.,0.));
#111800=DIRECTION('center_axis',(-3.85185988875507E-34,1.,0.));
#111801=DIRECTION('ref_axis',(0.,0.,1.));
#111802=DIRECTION('center_axis',(-3.85185988875507E-34,1.,0.));
#111803=DIRECTION('ref_axis',(0.,0.,1.));
#111804=DIRECTION('center_axis',(-3.85185988875507E-34,1.,0.));
#111805=DIRECTION('ref_axis',(1.,0.,0.));
#111806=DIRECTION('center_axis',(-3.85185988875507E-34,1.,0.));
#111807=DIRECTION('ref_axis',(0.,0.,1.));
#111808=DIRECTION('center_axis',(-3.85185988875507E-34,1.,0.));
#111809=DIRECTION('ref_axis',(0.,0.,1.));
#111810=DIRECTION('center_axis',(-3.85185988875507E-34,1.,0.));
#111811=DIRECTION('ref_axis',(1.,0.,0.));
#111812=DIRECTION('center_axis',(-3.85185988875507E-34,1.,0.));
#111813=DIRECTION('ref_axis',(0.,0.,1.));
#111814=DIRECTION('center_axis',(-3.85185988875507E-34,1.,0.));
#111815=DIRECTION('ref_axis',(0.,0.,1.));
#111816=DIRECTION('center_axis',(-3.85185988875507E-34,1.,0.));
#111817=DIRECTION('ref_axis',(1.,0.,0.));
#111818=DIRECTION('center_axis',(-3.85185988875507E-34,1.,0.));
#111819=DIRECTION('ref_axis',(0.,0.,1.));
#111820=DIRECTION('center_axis',(-3.85185988875507E-34,1.,0.));
#111821=DIRECTION('ref_axis',(0.,0.,1.));
#111822=DIRECTION('center_axis',(-3.85185988875507E-34,1.,0.));
#111823=DIRECTION('ref_axis',(1.,0.,0.));
#111824=DIRECTION('center_axis',(-3.85185988875507E-34,1.,0.));
#111825=DIRECTION('ref_axis',(0.,0.,1.));
#111826=DIRECTION('center_axis',(-3.85185988875507E-34,1.,0.));
#111827=DIRECTION('ref_axis',(0.,0.,1.));
#111828=DIRECTION('center_axis',(-3.85185988875507E-34,1.,0.));
#111829=DIRECTION('ref_axis',(1.,0.,0.));
#111830=DIRECTION('center_axis',(-3.85185988875507E-34,1.,0.));
#111831=DIRECTION('ref_axis',(0.,0.,1.));
#111832=DIRECTION('center_axis',(-3.85185988875507E-34,1.,0.));
#111833=DIRECTION('ref_axis',(0.,0.,1.));
#111834=DIRECTION('center_axis',(-3.85185988875507E-34,1.,0.));
#111835=DIRECTION('ref_axis',(1.,0.,0.));
#111836=DIRECTION('center_axis',(-3.85185988875507E-34,1.,0.));
#111837=DIRECTION('ref_axis',(0.,0.,1.));
#111838=DIRECTION('center_axis',(-3.85185988875507E-34,1.,0.));
#111839=DIRECTION('ref_axis',(0.,0.,1.));
#111840=DIRECTION('center_axis',(-3.85185988875507E-34,1.,0.));
#111841=DIRECTION('ref_axis',(1.,0.,0.));
#111842=DIRECTION('center_axis',(-3.85185988875507E-34,1.,0.));
#111843=DIRECTION('ref_axis',(0.,0.,1.));
#111844=DIRECTION('center_axis',(-3.85185988875507E-34,1.,0.));
#111845=DIRECTION('ref_axis',(0.,0.,1.));
#111846=DIRECTION('center_axis',(-3.85185988875507E-34,1.,0.));
#111847=DIRECTION('ref_axis',(1.,0.,0.));
#111848=DIRECTION('center_axis',(-3.85185988875507E-34,1.,0.));
#111849=DIRECTION('ref_axis',(0.,0.,1.));
#111850=DIRECTION('center_axis',(-3.85185988875507E-34,1.,0.));
#111851=DIRECTION('ref_axis',(0.,0.,1.));
#111852=DIRECTION('center_axis',(-3.85185988875507E-34,1.,0.));
#111853=DIRECTION('ref_axis',(1.,0.,0.));
#111854=DIRECTION('center_axis',(-3.85185988875507E-34,1.,0.));
#111855=DIRECTION('ref_axis',(0.,0.,1.));
#111856=DIRECTION('center_axis',(-3.85185988875507E-34,1.,0.));
#111857=DIRECTION('ref_axis',(0.,0.,1.));
#111858=DIRECTION('center_axis',(-3.85185988875507E-34,1.,0.));
#111859=DIRECTION('ref_axis',(1.,0.,0.));
#111860=DIRECTION('center_axis',(-3.85185988875507E-34,1.,0.));
#111861=DIRECTION('ref_axis',(0.,0.,1.));
#111862=DIRECTION('center_axis',(-3.85185988875507E-34,1.,0.));
#111863=DIRECTION('ref_axis',(0.,0.,1.));
#111864=DIRECTION('center_axis',(-3.85185988875507E-34,1.,0.));
#111865=DIRECTION('ref_axis',(1.,0.,0.));
#111866=DIRECTION('center_axis',(-3.85185988875507E-34,1.,0.));
#111867=DIRECTION('ref_axis',(0.,0.,1.));
#111868=DIRECTION('center_axis',(-3.85185988875507E-34,1.,0.));
#111869=DIRECTION('ref_axis',(0.,0.,1.));
#111870=DIRECTION('center_axis',(-3.85185988875507E-34,1.,0.));
#111871=DIRECTION('ref_axis',(1.,0.,0.));
#111872=DIRECTION('center_axis',(-3.85185988875507E-34,1.,0.));
#111873=DIRECTION('ref_axis',(0.,0.,1.));
#111874=DIRECTION('center_axis',(-3.85185988875507E-34,1.,0.));
#111875=DIRECTION('ref_axis',(0.,0.,1.));
#111876=DIRECTION('center_axis',(-3.85185988875507E-34,1.,0.));
#111877=DIRECTION('ref_axis',(1.,0.,0.));
#111878=DIRECTION('center_axis',(-3.85185988875507E-34,1.,0.));
#111879=DIRECTION('ref_axis',(0.,0.,1.));
#111880=DIRECTION('center_axis',(-3.85185988875507E-34,1.,0.));
#111881=DIRECTION('ref_axis',(0.,0.,1.));
#111882=DIRECTION('center_axis',(-3.85185988875507E-34,1.,0.));
#111883=DIRECTION('ref_axis',(1.,0.,0.));
#111884=DIRECTION('center_axis',(-3.85185988875507E-34,1.,0.));
#111885=DIRECTION('ref_axis',(0.,0.,1.));
#111886=DIRECTION('center_axis',(-3.85185988875507E-34,1.,0.));
#111887=DIRECTION('ref_axis',(0.,0.,1.));
#111888=DIRECTION('center_axis',(-3.85185988875507E-34,1.,0.));
#111889=DIRECTION('ref_axis',(1.,0.,0.));
#111890=DIRECTION('center_axis',(-3.85185988875507E-34,1.,0.));
#111891=DIRECTION('ref_axis',(0.,0.,1.));
#111892=DIRECTION('center_axis',(-3.85185988875507E-34,1.,0.));
#111893=DIRECTION('ref_axis',(0.,0.,1.));
#111894=DIRECTION('center_axis',(-3.85185988875507E-34,1.,0.));
#111895=DIRECTION('ref_axis',(1.,0.,0.));
#111896=DIRECTION('center_axis',(-3.85185988875507E-34,1.,0.));
#111897=DIRECTION('ref_axis',(0.,0.,1.));
#111898=DIRECTION('center_axis',(-3.85185988875507E-34,1.,0.));
#111899=DIRECTION('ref_axis',(0.,0.,1.));
#111900=DIRECTION('center_axis',(-3.85185988875507E-34,1.,0.));
#111901=DIRECTION('ref_axis',(1.,0.,0.));
#111902=DIRECTION('center_axis',(-3.85185988875507E-34,1.,0.));
#111903=DIRECTION('ref_axis',(0.,0.,1.));
#111904=DIRECTION('center_axis',(-3.85185988875507E-34,1.,0.));
#111905=DIRECTION('ref_axis',(0.,0.,1.));
#111906=DIRECTION('center_axis',(-3.85185988875507E-34,1.,0.));
#111907=DIRECTION('ref_axis',(1.,0.,0.));
#111908=DIRECTION('center_axis',(-3.85185988875507E-34,1.,0.));
#111909=DIRECTION('ref_axis',(0.,0.,1.));
#111910=DIRECTION('center_axis',(-3.85185988875507E-34,1.,0.));
#111911=DIRECTION('ref_axis',(0.,0.,1.));
#111912=DIRECTION('center_axis',(-3.85185988875507E-34,1.,0.));
#111913=DIRECTION('ref_axis',(1.,0.,0.));
#111914=DIRECTION('center_axis',(-3.85185988875507E-34,1.,0.));
#111915=DIRECTION('ref_axis',(0.,0.,1.));
#111916=DIRECTION('center_axis',(-3.85185988875507E-34,1.,0.));
#111917=DIRECTION('ref_axis',(0.,0.,1.));
#111918=DIRECTION('center_axis',(3.85185988875507E-34,-1.,0.));
#111919=DIRECTION('ref_axis',(-1.,-3.85185988875507E-34,0.));
#111920=DIRECTION('center_axis',(3.85185988875507E-34,-1.,0.));
#111921=DIRECTION('ref_axis',(0.,0.,1.));
#111922=DIRECTION('',(0.707106780557139,-0.707106781815956,8.6595605546469E-17));
#111923=DIRECTION('center_axis',(-3.85185988875507E-34,1.,0.));
#111924=DIRECTION('ref_axis',(0.,0.,-1.));
#111925=DIRECTION('center_axis',(3.85185988875507E-34,-1.,0.));
#111926=DIRECTION('ref_axis',(0.,0.,1.));
#111927=DIRECTION('center_axis',(3.85185988875507E-34,-1.,0.));
#111928=DIRECTION('ref_axis',(-1.,-3.85185988875507E-34,0.));
#111929=DIRECTION('center_axis',(3.85185988875507E-34,-1.,0.));
#111930=DIRECTION('ref_axis',(0.,0.,1.));
#111931=DIRECTION('',(0.707106780557139,-0.707106781815956,8.6595605546469E-17));
#111932=DIRECTION('center_axis',(-3.85185988875507E-34,1.,0.));
#111933=DIRECTION('ref_axis',(0.,0.,-1.));
#111934=DIRECTION('center_axis',(3.85185988875507E-34,-1.,0.));
#111935=DIRECTION('ref_axis',(0.,0.,1.));
#111936=DIRECTION('center_axis',(3.85185988875507E-34,-1.,0.));
#111937=DIRECTION('ref_axis',(-1.,-3.85185988875507E-34,0.));
#111938=DIRECTION('center_axis',(3.85185988875507E-34,-1.,0.));
#111939=DIRECTION('ref_axis',(0.,0.,1.));
#111940=DIRECTION('',(0.707106780557139,-0.707106781815956,8.6595605546469E-17));
#111941=DIRECTION('center_axis',(-3.85185988875507E-34,1.,0.));
#111942=DIRECTION('ref_axis',(0.,0.,-1.));
#111943=DIRECTION('center_axis',(3.85185988875507E-34,-1.,0.));
#111944=DIRECTION('ref_axis',(0.,0.,1.));
#111945=DIRECTION('center_axis',(3.85185988875507E-34,-1.,0.));
#111946=DIRECTION('ref_axis',(-1.,-3.85185988875507E-34,0.));
#111947=DIRECTION('center_axis',(3.85185988875507E-34,-1.,0.));
#111948=DIRECTION('ref_axis',(0.,0.,1.));
#111949=DIRECTION('',(-0.707106780557139,0.707106781815956,-8.65956055464691E-17));
#111950=DIRECTION('center_axis',(-3.85185988875507E-34,1.,0.));
#111951=DIRECTION('ref_axis',(0.,0.,-1.));
#111952=DIRECTION('center_axis',(3.85185988875507E-34,-1.,0.));
#111953=DIRECTION('ref_axis',(0.,0.,1.));
#111954=DIRECTION('center_axis',(-3.85185988875507E-34,1.,0.));
#111955=DIRECTION('ref_axis',(1.,3.85185988875507E-34,0.));
#111956=DIRECTION('center_axis',(-3.85185988875507E-34,1.,0.));
#111957=DIRECTION('ref_axis',(0.,0.,1.));
#111958=DIRECTION('',(-0.707106780557139,0.707106781815956,8.6595605546469E-17));
#111959=DIRECTION('center_axis',(3.85185988875507E-34,-1.,0.));
#111960=DIRECTION('ref_axis',(0.,0.,1.));
#111961=DIRECTION('center_axis',(-3.85185988875507E-34,1.,0.));
#111962=DIRECTION('ref_axis',(1.,3.85185988875507E-34,0.));
#111963=DIRECTION('center_axis',(-3.85185988875507E-34,1.,0.));
#111964=DIRECTION('ref_axis',(0.,0.,1.));
#111965=DIRECTION('',(-0.707106780557139,0.707106781815956,8.6595605546469E-17));
#111966=DIRECTION('center_axis',(3.85185988875507E-34,-1.,0.));
#111967=DIRECTION('ref_axis',(0.,0.,1.));
#111968=DIRECTION('center_axis',(3.85185988875507E-34,-1.,0.));
#111969=DIRECTION('ref_axis',(-1.,-3.85185988875507E-34,0.));
#111970=DIRECTION('center_axis',(3.85185988875507E-34,-1.,0.));
#111971=DIRECTION('ref_axis',(0.,0.,1.));
#111972=DIRECTION('',(-0.707106780557139,0.707106781815956,-8.65956055464691E-17));
#111973=DIRECTION('center_axis',(-3.85185988875507E-34,1.,0.));
#111974=DIRECTION('ref_axis',(0.,0.,-1.));
#111975=DIRECTION('center_axis',(3.85185988875507E-34,-1.,0.));
#111976=DIRECTION('ref_axis',(0.,0.,1.));
#111977=DIRECTION('center_axis',(-3.85185988875507E-34,1.,0.));
#111978=DIRECTION('ref_axis',(1.,3.85185988875507E-34,0.));
#111979=DIRECTION('center_axis',(-3.85185988875507E-34,1.,0.));
#111980=DIRECTION('ref_axis',(0.,0.,1.));
#111981=DIRECTION('',(-0.707106780557139,0.707106781815956,8.6595605546469E-17));
#111982=DIRECTION('center_axis',(3.85185988875507E-34,-1.,0.));
#111983=DIRECTION('ref_axis',(0.,0.,1.));
#111984=DIRECTION('center_axis',(-3.85185988875507E-34,1.,0.));
#111985=DIRECTION('ref_axis',(1.,3.85185988875507E-34,0.));
#111986=DIRECTION('',(-3.85185988875507E-34,1.,0.));
#111987=DIRECTION('center_axis',(-3.85185988875507E-34,1.,0.));
#111988=DIRECTION('ref_axis',(1.,3.85185988875507E-34,0.));
#111989=DIRECTION('',(-3.85185988875507E-34,1.,0.));
#111990=DIRECTION('center_axis',(-3.85185988875507E-34,1.,0.));
#111991=DIRECTION('ref_axis',(1.,3.85185988875507E-34,0.));
#111992=DIRECTION('',(0.707106780557139,-0.707106781815956,-8.6595605546469E-17));
#111993=DIRECTION('center_axis',(-3.85185988875507E-34,1.,0.));
#111994=DIRECTION('ref_axis',(0.,0.,1.));
#111995=DIRECTION('center_axis',(-3.85185988875507E-34,1.,0.));
#111996=DIRECTION('ref_axis',(1.,3.85185988875507E-34,0.));
#111997=DIRECTION('',(3.85185988875507E-34,-1.,0.));
#111998=DIRECTION('center_axis',(-3.85185988875507E-34,1.,0.));
#111999=DIRECTION('ref_axis',(1.,3.85185988875507E-34,0.));
#112000=DIRECTION('',(3.85185988875507E-34,-1.,0.));
#112001=DIRECTION('center_axis',(-3.85185988875507E-34,1.,0.));
#112002=DIRECTION('ref_axis',(0.,0.,1.));
#112003=DIRECTION('center_axis',(-3.85185988875507E-34,1.,0.));
#112004=DIRECTION('ref_axis',(1.,3.85185988875507E-34,0.));
#112005=DIRECTION('',(-3.85185988875507E-34,1.,0.));
#112006=DIRECTION('center_axis',(-3.85185988875507E-34,1.,0.));
#112007=DIRECTION('ref_axis',(1.,3.85185988875507E-34,0.));
#112008=DIRECTION('center_axis',(-3.85185988875507E-34,1.,0.));
#112009=DIRECTION('ref_axis',(1.,3.85185988875507E-34,0.));
#112010=DIRECTION('center_axis',(3.85185988875507E-34,-1.,0.));
#112011=DIRECTION('ref_axis',(-1.,-3.85185988875507E-34,0.));
#112012=DIRECTION('center_axis',(0.,0.,-1.));
#112013=DIRECTION('ref_axis',(-3.85185988875507E-34,1.,0.));
#112014=DIRECTION('center_axis',(0.,0.,-1.));
#112015=DIRECTION('ref_axis',(-1.,-3.85185988875507E-34,0.));
#112016=DIRECTION('center_axis',(0.,0.,-1.));
#112017=DIRECTION('ref_axis',(0.,1.,0.));
#112018=DIRECTION('center_axis',(0.,0.,-1.));
#112019=DIRECTION('ref_axis',(-1.,-3.85185988875507E-34,0.));
#112020=DIRECTION('center_axis',(0.,0.,1.));
#112021=DIRECTION('ref_axis',(3.85185988875507E-34,-1.,0.));
#112022=DIRECTION('center_axis',(-0.089639308998799,-3.45278058788195E-35,
-0.995974293986656));
#112023=DIRECTION('ref_axis',(-3.85185988875507E-34,1.,0.));
#112024=DIRECTION('center_axis',(-0.089639308998799,-3.45278058788195E-35,
-0.995974293986656));
#112025=DIRECTION('ref_axis',(-0.995974293986656,-3.83635343323835E-34,
0.089639308998799));
#112026=DIRECTION('center_axis',(-0.089639308998799,-3.45278058788195E-35,
-0.995974293986656));
#112027=DIRECTION('ref_axis',(0.,1.,0.));
#112028=DIRECTION('center_axis',(-0.089639308998799,-3.45278058788195E-35,
-0.995974293986656));
#112029=DIRECTION('ref_axis',(-0.995974293986656,-3.83635343323835E-34,
0.089639308998799));
#112030=DIRECTION('center_axis',(0.089639308998799,3.45278058788195E-35,
0.995974293986656));
#112031=DIRECTION('ref_axis',(3.85185988875507E-34,-1.,0.));
#112032=DIRECTION('center_axis',(-0.178556894923064,-6.87776141414805E-35,
-0.98392958857605));
#112033=DIRECTION('ref_axis',(-3.85185988875507E-34,1.,0.));
#112034=DIRECTION('center_axis',(-0.178556894923064,-6.87776141414805E-35,
-0.98392958857605));
#112035=DIRECTION('ref_axis',(-0.983929588576049,-3.78995891559536E-34,
0.178556894923064));
#112036=DIRECTION('center_axis',(-0.178556894923064,-6.87776141414805E-35,
-0.98392958857605));
#112037=DIRECTION('ref_axis',(0.,1.,0.));
#112038=DIRECTION('center_axis',(-0.178556894923064,-6.87776141414805E-35,
-0.98392958857605));
#112039=DIRECTION('ref_axis',(-0.983929588576049,-3.78995891559536E-34,
0.178556894923064));
#112040=DIRECTION('center_axis',(0.178556894923064,6.87776141414805E-35,
0.98392958857605));
#112041=DIRECTION('ref_axis',(3.85185988875507E-34,-1.,0.));
#112042=DIRECTION('center_axis',(-0.266036845891333,-1.02473665561974E-34,
-0.963962860606254));
#112043=DIRECTION('ref_axis',(-3.85185988875507E-34,1.,0.));
#112044=DIRECTION('center_axis',(-0.266036845891333,-1.02473665561974E-34,
-0.963962860606254));
#112045=DIRECTION('ref_axis',(-0.963962860606253,-3.71304987701882E-34,
0.266036845891333));
#112046=DIRECTION('center_axis',(-0.266036845891333,-1.02473665561974E-34,
-0.963962860606254));
#112047=DIRECTION('ref_axis',(0.,1.,0.));
#112048=DIRECTION('center_axis',(-0.266036845891333,-1.02473665561974E-34,
-0.963962860606254));
#112049=DIRECTION('ref_axis',(-0.963962860606253,-3.71304987701882E-34,
0.266036845891333));
#112050=DIRECTION('center_axis',(0.266036845891333,1.02473665561974E-34,
0.963962860606254));
#112051=DIRECTION('ref_axis',(3.85185988875507E-34,-1.,0.));
#112052=DIRECTION('center_axis',(-0.351374823891528,-1.35344659006615E-34,
-0.936234870710976));
#112053=DIRECTION('ref_axis',(-3.85185988875507E-34,1.,0.));
#112054=DIRECTION('center_axis',(-0.351374823891528,-1.35344659006615E-34,
-0.936234870710976));
#112055=DIRECTION('ref_axis',(-0.936234870710976,-3.60624554494539E-34,
0.351374823891528));
#112056=DIRECTION('center_axis',(-0.351374823891528,-1.35344659006615E-34,
-0.936234870710976));
#112057=DIRECTION('ref_axis',(0.,1.,0.));
#112058=DIRECTION('center_axis',(-0.351374823891528,-1.35344659006615E-34,
-0.936234870710976));
#112059=DIRECTION('ref_axis',(-0.936234870710976,-3.60624554494539E-34,
0.351374823891528));
#112060=DIRECTION('center_axis',(0.351374823891528,1.35344659006615E-34,
0.936234870710976));
#112061=DIRECTION('ref_axis',(3.85185988875507E-34,-1.,0.));
#112062=DIRECTION('center_axis',(-0.433883738983985,-1.67125937057549E-34,
-0.900968867966745));
#112063=DIRECTION('ref_axis',(-3.85185988875507E-34,1.,0.));
#112064=DIRECTION('center_axis',(-0.433883738983985,-1.67125937057549E-34,
-0.900968867966745));
#112065=DIRECTION('ref_axis',(-0.900968867966744,-3.47040584353816E-34,
0.433883738983985));
#112066=DIRECTION('center_axis',(-0.433883738983985,-1.67125937057549E-34,
-0.900968867966745));
#112067=DIRECTION('ref_axis',(0.,1.,0.));
#112068=DIRECTION('center_axis',(-0.433883738983985,-1.67125937057549E-34,
-0.900968867966745));
#112069=DIRECTION('ref_axis',(-0.900968867966744,-3.47040584353816E-34,
0.433883738983985));
#112070=DIRECTION('center_axis',(0.433883738983985,1.67125937057549E-34,
0.900968867966745));
#112071=DIRECTION('ref_axis',(3.85185988875507E-34,-1.,0.));
#112072=DIRECTION('center_axis',(-0.512899276931483,-1.97561615178386E-34,
-0.858448793885321));
#112073=DIRECTION('ref_axis',(-3.85185988875507E-34,1.,0.));
#112074=DIRECTION('center_axis',(-0.512899276931483,-1.97561615178386E-34,
-0.858448793885321));
#112075=DIRECTION('ref_axis',(-0.858448793885321,-3.30662447571703E-34,
0.512899276931483));
#112076=DIRECTION('center_axis',(-0.512899276931483,-1.97561615178386E-34,
-0.858448793885321));
#112077=DIRECTION('ref_axis',(0.,1.,0.));
#112078=DIRECTION('center_axis',(-0.512899276931483,-1.97561615178386E-34,
-0.858448793885321));
#112079=DIRECTION('ref_axis',(-0.858448793885321,-3.30662447571703E-34,
0.512899276931483));
#112080=DIRECTION('center_axis',(0.512899276931483,1.97561615178386E-34,
0.858448793885321));
#112081=DIRECTION('ref_axis',(3.85185988875507E-34,-1.,0.));
#112082=DIRECTION('center_axis',(-0.587785252279345,-2.26406643645659E-34,
-0.809016994384486));
#112083=DIRECTION('ref_axis',(-3.85185988875507E-34,1.,0.));
#112084=DIRECTION('center_axis',(-0.587785252279345,-2.26406643645659E-34,
-0.809016994384486));
#112085=DIRECTION('ref_axis',(-0.809016994384486,-3.11622010999078E-34,
0.587785252279345));
#112086=DIRECTION('center_axis',(-0.587785252279345,-2.26406643645659E-34,
-0.809016994384486));
#112087=DIRECTION('ref_axis',(0.,1.,0.));
#112088=DIRECTION('center_axis',(-0.587785252279345,-2.26406643645659E-34,
-0.809016994384486));
#112089=DIRECTION('ref_axis',(-0.809016994384486,-3.11622010999078E-34,
0.587785252279345));
#112090=DIRECTION('center_axis',(0.587785252279345,2.26406643645659E-34,
0.809016994384486));
#112091=DIRECTION('ref_axis',(3.85185988875507E-34,-1.,0.));
#112092=DIRECTION('center_axis',(-0.657938725975692,-2.53428778784438E-34,
-0.753071465972177));
#112093=DIRECTION('ref_axis',(-3.85185988875507E-34,1.,0.));
#112094=DIRECTION('center_axis',(-0.657938725975692,-2.53428778784438E-34,
-0.753071465972177));
#112095=DIRECTION('ref_axis',(-0.753071465972177,-2.9007257731442E-34,0.657938725975692));
#112096=DIRECTION('center_axis',(-0.657938725975692,-2.53428778784438E-34,
-0.753071465972177));
#112097=DIRECTION('ref_axis',(0.,1.,0.));
#112098=DIRECTION('center_axis',(-0.657938725975692,-2.53428778784438E-34,
-0.753071465972177));
#112099=DIRECTION('ref_axis',(-0.753071465972177,-2.9007257731442E-34,0.657938725975692));
#112100=DIRECTION('center_axis',(0.657938725975692,2.53428778784438E-34,
0.753071465972177));
#112101=DIRECTION('ref_axis',(3.85185988875507E-34,-1.,0.));
#112102=DIRECTION('center_axis',(-0.722794863903263,-2.78410454406716E-34,
-0.69106264890751));
#112103=DIRECTION('ref_axis',(-3.85185988875507E-34,1.,0.));
#112104=DIRECTION('center_axis',(-0.722794863903263,-2.78410454406716E-34,
-0.69106264890751));
#112105=DIRECTION('ref_axis',(-0.69106264890751,-2.66187649794366E-34,0.722794863903263));
#112106=DIRECTION('center_axis',(-0.722794863903263,-2.78410454406716E-34,
-0.69106264890751));
#112107=DIRECTION('ref_axis',(0.,1.,0.));
#112108=DIRECTION('center_axis',(-0.722794863903263,-2.78410454406716E-34,
-0.69106264890751));
#112109=DIRECTION('ref_axis',(-0.69106264890751,-2.66187649794366E-34,0.722794863903263));
#112110=DIRECTION('center_axis',(0.722794863903263,2.78410454406716E-34,
0.69106264890751));
#112111=DIRECTION('ref_axis',(3.85185988875507E-34,-1.,0.));
#112112=DIRECTION('center_axis',(-0.781831482217226,-3.01150532611845E-34,
-0.623489802173232));
#112113=DIRECTION('ref_axis',(-3.85185988875507E-34,1.,0.));
#112114=DIRECTION('center_axis',(-0.781831482217226,-3.01150532611845E-34,
-0.623489802173232));
#112115=DIRECTION('ref_axis',(-0.623489802173232,-2.4015953600389E-34,0.781831482217226));
#112116=DIRECTION('center_axis',(-0.781831482217226,-3.01150532611845E-34,
-0.623489802173232));
#112117=DIRECTION('ref_axis',(0.,1.,0.));
#112118=DIRECTION('center_axis',(-0.781831482217226,-3.01150532611845E-34,
-0.623489802173232));
#112119=DIRECTION('ref_axis',(-0.623489802173232,-2.4015953600389E-34,0.781831482217226));
#112120=DIRECTION('center_axis',(0.781831482217226,3.01150532611845E-34,
0.623489802173232));
#112121=DIRECTION('ref_axis',(3.85185988875507E-34,-1.,0.));
#112122=DIRECTION('center_axis',(-0.834573254013744,-3.21465924136334E-34,
-0.550896981009072));
#112123=DIRECTION('ref_axis',(-3.85185988875507E-34,1.,0.));
#112124=DIRECTION('center_axis',(-0.834573254013744,-3.21465924136334E-34,
-0.550896981009072));
#112125=DIRECTION('ref_axis',(-0.550896981009072,-2.12197798398511E-34,
0.834573254013744));
#112126=DIRECTION('center_axis',(-0.834573254013744,-3.21465924136334E-34,
-0.550896981009072));
#112127=DIRECTION('ref_axis',(0.,1.,0.));
#112128=DIRECTION('center_axis',(-0.834573254013744,-3.21465924136334E-34,
-0.550896981009072));
#112129=DIRECTION('ref_axis',(-0.550896981009072,-2.12197798398511E-34,
0.834573254013744));
#112130=DIRECTION('center_axis',(0.834573254013744,3.21465924136334E-34,
0.550896981009072));
#112131=DIRECTION('ref_axis',(3.85185988875507E-34,-1.,0.));
#112132=DIRECTION('center_axis',(-0.880595532086284,-3.39193060826008E-34,
-0.473868662046431));
#112133=DIRECTION('ref_axis',(-3.85185988875507E-34,1.,0.));
#112134=DIRECTION('center_axis',(-0.880595532086284,-3.39193060826008E-34,
-0.473868662046431));
#112135=DIRECTION('ref_axis',(-0.473868662046431,-1.82527569187468E-34,
0.880595532086284));
#112136=DIRECTION('center_axis',(-0.880595532086284,-3.39193060826008E-34,
-0.473868662046431));
#112137=DIRECTION('ref_axis',(0.,1.,0.));
#112138=DIRECTION('center_axis',(-0.880595532086284,-3.39193060826008E-34,
-0.473868662046431));
#112139=DIRECTION('ref_axis',(-0.473868662046431,-1.82527569187468E-34,
0.880595532086284));
#112140=DIRECTION('center_axis',(0.880595532086284,3.39193060826008E-34,
0.473868662046431));
#112141=DIRECTION('ref_axis',(3.85185988875507E-34,-1.,0.));
#112142=DIRECTION('center_axis',(-0.919527772341198,-3.54189214287736E-34,
-0.393025032145835));
#112143=DIRECTION('ref_axis',(-3.85185988875507E-34,1.,0.));
#112144=DIRECTION('center_axis',(-0.919527772341198,-3.54189214287736E-34,
-0.393025032145835));
#112145=DIRECTION('ref_axis',(-0.393025032145835,-1.51387735659921E-34,
0.919527772341198));
#112146=DIRECTION('center_axis',(-0.919527772341198,-3.54189214287736E-34,
-0.393025032145835));
#112147=DIRECTION('ref_axis',(0.,1.,0.));
#112148=DIRECTION('center_axis',(-0.919527772341198,-3.54189214287736E-34,
-0.393025032145835));
#112149=DIRECTION('ref_axis',(-0.393025032145835,-1.51387735659921E-34,
0.919527772341198));
#112150=DIRECTION('center_axis',(0.919527772341198,3.54189214287736E-34,
0.393025032145835));
#112151=DIRECTION('ref_axis',(3.85185988875507E-34,-1.,0.));
#112152=DIRECTION('center_axis',(-0.951056516377163,-3.66333644737232E-34,
-0.309016994122548));
#112153=DIRECTION('ref_axis',(-3.85185988875507E-34,1.,0.));
#112154=DIRECTION('center_axis',(-0.951056516377163,-3.66333644737232E-34,
-0.309016994122548));
#112155=DIRECTION('ref_axis',(-0.309016994122548,-1.1902901646043E-34,0.951056516377163));
#112156=DIRECTION('center_axis',(-0.951056516377163,-3.66333644737232E-34,
-0.309016994122548));
#112157=DIRECTION('ref_axis',(0.,1.,0.));
#112158=DIRECTION('center_axis',(-0.951056516377163,-3.66333644737232E-34,
-0.309016994122548));
#112159=DIRECTION('ref_axis',(-0.309016994122548,-1.1902901646043E-34,0.951056516377163));
#112160=DIRECTION('center_axis',(0.951056516377163,3.66333644737232E-34,
0.309016994122548));
#112161=DIRECTION('ref_axis',(3.85185988875507E-34,-1.,0.));
#112162=DIRECTION('center_axis',(-0.974927912163343,-3.75528571928971E-34,
-0.222520934037282));
#112163=DIRECTION('ref_axis',(-3.85185988875507E-34,1.,0.));
#112164=DIRECTION('center_axis',(-0.974927912163343,-3.75528571928971E-34,
-0.222520934037282));
#112165=DIRECTION('ref_axis',(-0.222520934037282,-8.57119460226519E-35,
0.974927912163343));
#112166=DIRECTION('center_axis',(-0.974927912163343,-3.75528571928971E-34,
-0.222520934037282));
#112167=DIRECTION('ref_axis',(0.,1.,0.));
#112168=DIRECTION('center_axis',(-0.974927912163343,-3.75528571928971E-34,
-0.222520934037282));
#112169=DIRECTION('ref_axis',(-0.222520934037282,-8.57119460226519E-35,
0.974927912163343));
#112170=DIRECTION('center_axis',(0.974927912163343,3.75528571928971E-34,
0.222520934037282));
#112171=DIRECTION('ref_axis',(3.85185988875507E-34,-1.,0.));
#112172=DIRECTION('center_axis',(-0.990949761747861,-3.81699963904798E-34,
-0.134233265965845));
#112173=DIRECTION('ref_axis',(-3.85185988875507E-34,1.,0.));
#112174=DIRECTION('center_axis',(-0.990949761747861,-3.81699963904798E-34,
-0.134233265965845));
#112175=DIRECTION('ref_axis',(-0.134233265965845,-5.17047732910431E-35,
0.990949761747861));
#112176=DIRECTION('center_axis',(-0.990949761747861,-3.81699963904798E-34,
-0.134233265965845));
#112177=DIRECTION('ref_axis',(0.,1.,0.));
#112178=DIRECTION('center_axis',(-0.990949761747861,-3.81699963904798E-34,
-0.134233265965845));
#112179=DIRECTION('ref_axis',(-0.134233265965845,-5.17047732910431E-35,
0.990949761747861));
#112180=DIRECTION('center_axis',(0.990949761747861,3.81699963904798E-34,
0.134233265965845));
#112181=DIRECTION('ref_axis',(3.85185988875507E-34,-1.,0.));
#112182=DIRECTION('center_axis',(-0.998993066557948,-3.84798132221898E-34,
-0.0448648299801474));
#112183=DIRECTION('ref_axis',(-3.85185988875507E-34,1.,0.));
#112184=DIRECTION('center_axis',(-0.998993066557948,-3.84798132221898E-34,
-0.0448648299801474));
#112185=DIRECTION('ref_axis',(-0.0448648299801474,-1.72813039016346E-35,
0.998993066557948));
#112186=DIRECTION('center_axis',(-0.998993066557948,-3.84798132221898E-34,
-0.0448648299801474));
#112187=DIRECTION('ref_axis',(0.,1.,0.));
#112188=DIRECTION('center_axis',(-0.998993066557948,-3.84798132221898E-34,
-0.0448648299801474));
#112189=DIRECTION('ref_axis',(-0.0448648299801474,-1.72813039016346E-35,
0.998993066557948));
#112190=DIRECTION('center_axis',(0.998993066557948,3.84798132221898E-34,
0.0448648299801474));
#112191=DIRECTION('ref_axis',(3.85185988875507E-34,-1.,0.));
#112192=DIRECTION('center_axis',(-0.998993066557948,-3.84798132221898E-34,
0.0448648299801474));
#112193=DIRECTION('ref_axis',(-3.85185988875507E-34,1.,0.));
#112194=DIRECTION('center_axis',(-0.998993066557948,-3.84798132221898E-34,
0.0448648299801474));
#112195=DIRECTION('ref_axis',(0.0448648299801474,1.72813039016346E-35,0.998993066557948));
#112196=DIRECTION('center_axis',(-0.998993066557948,-3.84798132221898E-34,
0.0448648299801474));
#112197=DIRECTION('ref_axis',(0.,1.,0.));
#112198=DIRECTION('center_axis',(-0.998993066557948,-3.84798132221898E-34,
0.0448648299801474));
#112199=DIRECTION('ref_axis',(0.0448648299801474,1.72813039016346E-35,0.998993066557948));
#112200=DIRECTION('center_axis',(0.998993066557948,3.84798132221898E-34,
-0.0448648299801474));
#112201=DIRECTION('ref_axis',(3.85185988875507E-34,-1.,0.));
#112202=DIRECTION('center_axis',(-0.990949761747861,-3.81699963904798E-34,
0.134233265965845));
#112203=DIRECTION('ref_axis',(-3.85185988875507E-34,1.,0.));
#112204=DIRECTION('center_axis',(-0.990949761747861,-3.81699963904798E-34,
0.134233265965845));
#112205=DIRECTION('ref_axis',(0.134233265965845,5.17047732910431E-35,0.990949761747861));
#112206=DIRECTION('center_axis',(-0.990949761747861,-3.81699963904798E-34,
0.134233265965845));
#112207=DIRECTION('ref_axis',(0.,1.,0.));
#112208=DIRECTION('center_axis',(-0.990949761747861,-3.81699963904798E-34,
0.134233265965845));
#112209=DIRECTION('ref_axis',(0.134233265965845,5.17047732910431E-35,0.990949761747861));
#112210=DIRECTION('center_axis',(0.990949761747861,3.81699963904798E-34,
-0.134233265965845));
#112211=DIRECTION('ref_axis',(3.85185988875507E-34,-1.,0.));
#112212=DIRECTION('center_axis',(-0.974927912163343,-3.75528571928971E-34,
0.222520934037282));
#112213=DIRECTION('ref_axis',(-3.85185988875507E-34,1.,0.));
#112214=DIRECTION('center_axis',(-0.974927912163343,-3.75528571928971E-34,
0.222520934037282));
#112215=DIRECTION('ref_axis',(0.222520934037282,8.57119460226519E-35,0.974927912163343));
#112216=DIRECTION('center_axis',(-0.974927912163343,-3.75528571928971E-34,
0.222520934037282));
#112217=DIRECTION('ref_axis',(0.,1.,0.));
#112218=DIRECTION('center_axis',(-0.974927912163343,-3.75528571928971E-34,
0.222520934037282));
#112219=DIRECTION('ref_axis',(0.222520934037282,8.57119460226519E-35,0.974927912163343));
#112220=DIRECTION('center_axis',(0.974927912163343,3.75528571928971E-34,
-0.222520934037282));
#112221=DIRECTION('ref_axis',(3.85185988875507E-34,-1.,0.));
#112222=DIRECTION('center_axis',(-0.951056516377163,-3.66333644737232E-34,
0.309016994122548));
#112223=DIRECTION('ref_axis',(-3.85185988875507E-34,1.,0.));
#112224=DIRECTION('center_axis',(-0.951056516377163,-3.66333644737232E-34,
0.309016994122548));
#112225=DIRECTION('ref_axis',(0.309016994122548,1.1902901646043E-34,0.951056516377163));
#112226=DIRECTION('center_axis',(-0.951056516377163,-3.66333644737232E-34,
0.309016994122548));
#112227=DIRECTION('ref_axis',(0.,1.,0.));
#112228=DIRECTION('center_axis',(-0.951056516377163,-3.66333644737232E-34,
0.309016994122548));
#112229=DIRECTION('ref_axis',(0.309016994122548,1.1902901646043E-34,0.951056516377163));
#112230=DIRECTION('center_axis',(0.951056516377163,3.66333644737232E-34,
-0.309016994122548));
#112231=DIRECTION('ref_axis',(3.85185988875507E-34,-1.,0.));
#112232=DIRECTION('center_axis',(-0.919527772341198,-3.54189214287736E-34,
0.393025032145835));
#112233=DIRECTION('ref_axis',(-3.85185988875507E-34,1.,0.));
#112234=DIRECTION('center_axis',(-0.919527772341198,-3.54189214287736E-34,
0.393025032145835));
#112235=DIRECTION('ref_axis',(0.393025032145835,1.51387735659921E-34,0.919527772341198));
#112236=DIRECTION('center_axis',(-0.919527772341198,-3.54189214287736E-34,
0.393025032145835));
#112237=DIRECTION('ref_axis',(0.,1.,0.));
#112238=DIRECTION('center_axis',(-0.919527772341198,-3.54189214287736E-34,
0.393025032145835));
#112239=DIRECTION('ref_axis',(0.393025032145835,1.51387735659921E-34,0.919527772341198));
#112240=DIRECTION('center_axis',(0.919527772341198,3.54189214287736E-34,
-0.393025032145835));
#112241=DIRECTION('ref_axis',(3.85185988875507E-34,-1.,0.));
#112242=DIRECTION('center_axis',(-0.880595532086284,-3.39193060826008E-34,
0.473868662046431));
#112243=DIRECTION('ref_axis',(-3.85185988875507E-34,1.,0.));
#112244=DIRECTION('center_axis',(-0.880595532086284,-3.39193060826008E-34,
0.473868662046431));
#112245=DIRECTION('ref_axis',(0.473868662046431,1.82527569187468E-34,0.880595532086284));
#112246=DIRECTION('center_axis',(-0.880595532086284,-3.39193060826008E-34,
0.473868662046431));
#112247=DIRECTION('ref_axis',(0.,1.,0.));
#112248=DIRECTION('center_axis',(-0.880595532086284,-3.39193060826008E-34,
0.473868662046431));
#112249=DIRECTION('ref_axis',(0.473868662046431,1.82527569187468E-34,0.880595532086284));
#112250=DIRECTION('center_axis',(0.880595532086284,3.39193060826008E-34,
-0.473868662046431));
#112251=DIRECTION('ref_axis',(3.85185988875507E-34,-1.,0.));
#112252=DIRECTION('center_axis',(-0.834573254013744,-3.21465924136334E-34,
0.550896981009072));
#112253=DIRECTION('ref_axis',(-3.85185988875507E-34,1.,0.));
#112254=DIRECTION('center_axis',(-0.834573254013744,-3.21465924136334E-34,
0.550896981009072));
#112255=DIRECTION('ref_axis',(0.550896981009072,2.12197798398511E-34,0.834573254013744));
#112256=DIRECTION('center_axis',(-0.834573254013744,-3.21465924136334E-34,
0.550896981009072));
#112257=DIRECTION('ref_axis',(0.,1.,0.));
#112258=DIRECTION('center_axis',(-0.834573254013744,-3.21465924136334E-34,
0.550896981009072));
#112259=DIRECTION('ref_axis',(0.550896981009072,2.12197798398511E-34,0.834573254013744));
#112260=DIRECTION('center_axis',(0.834573254013744,3.21465924136334E-34,
-0.550896981009072));
#112261=DIRECTION('ref_axis',(3.85185988875507E-34,-1.,0.));
#112262=DIRECTION('center_axis',(-0.781831482217226,-3.01150532611845E-34,
0.623489802173232));
#112263=DIRECTION('ref_axis',(-3.85185988875507E-34,1.,0.));
#112264=DIRECTION('center_axis',(-0.781831482217226,-3.01150532611845E-34,
0.623489802173232));
#112265=DIRECTION('ref_axis',(0.623489802173232,2.4015953600389E-34,0.781831482217226));
#112266=DIRECTION('center_axis',(-0.781831482217226,-3.01150532611845E-34,
0.623489802173232));
#112267=DIRECTION('ref_axis',(0.,1.,0.));
#112268=DIRECTION('center_axis',(-0.781831482217226,-3.01150532611845E-34,
0.623489802173232));
#112269=DIRECTION('ref_axis',(0.623489802173232,2.4015953600389E-34,0.781831482217226));
#112270=DIRECTION('center_axis',(0.781831482217226,3.01150532611845E-34,
-0.623489802173232));
#112271=DIRECTION('ref_axis',(3.85185988875507E-34,-1.,0.));
#112272=DIRECTION('center_axis',(-0.722794863903263,-2.78410454406716E-34,
0.69106264890751));
#112273=DIRECTION('ref_axis',(-3.85185988875507E-34,1.,0.));
#112274=DIRECTION('center_axis',(-0.722794863903263,-2.78410454406716E-34,
0.69106264890751));
#112275=DIRECTION('ref_axis',(0.69106264890751,2.66187649794366E-34,0.722794863903263));
#112276=DIRECTION('center_axis',(-0.722794863903263,-2.78410454406716E-34,
0.69106264890751));
#112277=DIRECTION('ref_axis',(0.,1.,0.));
#112278=DIRECTION('center_axis',(-0.722794863903263,-2.78410454406716E-34,
0.69106264890751));
#112279=DIRECTION('ref_axis',(0.69106264890751,2.66187649794366E-34,0.722794863903263));
#112280=DIRECTION('center_axis',(0.722794863903263,2.78410454406716E-34,
-0.69106264890751));
#112281=DIRECTION('ref_axis',(3.85185988875507E-34,-1.,0.));
#112282=DIRECTION('center_axis',(-0.657938725975692,-2.53428778784438E-34,
0.753071465972177));
#112283=DIRECTION('ref_axis',(-3.85185988875507E-34,1.,0.));
#112284=DIRECTION('center_axis',(-0.657938725975692,-2.53428778784438E-34,
0.753071465972177));
#112285=DIRECTION('ref_axis',(0.753071465972177,2.9007257731442E-34,0.657938725975692));
#112286=DIRECTION('center_axis',(-0.657938725975692,-2.53428778784438E-34,
0.753071465972177));
#112287=DIRECTION('ref_axis',(0.,1.,0.));
#112288=DIRECTION('center_axis',(-0.657938725975692,-2.53428778784438E-34,
0.753071465972177));
#112289=DIRECTION('ref_axis',(0.753071465972177,2.9007257731442E-34,0.657938725975692));
#112290=DIRECTION('center_axis',(0.657938725975692,2.53428778784438E-34,
-0.753071465972177));
#112291=DIRECTION('ref_axis',(3.85185988875507E-34,-1.,0.));
#112292=DIRECTION('center_axis',(-0.587785252279345,-2.26406643645659E-34,
0.809016994384486));
#112293=DIRECTION('ref_axis',(-3.85185988875507E-34,1.,0.));
#112294=DIRECTION('center_axis',(-0.587785252279345,-2.26406643645659E-34,
0.809016994384486));
#112295=DIRECTION('ref_axis',(0.809016994384486,3.11622010999078E-34,0.587785252279345));
#112296=DIRECTION('center_axis',(-0.587785252279345,-2.26406643645659E-34,
0.809016994384486));
#112297=DIRECTION('ref_axis',(0.,1.,0.));
#112298=DIRECTION('center_axis',(-0.587785252279345,-2.26406643645659E-34,
0.809016994384486));
#112299=DIRECTION('ref_axis',(0.809016994384486,3.11622010999078E-34,0.587785252279345));
#112300=DIRECTION('center_axis',(0.587785252279345,2.26406643645659E-34,
-0.809016994384486));
#112301=DIRECTION('ref_axis',(3.85185988875507E-34,-1.,0.));
#112302=DIRECTION('center_axis',(-0.512899276931483,-1.97561615178386E-34,
0.858448793885321));
#112303=DIRECTION('ref_axis',(-3.85185988875507E-34,1.,0.));
#112304=DIRECTION('center_axis',(-0.512899276931483,-1.97561615178386E-34,
0.858448793885321));
#112305=DIRECTION('ref_axis',(0.858448793885321,3.30662447571703E-34,0.512899276931483));
#112306=DIRECTION('center_axis',(-0.512899276931483,-1.97561615178386E-34,
0.858448793885321));
#112307=DIRECTION('ref_axis',(0.,1.,0.));
#112308=DIRECTION('center_axis',(-0.512899276931483,-1.97561615178386E-34,
0.858448793885321));
#112309=DIRECTION('ref_axis',(0.858448793885321,3.30662447571703E-34,0.512899276931483));
#112310=DIRECTION('center_axis',(0.512899276931483,1.97561615178386E-34,
-0.858448793885321));
#112311=DIRECTION('ref_axis',(3.85185988875507E-34,-1.,0.));
#112312=DIRECTION('center_axis',(-0.433883738983985,-1.67125937057549E-34,
0.900968867966745));
#112313=DIRECTION('ref_axis',(-3.85185988875507E-34,1.,0.));
#112314=DIRECTION('center_axis',(-0.433883738983985,-1.67125937057549E-34,
0.900968867966745));
#112315=DIRECTION('ref_axis',(0.900968867966744,3.47040584353816E-34,0.433883738983985));
#112316=DIRECTION('center_axis',(-0.433883738983985,-1.67125937057549E-34,
0.900968867966745));
#112317=DIRECTION('ref_axis',(0.,1.,0.));
#112318=DIRECTION('center_axis',(-0.433883738983985,-1.67125937057549E-34,
0.900968867966745));
#112319=DIRECTION('ref_axis',(0.900968867966744,3.47040584353816E-34,0.433883738983985));
#112320=DIRECTION('center_axis',(0.433883738983985,1.67125937057549E-34,
-0.900968867966745));
#112321=DIRECTION('ref_axis',(3.85185988875507E-34,-1.,0.));
#112322=DIRECTION('center_axis',(-0.351374823891528,-1.35344659006615E-34,
0.936234870710976));
#112323=DIRECTION('ref_axis',(-3.85185988875507E-34,1.,0.));
#112324=DIRECTION('center_axis',(-0.351374823891528,-1.35344659006615E-34,
0.936234870710976));
#112325=DIRECTION('ref_axis',(0.936234870710976,3.60624554494539E-34,0.351374823891528));
#112326=DIRECTION('center_axis',(-0.351374823891528,-1.35344659006615E-34,
0.936234870710976));
#112327=DIRECTION('ref_axis',(0.,1.,0.));
#112328=DIRECTION('center_axis',(-0.351374823891528,-1.35344659006615E-34,
0.936234870710976));
#112329=DIRECTION('ref_axis',(0.936234870710976,3.60624554494539E-34,0.351374823891528));
#112330=DIRECTION('center_axis',(0.351374823891528,1.35344659006615E-34,
-0.936234870710976));
#112331=DIRECTION('ref_axis',(3.85185988875507E-34,-1.,0.));
#112332=DIRECTION('center_axis',(-0.266036845891333,-1.02473665561974E-34,
0.963962860606254));
#112333=DIRECTION('ref_axis',(-3.85185988875507E-34,1.,0.));
#112334=DIRECTION('center_axis',(-0.266036845891333,-1.02473665561974E-34,
0.963962860606254));
#112335=DIRECTION('ref_axis',(0.963962860606253,3.71304987701882E-34,0.266036845891333));
#112336=DIRECTION('center_axis',(-0.266036845891333,-1.02473665561974E-34,
0.963962860606254));
#112337=DIRECTION('ref_axis',(0.,1.,0.));
#112338=DIRECTION('center_axis',(-0.266036845891333,-1.02473665561974E-34,
0.963962860606254));
#112339=DIRECTION('ref_axis',(0.963962860606253,3.71304987701882E-34,0.266036845891333));
#112340=DIRECTION('center_axis',(0.266036845891333,1.02473665561974E-34,
-0.963962860606254));
#112341=DIRECTION('ref_axis',(3.85185988875507E-34,-1.,0.));
#112342=DIRECTION('center_axis',(-0.178556894923064,-6.87776141414805E-35,
0.98392958857605));
#112343=DIRECTION('ref_axis',(-3.85185988875507E-34,1.,0.));
#112344=DIRECTION('center_axis',(-0.178556894923064,-6.87776141414805E-35,
0.98392958857605));
#112345=DIRECTION('ref_axis',(0.983929588576049,3.78995891559536E-34,0.178556894923064));
#112346=DIRECTION('center_axis',(-0.178556894923064,-6.87776141414805E-35,
0.98392958857605));
#112347=DIRECTION('ref_axis',(0.,1.,0.));
#112348=DIRECTION('center_axis',(-0.178556894923064,-6.87776141414805E-35,
0.98392958857605));
#112349=DIRECTION('ref_axis',(0.983929588576049,3.78995891559536E-34,0.178556894923064));
#112350=DIRECTION('center_axis',(0.178556894923064,6.87776141414805E-35,
-0.98392958857605));
#112351=DIRECTION('ref_axis',(3.85185988875507E-34,-1.,0.));
#112352=DIRECTION('center_axis',(-0.089639308998799,-3.45278058788195E-35,
0.995974293986656));
#112353=DIRECTION('ref_axis',(-3.85185988875507E-34,1.,0.));
#112354=DIRECTION('center_axis',(-0.089639308998799,-3.45278058788195E-35,
0.995974293986656));
#112355=DIRECTION('ref_axis',(0.995974293986656,3.83635343323835E-34,0.089639308998799));
#112356=DIRECTION('center_axis',(-0.089639308998799,-3.45278058788195E-35,
0.995974293986656));
#112357=DIRECTION('ref_axis',(0.,1.,0.));
#112358=DIRECTION('center_axis',(-0.089639308998799,-3.45278058788195E-35,
0.995974293986656));
#112359=DIRECTION('ref_axis',(0.995974293986656,3.83635343323835E-34,0.089639308998799));
#112360=DIRECTION('center_axis',(0.089639308998799,3.45278058788195E-35,
-0.995974293986656));
#112361=DIRECTION('ref_axis',(3.85185988875507E-34,-1.,0.));
#112362=DIRECTION('center_axis',(0.,0.,1.));
#112363=DIRECTION('ref_axis',(-3.85185988875507E-34,1.,0.));
#112364=DIRECTION('center_axis',(0.,0.,1.));
#112365=DIRECTION('ref_axis',(1.,3.85185988875507E-34,0.));
#112366=DIRECTION('center_axis',(0.,0.,1.));
#112367=DIRECTION('ref_axis',(0.,1.,0.));
#112368=DIRECTION('center_axis',(0.,0.,1.));
#112369=DIRECTION('ref_axis',(1.,3.85185988875507E-34,0.));
#112370=DIRECTION('center_axis',(0.,0.,-1.));
#112371=DIRECTION('ref_axis',(3.85185988875507E-34,-1.,0.));
#112372=DIRECTION('center_axis',(0.089639308998799,3.45278058788195E-35,
0.995974293986656));
#112373=DIRECTION('ref_axis',(-3.85185988875507E-34,1.,0.));
#112374=DIRECTION('center_axis',(0.089639308998799,3.45278058788195E-35,
0.995974293986656));
#112375=DIRECTION('ref_axis',(0.995974293986656,3.83635343323835E-34,-0.089639308998799));
#112376=DIRECTION('center_axis',(0.089639308998799,3.45278058788195E-35,
0.995974293986656));
#112377=DIRECTION('ref_axis',(0.,1.,0.));
#112378=DIRECTION('center_axis',(0.089639308998799,3.45278058788195E-35,
0.995974293986656));
#112379=DIRECTION('ref_axis',(0.995974293986656,3.83635343323835E-34,-0.089639308998799));
#112380=DIRECTION('center_axis',(-0.089639308998799,-3.45278058788195E-35,
-0.995974293986656));
#112381=DIRECTION('ref_axis',(3.85185988875507E-34,-1.,0.));
#112382=DIRECTION('center_axis',(0.178556894923064,6.87776141414805E-35,
0.98392958857605));
#112383=DIRECTION('ref_axis',(-3.85185988875507E-34,1.,0.));
#112384=DIRECTION('center_axis',(0.178556894923064,6.87776141414805E-35,
0.98392958857605));
#112385=DIRECTION('ref_axis',(0.983929588576049,3.78995891559536E-34,-0.178556894923064));
#112386=DIRECTION('center_axis',(0.178556894923064,6.87776141414805E-35,
0.98392958857605));
#112387=DIRECTION('ref_axis',(0.,1.,0.));
#112388=DIRECTION('center_axis',(0.178556894923064,6.87776141414805E-35,
0.98392958857605));
#112389=DIRECTION('ref_axis',(0.983929588576049,3.78995891559536E-34,-0.178556894923064));
#112390=DIRECTION('center_axis',(-0.178556894923064,-6.87776141414805E-35,
-0.98392958857605));
#112391=DIRECTION('ref_axis',(3.85185988875507E-34,-1.,0.));
#112392=DIRECTION('center_axis',(0.266036845891333,1.02473665561974E-34,
0.963962860606254));
#112393=DIRECTION('ref_axis',(-3.85185988875507E-34,1.,0.));
#112394=DIRECTION('center_axis',(0.266036845891333,1.02473665561974E-34,
0.963962860606254));
#112395=DIRECTION('ref_axis',(0.963962860606253,3.71304987701882E-34,-0.266036845891333));
#112396=DIRECTION('center_axis',(0.266036845891333,1.02473665561974E-34,
0.963962860606254));
#112397=DIRECTION('ref_axis',(0.,1.,0.));
#112398=DIRECTION('center_axis',(0.266036845891333,1.02473665561974E-34,
0.963962860606254));
#112399=DIRECTION('ref_axis',(0.963962860606253,3.71304987701882E-34,-0.266036845891333));
#112400=DIRECTION('center_axis',(-0.266036845891333,-1.02473665561974E-34,
-0.963962860606254));
#112401=DIRECTION('ref_axis',(3.85185988875507E-34,-1.,0.));
#112402=DIRECTION('center_axis',(0.351374823891528,1.35344659006615E-34,
0.936234870710976));
#112403=DIRECTION('ref_axis',(-3.85185988875507E-34,1.,0.));
#112404=DIRECTION('center_axis',(0.351374823891528,1.35344659006615E-34,
0.936234870710976));
#112405=DIRECTION('ref_axis',(0.936234870710976,3.60624554494539E-34,-0.351374823891528));
#112406=DIRECTION('center_axis',(0.351374823891528,1.35344659006615E-34,
0.936234870710976));
#112407=DIRECTION('ref_axis',(0.,1.,0.));
#112408=DIRECTION('center_axis',(0.351374823891528,1.35344659006615E-34,
0.936234870710976));
#112409=DIRECTION('ref_axis',(0.936234870710976,3.60624554494539E-34,-0.351374823891528));
#112410=DIRECTION('center_axis',(-0.351374823891528,-1.35344659006615E-34,
-0.936234870710976));
#112411=DIRECTION('ref_axis',(3.85185988875507E-34,-1.,0.));
#112412=DIRECTION('center_axis',(0.433883738983985,1.67125937057549E-34,
0.900968867966745));
#112413=DIRECTION('ref_axis',(-3.85185988875507E-34,1.,0.));
#112414=DIRECTION('center_axis',(0.433883738983985,1.67125937057549E-34,
0.900968867966745));
#112415=DIRECTION('ref_axis',(0.900968867966744,3.47040584353816E-34,-0.433883738983985));
#112416=DIRECTION('center_axis',(0.433883738983985,1.67125937057549E-34,
0.900968867966745));
#112417=DIRECTION('ref_axis',(0.,1.,0.));
#112418=DIRECTION('center_axis',(0.433883738983985,1.67125937057549E-34,
0.900968867966745));
#112419=DIRECTION('ref_axis',(0.900968867966744,3.47040584353816E-34,-0.433883738983985));
#112420=DIRECTION('center_axis',(-0.433883738983985,-1.67125937057549E-34,
-0.900968867966745));
#112421=DIRECTION('ref_axis',(3.85185988875507E-34,-1.,0.));
#112422=DIRECTION('center_axis',(0.512899276931483,1.97561615178386E-34,
0.858448793885321));
#112423=DIRECTION('ref_axis',(-3.85185988875507E-34,1.,0.));
#112424=DIRECTION('center_axis',(0.512899276931483,1.97561615178386E-34,
0.858448793885321));
#112425=DIRECTION('ref_axis',(0.858448793885321,3.30662447571703E-34,-0.512899276931483));
#112426=DIRECTION('center_axis',(0.512899276931483,1.97561615178386E-34,
0.858448793885321));
#112427=DIRECTION('ref_axis',(0.,1.,0.));
#112428=DIRECTION('center_axis',(0.512899276931483,1.97561615178386E-34,
0.858448793885321));
#112429=DIRECTION('ref_axis',(0.858448793885321,3.30662447571703E-34,-0.512899276931483));
#112430=DIRECTION('center_axis',(-0.512899276931483,-1.97561615178386E-34,
-0.858448793885321));
#112431=DIRECTION('ref_axis',(3.85185988875507E-34,-1.,0.));
#112432=DIRECTION('center_axis',(0.587785252279345,2.26406643645659E-34,
0.809016994384486));
#112433=DIRECTION('ref_axis',(-3.85185988875507E-34,1.,0.));
#112434=DIRECTION('center_axis',(0.587785252279345,2.26406643645659E-34,
0.809016994384486));
#112435=DIRECTION('ref_axis',(0.809016994384486,3.11622010999078E-34,-0.587785252279345));
#112436=DIRECTION('center_axis',(0.587785252279345,2.26406643645659E-34,
0.809016994384486));
#112437=DIRECTION('ref_axis',(0.,1.,0.));
#112438=DIRECTION('center_axis',(0.587785252279345,2.26406643645659E-34,
0.809016994384486));
#112439=DIRECTION('ref_axis',(0.809016994384486,3.11622010999078E-34,-0.587785252279345));
#112440=DIRECTION('center_axis',(-0.587785252279345,-2.26406643645659E-34,
-0.809016994384486));
#112441=DIRECTION('ref_axis',(3.85185988875507E-34,-1.,0.));
#112442=DIRECTION('center_axis',(0.657938725975692,2.53428778784438E-34,
0.753071465972177));
#112443=DIRECTION('ref_axis',(-3.85185988875507E-34,1.,0.));
#112444=DIRECTION('center_axis',(0.657938725975692,2.53428778784438E-34,
0.753071465972177));
#112445=DIRECTION('ref_axis',(0.753071465972177,2.9007257731442E-34,-0.657938725975692));
#112446=DIRECTION('center_axis',(0.657938725975692,2.53428778784438E-34,
0.753071465972177));
#112447=DIRECTION('ref_axis',(0.,1.,0.));
#112448=DIRECTION('center_axis',(0.657938725975692,2.53428778784438E-34,
0.753071465972177));
#112449=DIRECTION('ref_axis',(0.753071465972177,2.9007257731442E-34,-0.657938725975692));
#112450=DIRECTION('center_axis',(-0.657938725975692,-2.53428778784438E-34,
-0.753071465972177));
#112451=DIRECTION('ref_axis',(3.85185988875507E-34,-1.,0.));
#112452=DIRECTION('center_axis',(0.722794863903263,2.78410454406716E-34,
0.69106264890751));
#112453=DIRECTION('ref_axis',(-3.85185988875507E-34,1.,0.));
#112454=DIRECTION('center_axis',(0.722794863903263,2.78410454406716E-34,
0.69106264890751));
#112455=DIRECTION('ref_axis',(0.69106264890751,2.66187649794366E-34,-0.722794863903263));
#112456=DIRECTION('center_axis',(0.722794863903263,2.78410454406716E-34,
0.69106264890751));
#112457=DIRECTION('ref_axis',(0.,1.,0.));
#112458=DIRECTION('center_axis',(0.722794863903263,2.78410454406716E-34,
0.69106264890751));
#112459=DIRECTION('ref_axis',(0.69106264890751,2.66187649794366E-34,-0.722794863903263));
#112460=DIRECTION('center_axis',(-0.722794863903263,-2.78410454406716E-34,
-0.69106264890751));
#112461=DIRECTION('ref_axis',(3.85185988875507E-34,-1.,0.));
#112462=DIRECTION('center_axis',(0.781831482217226,3.01150532611845E-34,
0.623489802173232));
#112463=DIRECTION('ref_axis',(-3.85185988875507E-34,1.,0.));
#112464=DIRECTION('center_axis',(0.781831482217226,3.01150532611845E-34,
0.623489802173232));
#112465=DIRECTION('ref_axis',(0.623489802173232,2.4015953600389E-34,-0.781831482217226));
#112466=DIRECTION('center_axis',(0.781831482217226,3.01150532611845E-34,
0.623489802173232));
#112467=DIRECTION('ref_axis',(0.,1.,0.));
#112468=DIRECTION('center_axis',(0.781831482217226,3.01150532611845E-34,
0.623489802173232));
#112469=DIRECTION('ref_axis',(0.623489802173232,2.4015953600389E-34,-0.781831482217226));
#112470=DIRECTION('center_axis',(-0.781831482217226,-3.01150532611845E-34,
-0.623489802173232));
#112471=DIRECTION('ref_axis',(3.85185988875507E-34,-1.,0.));
#112472=DIRECTION('center_axis',(0.834573254013744,3.21465924136334E-34,
0.550896981009072));
#112473=DIRECTION('ref_axis',(-3.85185988875507E-34,1.,0.));
#112474=DIRECTION('center_axis',(0.834573254013744,3.21465924136334E-34,
0.550896981009072));
#112475=DIRECTION('ref_axis',(0.550896981009072,2.12197798398511E-34,-0.834573254013744));
#112476=DIRECTION('center_axis',(0.834573254013744,3.21465924136334E-34,
0.550896981009072));
#112477=DIRECTION('ref_axis',(0.,1.,0.));
#112478=DIRECTION('center_axis',(0.834573254013744,3.21465924136334E-34,
0.550896981009072));
#112479=DIRECTION('ref_axis',(0.550896981009072,2.12197798398511E-34,-0.834573254013744));
#112480=DIRECTION('center_axis',(-0.834573254013744,-3.21465924136334E-34,
-0.550896981009072));
#112481=DIRECTION('ref_axis',(3.85185988875507E-34,-1.,0.));
#112482=DIRECTION('center_axis',(0.880595532086284,3.39193060826008E-34,
0.473868662046431));
#112483=DIRECTION('ref_axis',(-3.85185988875507E-34,1.,0.));
#112484=DIRECTION('center_axis',(0.880595532086284,3.39193060826008E-34,
0.473868662046431));
#112485=DIRECTION('ref_axis',(0.473868662046431,1.82527569187468E-34,-0.880595532086284));
#112486=DIRECTION('center_axis',(0.880595532086284,3.39193060826008E-34,
0.473868662046431));
#112487=DIRECTION('ref_axis',(0.,1.,0.));
#112488=DIRECTION('center_axis',(0.880595532086284,3.39193060826008E-34,
0.473868662046431));
#112489=DIRECTION('ref_axis',(0.473868662046431,1.82527569187468E-34,-0.880595532086284));
#112490=DIRECTION('center_axis',(-0.880595532086284,-3.39193060826008E-34,
-0.473868662046431));
#112491=DIRECTION('ref_axis',(3.85185988875507E-34,-1.,0.));
#112492=DIRECTION('center_axis',(0.919527772341198,3.54189214287736E-34,
0.393025032145835));
#112493=DIRECTION('ref_axis',(-3.85185988875507E-34,1.,0.));
#112494=DIRECTION('center_axis',(0.919527772341198,3.54189214287736E-34,
0.393025032145835));
#112495=DIRECTION('ref_axis',(0.393025032145835,1.51387735659921E-34,-0.919527772341198));
#112496=DIRECTION('center_axis',(0.919527772341198,3.54189214287736E-34,
0.393025032145835));
#112497=DIRECTION('ref_axis',(0.,1.,0.));
#112498=DIRECTION('center_axis',(0.919527772341198,3.54189214287736E-34,
0.393025032145835));
#112499=DIRECTION('ref_axis',(0.393025032145835,1.51387735659921E-34,-0.919527772341198));
#112500=DIRECTION('center_axis',(-0.919527772341198,-3.54189214287736E-34,
-0.393025032145835));
#112501=DIRECTION('ref_axis',(3.85185988875507E-34,-1.,0.));
#112502=DIRECTION('center_axis',(0.951056516377163,3.66333644737232E-34,
0.309016994122548));
#112503=DIRECTION('ref_axis',(-3.85185988875507E-34,1.,0.));
#112504=DIRECTION('center_axis',(0.951056516377163,3.66333644737232E-34,
0.309016994122548));
#112505=DIRECTION('ref_axis',(0.309016994122548,1.1902901646043E-34,-0.951056516377163));
#112506=DIRECTION('center_axis',(0.951056516377163,3.66333644737232E-34,
0.309016994122548));
#112507=DIRECTION('ref_axis',(0.,1.,0.));
#112508=DIRECTION('center_axis',(0.951056516377163,3.66333644737232E-34,
0.309016994122548));
#112509=DIRECTION('ref_axis',(0.309016994122548,1.1902901646043E-34,-0.951056516377163));
#112510=DIRECTION('center_axis',(-0.951056516377163,-3.66333644737232E-34,
-0.309016994122548));
#112511=DIRECTION('ref_axis',(3.85185988875507E-34,-1.,0.));
#112512=DIRECTION('center_axis',(0.974927912163343,3.75528571928971E-34,
0.222520934037282));
#112513=DIRECTION('ref_axis',(-3.85185988875507E-34,1.,0.));
#112514=DIRECTION('center_axis',(0.974927912163343,3.75528571928971E-34,
0.222520934037282));
#112515=DIRECTION('ref_axis',(0.222520934037282,8.57119460226519E-35,-0.974927912163343));
#112516=DIRECTION('center_axis',(0.974927912163343,3.75528571928971E-34,
0.222520934037282));
#112517=DIRECTION('ref_axis',(0.,1.,0.));
#112518=DIRECTION('center_axis',(0.974927912163343,3.75528571928971E-34,
0.222520934037282));
#112519=DIRECTION('ref_axis',(0.222520934037282,8.57119460226519E-35,-0.974927912163343));
#112520=DIRECTION('center_axis',(-0.974927912163343,-3.75528571928971E-34,
-0.222520934037282));
#112521=DIRECTION('ref_axis',(3.85185988875507E-34,-1.,0.));
#112522=DIRECTION('center_axis',(0.990949761747861,3.81699963904798E-34,
0.134233265965845));
#112523=DIRECTION('ref_axis',(-3.85185988875507E-34,1.,0.));
#112524=DIRECTION('center_axis',(0.990949761747861,3.81699963904798E-34,
0.134233265965845));
#112525=DIRECTION('ref_axis',(0.134233265965845,5.17047732910431E-35,-0.990949761747861));
#112526=DIRECTION('center_axis',(0.990949761747861,3.81699963904798E-34,
0.134233265965845));
#112527=DIRECTION('ref_axis',(0.,1.,0.));
#112528=DIRECTION('center_axis',(0.990949761747861,3.81699963904798E-34,
0.134233265965845));
#112529=DIRECTION('ref_axis',(0.134233265965845,5.17047732910431E-35,-0.990949761747861));
#112530=DIRECTION('center_axis',(-0.990949761747861,-3.81699963904798E-34,
-0.134233265965845));
#112531=DIRECTION('ref_axis',(3.85185988875507E-34,-1.,0.));
#112532=DIRECTION('center_axis',(0.998993066557948,3.84798132221898E-34,
0.0448648299801474));
#112533=DIRECTION('ref_axis',(-3.85185988875507E-34,1.,0.));
#112534=DIRECTION('center_axis',(0.998993066557948,3.84798132221898E-34,
0.0448648299801474));
#112535=DIRECTION('ref_axis',(0.0448648299801474,1.72813039016346E-35,-0.998993066557948));
#112536=DIRECTION('center_axis',(0.998993066557948,3.84798132221898E-34,
0.0448648299801474));
#112537=DIRECTION('ref_axis',(0.,1.,0.));
#112538=DIRECTION('center_axis',(0.998993066557948,3.84798132221898E-34,
0.0448648299801474));
#112539=DIRECTION('ref_axis',(0.0448648299801474,1.72813039016346E-35,-0.998993066557948));
#112540=DIRECTION('center_axis',(-0.998993066557948,-3.84798132221898E-34,
-0.0448648299801474));
#112541=DIRECTION('ref_axis',(3.85185988875507E-34,-1.,0.));
#112542=DIRECTION('center_axis',(0.998993066557948,3.84798132221898E-34,
-0.0448648299801474));
#112543=DIRECTION('ref_axis',(-3.85185988875507E-34,1.,0.));
#112544=DIRECTION('center_axis',(0.998993066557948,3.84798132221898E-34,
-0.0448648299801474));
#112545=DIRECTION('ref_axis',(-0.0448648299801474,-1.72813039016346E-35,
-0.998993066557948));
#112546=DIRECTION('center_axis',(0.998993066557948,3.84798132221898E-34,
-0.0448648299801474));
#112547=DIRECTION('ref_axis',(0.,1.,0.));
#112548=DIRECTION('center_axis',(0.998993066557948,3.84798132221898E-34,
-0.0448648299801474));
#112549=DIRECTION('ref_axis',(-0.0448648299801474,-1.72813039016346E-35,
-0.998993066557948));
#112550=DIRECTION('center_axis',(-0.998993066557948,-3.84798132221898E-34,
0.0448648299801474));
#112551=DIRECTION('ref_axis',(3.85185988875507E-34,-1.,0.));
#112552=DIRECTION('center_axis',(0.990949761747861,3.81699963904798E-34,
-0.134233265965845));
#112553=DIRECTION('ref_axis',(-3.85185988875507E-34,1.,0.));
#112554=DIRECTION('center_axis',(0.990949761747861,3.81699963904798E-34,
-0.134233265965845));
#112555=DIRECTION('ref_axis',(-0.134233265965845,-5.17047732910431E-35,
-0.990949761747861));
#112556=DIRECTION('center_axis',(0.990949761747861,3.81699963904798E-34,
-0.134233265965845));
#112557=DIRECTION('ref_axis',(0.,1.,0.));
#112558=DIRECTION('center_axis',(0.990949761747861,3.81699963904798E-34,
-0.134233265965845));
#112559=DIRECTION('ref_axis',(-0.134233265965845,-5.17047732910431E-35,
-0.990949761747861));
#112560=DIRECTION('center_axis',(-0.990949761747861,-3.81699963904798E-34,
0.134233265965845));
#112561=DIRECTION('ref_axis',(3.85185988875507E-34,-1.,0.));
#112562=DIRECTION('center_axis',(0.974927912163343,3.75528571928971E-34,
-0.222520934037282));
#112563=DIRECTION('ref_axis',(-3.85185988875507E-34,1.,0.));
#112564=DIRECTION('center_axis',(0.974927912163343,3.75528571928971E-34,
-0.222520934037282));
#112565=DIRECTION('ref_axis',(-0.222520934037282,-8.57119460226519E-35,
-0.974927912163343));
#112566=DIRECTION('center_axis',(0.974927912163343,3.75528571928971E-34,
-0.222520934037282));
#112567=DIRECTION('ref_axis',(0.,1.,0.));
#112568=DIRECTION('center_axis',(0.974927912163343,3.75528571928971E-34,
-0.222520934037282));
#112569=DIRECTION('ref_axis',(-0.222520934037282,-8.57119460226519E-35,
-0.974927912163343));
#112570=DIRECTION('center_axis',(-0.974927912163343,-3.75528571928971E-34,
0.222520934037282));
#112571=DIRECTION('ref_axis',(3.85185988875507E-34,-1.,0.));
#112572=DIRECTION('center_axis',(0.951056516377163,3.66333644737232E-34,
-0.309016994122548));
#112573=DIRECTION('ref_axis',(-3.85185988875507E-34,1.,0.));
#112574=DIRECTION('center_axis',(0.951056516377163,3.66333644737232E-34,
-0.309016994122548));
#112575=DIRECTION('ref_axis',(-0.309016994122548,-1.1902901646043E-34,-0.951056516377163));
#112576=DIRECTION('center_axis',(0.951056516377163,3.66333644737232E-34,
-0.309016994122548));
#112577=DIRECTION('ref_axis',(0.,1.,0.));
#112578=DIRECTION('center_axis',(0.951056516377163,3.66333644737232E-34,
-0.309016994122548));
#112579=DIRECTION('ref_axis',(-0.309016994122548,-1.1902901646043E-34,-0.951056516377163));
#112580=DIRECTION('center_axis',(-0.951056516377163,-3.66333644737232E-34,
0.309016994122548));
#112581=DIRECTION('ref_axis',(3.85185988875507E-34,-1.,0.));
#112582=DIRECTION('center_axis',(0.919527772341198,3.54189214287736E-34,
-0.393025032145835));
#112583=DIRECTION('ref_axis',(-3.85185988875507E-34,1.,0.));
#112584=DIRECTION('center_axis',(0.919527772341198,3.54189214287736E-34,
-0.393025032145835));
#112585=DIRECTION('ref_axis',(-0.393025032145835,-1.51387735659921E-34,
-0.919527772341198));
#112586=DIRECTION('center_axis',(0.919527772341198,3.54189214287736E-34,
-0.393025032145835));
#112587=DIRECTION('ref_axis',(0.,1.,0.));
#112588=DIRECTION('center_axis',(0.919527772341198,3.54189214287736E-34,
-0.393025032145835));
#112589=DIRECTION('ref_axis',(-0.393025032145835,-1.51387735659921E-34,
-0.919527772341198));
#112590=DIRECTION('center_axis',(-0.919527772341198,-3.54189214287736E-34,
0.393025032145835));
#112591=DIRECTION('ref_axis',(3.85185988875507E-34,-1.,0.));
#112592=DIRECTION('center_axis',(0.880595532086284,3.39193060826008E-34,
-0.473868662046431));
#112593=DIRECTION('ref_axis',(-3.85185988875507E-34,1.,0.));
#112594=DIRECTION('center_axis',(0.880595532086284,3.39193060826008E-34,
-0.473868662046431));
#112595=DIRECTION('ref_axis',(-0.473868662046431,-1.82527569187468E-34,
-0.880595532086284));
#112596=DIRECTION('center_axis',(0.880595532086284,3.39193060826008E-34,
-0.473868662046431));
#112597=DIRECTION('ref_axis',(0.,1.,0.));
#112598=DIRECTION('center_axis',(0.880595532086284,3.39193060826008E-34,
-0.473868662046431));
#112599=DIRECTION('ref_axis',(-0.473868662046431,-1.82527569187468E-34,
-0.880595532086284));
#112600=DIRECTION('center_axis',(-0.880595532086284,-3.39193060826008E-34,
0.473868662046431));
#112601=DIRECTION('ref_axis',(3.85185988875507E-34,-1.,0.));
#112602=DIRECTION('center_axis',(0.834573254013744,3.21465924136334E-34,
-0.550896981009072));
#112603=DIRECTION('ref_axis',(-3.85185988875507E-34,1.,0.));
#112604=DIRECTION('center_axis',(0.834573254013744,3.21465924136334E-34,
-0.550896981009072));
#112605=DIRECTION('ref_axis',(-0.550896981009072,-2.12197798398511E-34,
-0.834573254013744));
#112606=DIRECTION('center_axis',(0.834573254013744,3.21465924136334E-34,
-0.550896981009072));
#112607=DIRECTION('ref_axis',(0.,1.,0.));
#112608=DIRECTION('center_axis',(0.834573254013744,3.21465924136334E-34,
-0.550896981009072));
#112609=DIRECTION('ref_axis',(-0.550896981009072,-2.12197798398511E-34,
-0.834573254013744));
#112610=DIRECTION('center_axis',(-0.834573254013744,-3.21465924136334E-34,
0.550896981009072));
#112611=DIRECTION('ref_axis',(3.85185988875507E-34,-1.,0.));
#112612=DIRECTION('center_axis',(0.781831482217226,3.01150532611845E-34,
-0.623489802173232));
#112613=DIRECTION('ref_axis',(-3.85185988875507E-34,1.,0.));
#112614=DIRECTION('center_axis',(0.781831482217226,3.01150532611845E-34,
-0.623489802173232));
#112615=DIRECTION('ref_axis',(-0.623489802173232,-2.4015953600389E-34,-0.781831482217226));
#112616=DIRECTION('center_axis',(0.781831482217226,3.01150532611845E-34,
-0.623489802173232));
#112617=DIRECTION('ref_axis',(0.,1.,0.));
#112618=DIRECTION('center_axis',(0.781831482217226,3.01150532611845E-34,
-0.623489802173232));
#112619=DIRECTION('ref_axis',(-0.623489802173232,-2.4015953600389E-34,-0.781831482217226));
#112620=DIRECTION('center_axis',(-0.781831482217226,-3.01150532611845E-34,
0.623489802173232));
#112621=DIRECTION('ref_axis',(3.85185988875507E-34,-1.,0.));
#112622=DIRECTION('center_axis',(0.722794863903263,2.78410454406716E-34,
-0.69106264890751));
#112623=DIRECTION('ref_axis',(-3.85185988875507E-34,1.,0.));
#112624=DIRECTION('center_axis',(0.722794863903263,2.78410454406716E-34,
-0.69106264890751));
#112625=DIRECTION('ref_axis',(-0.69106264890751,-2.66187649794366E-34,-0.722794863903263));
#112626=DIRECTION('center_axis',(0.722794863903263,2.78410454406716E-34,
-0.69106264890751));
#112627=DIRECTION('ref_axis',(0.,1.,0.));
#112628=DIRECTION('center_axis',(0.722794863903263,2.78410454406716E-34,
-0.69106264890751));
#112629=DIRECTION('ref_axis',(-0.69106264890751,-2.66187649794366E-34,-0.722794863903263));
#112630=DIRECTION('center_axis',(-0.722794863903263,-2.78410454406716E-34,
0.69106264890751));
#112631=DIRECTION('ref_axis',(3.85185988875507E-34,-1.,0.));
#112632=DIRECTION('center_axis',(0.657938725975692,2.53428778784438E-34,
-0.753071465972177));
#112633=DIRECTION('ref_axis',(-3.85185988875507E-34,1.,0.));
#112634=DIRECTION('center_axis',(0.657938725975692,2.53428778784438E-34,
-0.753071465972177));
#112635=DIRECTION('ref_axis',(-0.753071465972177,-2.9007257731442E-34,-0.657938725975692));
#112636=DIRECTION('center_axis',(0.657938725975692,2.53428778784438E-34,
-0.753071465972177));
#112637=DIRECTION('ref_axis',(0.,1.,0.));
#112638=DIRECTION('center_axis',(0.657938725975692,2.53428778784438E-34,
-0.753071465972177));
#112639=DIRECTION('ref_axis',(-0.753071465972177,-2.9007257731442E-34,-0.657938725975692));
#112640=DIRECTION('center_axis',(-0.657938725975692,-2.53428778784438E-34,
0.753071465972177));
#112641=DIRECTION('ref_axis',(3.85185988875507E-34,-1.,0.));
#112642=DIRECTION('center_axis',(0.587785252279345,2.26406643645659E-34,
-0.809016994384486));
#112643=DIRECTION('ref_axis',(-3.85185988875507E-34,1.,0.));
#112644=DIRECTION('center_axis',(0.587785252279345,2.26406643645659E-34,
-0.809016994384486));
#112645=DIRECTION('ref_axis',(-0.809016994384486,-3.11622010999078E-34,
-0.587785252279345));
#112646=DIRECTION('center_axis',(0.587785252279345,2.26406643645659E-34,
-0.809016994384486));
#112647=DIRECTION('ref_axis',(0.,1.,0.));
#112648=DIRECTION('center_axis',(0.587785252279345,2.26406643645659E-34,
-0.809016994384486));
#112649=DIRECTION('ref_axis',(-0.809016994384486,-3.11622010999078E-34,
-0.587785252279345));
#112650=DIRECTION('center_axis',(-0.587785252279345,-2.26406643645659E-34,
0.809016994384486));
#112651=DIRECTION('ref_axis',(3.85185988875507E-34,-1.,0.));
#112652=DIRECTION('center_axis',(0.512899276931483,1.97561615178386E-34,
-0.858448793885321));
#112653=DIRECTION('ref_axis',(-3.85185988875507E-34,1.,0.));
#112654=DIRECTION('center_axis',(0.512899276931483,1.97561615178386E-34,
-0.858448793885321));
#112655=DIRECTION('ref_axis',(-0.858448793885321,-3.30662447571703E-34,
-0.512899276931483));
#112656=DIRECTION('center_axis',(0.512899276931483,1.97561615178386E-34,
-0.858448793885321));
#112657=DIRECTION('ref_axis',(0.,1.,0.));
#112658=DIRECTION('center_axis',(0.512899276931483,1.97561615178386E-34,
-0.858448793885321));
#112659=DIRECTION('ref_axis',(-0.858448793885321,-3.30662447571703E-34,
-0.512899276931483));
#112660=DIRECTION('center_axis',(-0.512899276931483,-1.97561615178386E-34,
0.858448793885321));
#112661=DIRECTION('ref_axis',(3.85185988875507E-34,-1.,0.));
#112662=DIRECTION('center_axis',(0.433883738983985,1.67125937057549E-34,
-0.900968867966745));
#112663=DIRECTION('ref_axis',(-3.85185988875507E-34,1.,0.));
#112664=DIRECTION('center_axis',(0.433883738983985,1.67125937057549E-34,
-0.900968867966745));
#112665=DIRECTION('ref_axis',(-0.900968867966744,-3.47040584353816E-34,
-0.433883738983985));
#112666=DIRECTION('center_axis',(0.433883738983985,1.67125937057549E-34,
-0.900968867966745));
#112667=DIRECTION('ref_axis',(0.,1.,0.));
#112668=DIRECTION('center_axis',(0.433883738983985,1.67125937057549E-34,
-0.900968867966745));
#112669=DIRECTION('ref_axis',(-0.900968867966744,-3.47040584353816E-34,
-0.433883738983985));
#112670=DIRECTION('center_axis',(-0.433883738983985,-1.67125937057549E-34,
0.900968867966745));
#112671=DIRECTION('ref_axis',(3.85185988875507E-34,-1.,0.));
#112672=DIRECTION('center_axis',(0.351374823891528,1.35344659006615E-34,
-0.936234870710976));
#112673=DIRECTION('ref_axis',(-3.85185988875507E-34,1.,0.));
#112674=DIRECTION('center_axis',(0.351374823891528,1.35344659006615E-34,
-0.936234870710976));
#112675=DIRECTION('ref_axis',(-0.936234870710976,-3.60624554494539E-34,
-0.351374823891528));
#112676=DIRECTION('center_axis',(0.351374823891528,1.35344659006615E-34,
-0.936234870710976));
#112677=DIRECTION('ref_axis',(0.,1.,0.));
#112678=DIRECTION('center_axis',(0.351374823891528,1.35344659006615E-34,
-0.936234870710976));
#112679=DIRECTION('ref_axis',(-0.936234870710976,-3.60624554494539E-34,
-0.351374823891528));
#112680=DIRECTION('center_axis',(-0.351374823891528,-1.35344659006615E-34,
0.936234870710976));
#112681=DIRECTION('ref_axis',(3.85185988875507E-34,-1.,0.));
#112682=DIRECTION('center_axis',(0.266036845891333,1.02473665561974E-34,
-0.963962860606254));
#112683=DIRECTION('ref_axis',(-3.85185988875507E-34,1.,0.));
#112684=DIRECTION('center_axis',(0.266036845891333,1.02473665561974E-34,
-0.963962860606254));
#112685=DIRECTION('ref_axis',(-0.963962860606253,-3.71304987701882E-34,
-0.266036845891333));
#112686=DIRECTION('center_axis',(0.266036845891333,1.02473665561974E-34,
-0.963962860606254));
#112687=DIRECTION('ref_axis',(0.,1.,0.));
#112688=DIRECTION('center_axis',(0.266036845891333,1.02473665561974E-34,
-0.963962860606254));
#112689=DIRECTION('ref_axis',(-0.963962860606253,-3.71304987701882E-34,
-0.266036845891333));
#112690=DIRECTION('center_axis',(-0.266036845891333,-1.02473665561974E-34,
0.963962860606254));
#112691=DIRECTION('ref_axis',(3.85185988875507E-34,-1.,0.));
#112692=DIRECTION('center_axis',(0.178556894923064,6.87776141414805E-35,
-0.98392958857605));
#112693=DIRECTION('ref_axis',(-3.85185988875507E-34,1.,0.));
#112694=DIRECTION('center_axis',(0.178556894923064,6.87776141414805E-35,
-0.98392958857605));
#112695=DIRECTION('ref_axis',(-0.983929588576049,-3.78995891559536E-34,
-0.178556894923064));
#112696=DIRECTION('center_axis',(0.178556894923064,6.87776141414805E-35,
-0.98392958857605));
#112697=DIRECTION('ref_axis',(0.,1.,0.));
#112698=DIRECTION('center_axis',(0.178556894923064,6.87776141414805E-35,
-0.98392958857605));
#112699=DIRECTION('ref_axis',(-0.983929588576049,-3.78995891559536E-34,
-0.178556894923064));
#112700=DIRECTION('center_axis',(-0.178556894923064,-6.87776141414805E-35,
0.98392958857605));
#112701=DIRECTION('ref_axis',(3.85185988875507E-34,-1.,0.));
#112702=DIRECTION('center_axis',(0.089639308998799,3.45278058788195E-35,
-0.995974293986656));
#112703=DIRECTION('ref_axis',(-3.85185988875507E-34,1.,0.));
#112704=DIRECTION('center_axis',(0.089639308998799,3.45278058788195E-35,
-0.995974293986656));
#112705=DIRECTION('ref_axis',(-0.995974293986656,-3.83635343323835E-34,
-0.089639308998799));
#112706=DIRECTION('center_axis',(0.089639308998799,3.45278058788195E-35,
-0.995974293986656));
#112707=DIRECTION('ref_axis',(0.,1.,0.));
#112708=DIRECTION('center_axis',(0.089639308998799,3.45278058788195E-35,
-0.995974293986656));
#112709=DIRECTION('ref_axis',(-0.995974293986656,-3.83635343323835E-34,
-0.089639308998799));
#112710=DIRECTION('center_axis',(-0.089639308998799,-3.45278058788195E-35,
0.995974293986656));
#112711=DIRECTION('ref_axis',(3.85185988875507E-34,-1.,0.));
#112712=DIRECTION('center_axis',(-3.85185988875507E-34,1.,0.));
#112713=DIRECTION('ref_axis',(1.,3.85185988875507E-34,0.));
#112714=DIRECTION('center_axis',(-3.85185988875507E-34,1.,0.));
#112715=DIRECTION('ref_axis',(0.,0.,1.));
#112716=DIRECTION('',(-3.85185988875507E-34,1.,0.));
#112717=DIRECTION('center_axis',(-3.85185988875507E-34,1.,0.));
#112718=DIRECTION('ref_axis',(0.,0.,1.));
#112719=DIRECTION('center_axis',(-3.85185988875507E-34,1.,0.));
#112720=DIRECTION('ref_axis',(1.,3.85185988875507E-34,0.));
#112721=DIRECTION('center_axis',(-3.85185988875507E-34,1.,0.));
#112722=DIRECTION('ref_axis',(0.,0.,1.));
#112723=DIRECTION('',(-3.85185988875507E-34,1.,0.));
#112724=DIRECTION('center_axis',(-3.85185988875507E-34,1.,0.));
#112725=DIRECTION('ref_axis',(0.,0.,1.));
#112726=DIRECTION('center_axis',(-3.85185988875507E-34,1.,0.));
#112727=DIRECTION('ref_axis',(1.,0.,0.));
#112728=DIRECTION('center_axis',(-3.85185988875507E-34,1.,0.));
#112729=DIRECTION('ref_axis',(0.,0.,1.));
#112730=DIRECTION('center_axis',(-1.22464679914735E-16,-4.71716788352798E-50,
-1.));
#112731=DIRECTION('ref_axis',(-1.,0.,1.22464679914735E-16));
#112732=DIRECTION('center_axis',(3.85185988875507E-34,-1.,0.));
#112733=DIRECTION('ref_axis',(0.,0.,1.));
#112734=DIRECTION('center_axis',(-3.85185988875507E-34,1.,0.));
#112735=DIRECTION('ref_axis',(1.,0.,0.));
#112736=DIRECTION('center_axis',(-3.85185988875507E-34,1.,0.));
#112737=DIRECTION('ref_axis',(0.,0.,1.));
#112738=DIRECTION('center_axis',(-1.22464679914735E-16,-4.71716788352798E-50,
-1.));
#112739=DIRECTION('ref_axis',(-1.,0.,1.22464679914735E-16));
#112740=DIRECTION('center_axis',(3.85185988875507E-34,-1.,0.));
#112741=DIRECTION('ref_axis',(0.,0.,1.));
#112742=DIRECTION('center_axis',(3.85185988875507E-34,-1.,0.));
#112743=DIRECTION('ref_axis',(-1.,0.,0.));
#112744=DIRECTION('center_axis',(3.85185988875507E-34,-1.,0.));
#112745=DIRECTION('ref_axis',(0.,0.,1.));
#112746=DIRECTION('center_axis',(-1.22464679914735E-16,-4.71716788352798E-50,
1.));
#112747=DIRECTION('ref_axis',(1.,0.,1.22464679914735E-16));
#112748=DIRECTION('center_axis',(-3.85185988875507E-34,1.,0.));
#112749=DIRECTION('ref_axis',(0.,0.,-1.));
#112750=DIRECTION('center_axis',(3.85185988875507E-34,-1.,0.));
#112751=DIRECTION('ref_axis',(0.,0.,1.));
#112752=DIRECTION('center_axis',(-3.85185988875507E-34,1.,0.));
#112753=DIRECTION('ref_axis',(1.,0.,0.));
#112754=DIRECTION('center_axis',(-3.85185988875507E-34,1.,0.));
#112755=DIRECTION('ref_axis',(0.,0.,1.));
#112756=DIRECTION('center_axis',(1.22464679914735E-16,4.71716788352798E-50,
1.));
#112757=DIRECTION('ref_axis',(-1.,0.,1.22464679914735E-16));
#112758=DIRECTION('center_axis',(3.85185988875507E-34,-1.,0.));
#112759=DIRECTION('ref_axis',(0.,0.,1.));
#112760=DIRECTION('center_axis',(-3.85185988875507E-34,1.,0.));
#112761=DIRECTION('ref_axis',(1.,0.,0.));
#112762=DIRECTION('center_axis',(-3.85185988875507E-34,1.,0.));
#112763=DIRECTION('ref_axis',(0.,0.,1.));
#112764=DIRECTION('center_axis',(1.22464679914735E-16,4.71716788352798E-50,
1.));
#112765=DIRECTION('ref_axis',(-1.,0.,1.22464679914735E-16));
#112766=DIRECTION('center_axis',(3.85185988875507E-34,-1.,0.));
#112767=DIRECTION('ref_axis',(0.,0.,-1.));
#112768=DIRECTION('center_axis',(3.85185988875507E-34,-1.,0.));
#112769=DIRECTION('ref_axis',(0.,0.,-1.));
#112770=DIRECTION('center_axis',(-3.85185988875507E-34,1.,0.));
#112771=DIRECTION('ref_axis',(1.,0.,0.));
#112772=DIRECTION('center_axis',(3.85185988875507E-34,-1.,0.));
#112773=DIRECTION('ref_axis',(0.,0.,-1.));
#112774=DIRECTION('center_axis',(0.942809041733257,3.63156833060794E-34,
0.333333332905692));
#112775=DIRECTION('ref_axis',(0.333333332905692,1.28395329460448E-34,-0.942809041733257));
#112776=DIRECTION('center_axis',(-3.85185988875507E-34,1.,0.));
#112777=DIRECTION('ref_axis',(0.,0.,1.));
#112778=DIRECTION('center_axis',(-0.388215488117679,-1.49535166687396E-34,
0.921568627279354));
#112779=DIRECTION('ref_axis',(0.921568627279354,3.54975323015241E-34,0.388215488117679));
#112780=DIRECTION('center_axis',(-3.85185988875507E-34,1.,0.));
#112781=DIRECTION('ref_axis',(1.,0.,0.));
#112782=DIRECTION('center_axis',(3.85185988875507E-34,-1.,0.));
#112783=DIRECTION('ref_axis',(0.,0.,-1.));
#112784=DIRECTION('center_axis',(0.388215488966968,1.4953516701453E-34,
0.921568626921586));
#112785=DIRECTION('ref_axis',(0.921568626921586,3.54975322877434E-34,-0.388215488966968));
#112786=DIRECTION('center_axis',(-3.85185988875507E-34,1.,0.));
#112787=DIRECTION('ref_axis',(0.,0.,1.));
#112788=DIRECTION('center_axis',(-0.942809041733257,-3.63156833060794E-34,
0.333333332905692));
#112789=DIRECTION('ref_axis',(0.333333332905692,1.28395329460448E-34,0.942809041733257));
#112790=DIRECTION('center_axis',(-3.85185988875507E-34,1.,0.));
#112791=DIRECTION('ref_axis',(1.,0.,0.));
#112792=DIRECTION('center_axis',(-3.85185988875507E-34,1.,0.));
#112793=DIRECTION('ref_axis',(0.,0.,1.));
#112794=DIRECTION('center_axis',(1.22464679914735E-16,4.71716788352797E-50,
1.));
#112795=DIRECTION('ref_axis',(-1.,0.,1.22464679914735E-16));
#112796=DIRECTION('center_axis',(3.85185988875507E-34,-1.,0.));
#112797=DIRECTION('ref_axis',(0.,0.,-1.));
#112798=DIRECTION('center_axis',(3.85185988875507E-34,-1.,0.));
#112799=DIRECTION('ref_axis',(0.,0.,-1.));
#112800=DIRECTION('center_axis',(3.85185988875507E-34,-1.,0.));
#112801=DIRECTION('ref_axis',(-1.,0.,0.));
#112802=DIRECTION('center_axis',(3.85185988875507E-34,-1.,0.));
#112803=DIRECTION('ref_axis',(0.,0.,-1.));
#112804=DIRECTION('center_axis',(-1.22464679914735E-16,-4.71716788352797E-50,
1.));
#112805=DIRECTION('ref_axis',(1.,0.,1.22464679914735E-16));
#112806=DIRECTION('center_axis',(-3.85185988875507E-34,1.,0.));
#112807=DIRECTION('ref_axis',(0.,0.,1.));
#112808=DIRECTION('center_axis',(-3.85185988875507E-34,1.,0.));
#112809=DIRECTION('ref_axis',(0.,0.,1.));
#112810=DIRECTION('center_axis',(3.85185988875507E-34,-1.,0.));
#112811=DIRECTION('ref_axis',(-1.,0.,0.));
#112812=DIRECTION('center_axis',(3.85185988875507E-34,-1.,0.));
#112813=DIRECTION('ref_axis',(0.,0.,-1.));
#112814=DIRECTION('center_axis',(-1.22464679914735E-16,-4.71716788352797E-50,
1.));
#112815=DIRECTION('ref_axis',(1.,0.,1.22464679914735E-16));
#112816=DIRECTION('center_axis',(-3.85185988875507E-34,1.,0.));
#112817=DIRECTION('ref_axis',(0.,0.,1.));
#112818=DIRECTION('center_axis',(-3.85185988875507E-34,1.,0.));
#112819=DIRECTION('ref_axis',(0.,0.,1.));
#112820=DIRECTION('center_axis',(3.85185988875507E-34,-1.,0.));
#112821=DIRECTION('ref_axis',(-1.,-3.85185988875507E-34,0.));
#112822=DIRECTION('center_axis',(3.85185988875507E-34,-1.,0.));
#112823=DIRECTION('ref_axis',(0.,0.,-1.));
#112824=DIRECTION('',(3.85185988875507E-34,-1.,0.));
#112825=DIRECTION('center_axis',(-3.85185988875507E-34,1.,0.));
#112826=DIRECTION('ref_axis',(0.,0.,-1.));
#112827=DIRECTION('',(3.85185988875507E-34,-1.,0.));
#112828=DIRECTION('center_axis',(3.85185988875507E-34,-1.,0.));
#112829=DIRECTION('ref_axis',(-1.,-3.85185988875507E-34,0.));
#112830=DIRECTION('center_axis',(3.85185988875507E-34,-1.,0.));
#112831=DIRECTION('ref_axis',(0.,0.,-1.));
#112832=DIRECTION('',(3.85185988875507E-34,-1.,0.));
#112833=DIRECTION('center_axis',(-3.85185988875507E-34,1.,0.));
#112834=DIRECTION('ref_axis',(0.,0.,-1.));
#112835=DIRECTION('',(3.85185988875507E-34,-1.,0.));
#112836=DIRECTION('center_axis',(3.85185988875507E-34,-1.,0.));
#112837=DIRECTION('ref_axis',(-1.,-3.85185988875507E-34,0.));
#112838=DIRECTION('center_axis',(3.85185988875507E-34,-1.,0.));
#112839=DIRECTION('ref_axis',(0.,0.,-1.));
#112840=DIRECTION('',(3.85185988875507E-34,-1.,0.));
#112841=DIRECTION('center_axis',(-3.85185988875507E-34,1.,0.));
#112842=DIRECTION('ref_axis',(1.,3.85185988875507E-34,0.));
#112843=DIRECTION('',(3.85185988875507E-34,-1.,0.));
#112844=DIRECTION('center_axis',(-3.85185988875507E-34,1.,0.));
#112845=DIRECTION('ref_axis',(1.,3.85185988875507E-34,0.));
#112846=DIRECTION('',(3.85185988875507E-34,-1.,0.));
#112847=DIRECTION('center_axis',(3.85185988875507E-34,-1.,0.));
#112848=DIRECTION('ref_axis',(-1.,-3.85185988875507E-34,0.));
#112849=DIRECTION('center_axis',(-3.85185988875507E-34,1.,0.));
#112850=DIRECTION('ref_axis',(0.,0.,-1.));
#112851=DIRECTION('',(-3.85185988875507E-34,1.,0.));
#112852=DIRECTION('center_axis',(-3.85185988875507E-34,1.,0.));
#112853=DIRECTION('ref_axis',(1.,3.85185988875507E-34,0.));
#112854=DIRECTION('center_axis',(-3.85185988875507E-34,1.,0.));
#112855=DIRECTION('ref_axis',(0.,0.,1.));
#112856=DIRECTION('',(-3.85185988875507E-34,1.,0.));
#112857=DIRECTION('center_axis',(-3.85185988875507E-34,1.,0.));
#112858=DIRECTION('ref_axis',(0.,0.,1.));
#112859=DIRECTION('',(-3.85185988875507E-34,1.,0.));
#112860=DIRECTION('center_axis',(-3.85185988875507E-34,1.,0.));
#112861=DIRECTION('ref_axis',(1.,3.85185988875507E-34,0.));
#112862=DIRECTION('center_axis',(-3.85185988875507E-34,1.,0.));
#112863=DIRECTION('ref_axis',(0.,0.,1.));
#112864=DIRECTION('',(-3.85185988875507E-34,1.,0.));
#112865=DIRECTION('center_axis',(-3.85185988875507E-34,1.,0.));
#112866=DIRECTION('ref_axis',(0.,0.,1.));
#112867=DIRECTION('',(-3.85185988875507E-34,1.,0.));
#112868=DIRECTION('center_axis',(-3.85185988875507E-34,1.,0.));
#112869=DIRECTION('ref_axis',(1.,3.85185988875507E-34,0.));
#112870=DIRECTION('center_axis',(-3.85185988875507E-34,1.,0.));
#112871=DIRECTION('ref_axis',(0.,0.,1.));
#112872=DIRECTION('',(-3.85185988875507E-34,1.,0.));
#112873=DIRECTION('center_axis',(3.85185988875507E-34,-1.,0.));
#112874=DIRECTION('ref_axis',(0.,0.,1.));
#112875=DIRECTION('',(3.85185988875507E-34,-1.,0.));
#112876=DIRECTION('center_axis',(-3.85185988875507E-34,1.,0.));
#112877=DIRECTION('ref_axis',(1.,3.85185988875507E-34,0.));
#112878=DIRECTION('center_axis',(-3.85185988875507E-34,1.,0.));
#112879=DIRECTION('ref_axis',(0.,0.,1.));
#112880=DIRECTION('',(-3.85185988875507E-34,1.,0.));
#112881=DIRECTION('center_axis',(3.85185988875507E-34,-1.,0.));
#112882=DIRECTION('ref_axis',(0.,0.,1.));
#112883=DIRECTION('',(3.85185988875507E-34,-1.,0.));
#112884=DIRECTION('center_axis',(-3.85185988875507E-34,1.,0.));
#112885=DIRECTION('ref_axis',(1.,3.85185988875507E-34,0.));
#112886=DIRECTION('',(-3.85185988875507E-34,1.,0.));
#112887=DIRECTION('center_axis',(-3.85185988875507E-34,1.,0.));
#112888=DIRECTION('ref_axis',(1.,3.85185988875507E-34,0.));
#112889=DIRECTION('center_axis',(-3.85185988875507E-34,1.,0.));
#112890=DIRECTION('ref_axis',(0.,0.,1.));
#112891=DIRECTION('center_axis',(-3.85185988875507E-34,1.,0.));
#112892=DIRECTION('ref_axis',(0.,0.,1.));
#112893=DIRECTION('center_axis',(-3.85185988875507E-34,1.,0.));
#112894=DIRECTION('ref_axis',(0.,0.,1.));
#112895=DIRECTION('center_axis',(-3.85185988875507E-34,1.,0.));
#112896=DIRECTION('ref_axis',(0.,0.,1.));
#112897=DIRECTION('center_axis',(-3.85185988875507E-34,1.,0.));
#112898=DIRECTION('ref_axis',(0.,0.,1.));
#112899=DIRECTION('center_axis',(-3.85185988875507E-34,1.,0.));
#112900=DIRECTION('ref_axis',(0.,0.,1.));
#112901=DIRECTION('center_axis',(-3.85185988875507E-34,1.,0.));
#112902=DIRECTION('ref_axis',(0.,0.,1.));
#112903=DIRECTION('center_axis',(-3.85185988875507E-34,1.,0.));
#112904=DIRECTION('ref_axis',(0.,0.,1.));
#112905=DIRECTION('center_axis',(-3.85185988875507E-34,1.,0.));
#112906=DIRECTION('ref_axis',(0.,0.,1.));
#112907=DIRECTION('center_axis',(-3.85185988875507E-34,1.,0.));
#112908=DIRECTION('ref_axis',(0.,0.,1.));
#112909=DIRECTION('center_axis',(-3.85185988875507E-34,1.,0.));
#112910=DIRECTION('ref_axis',(0.,0.,1.));
#112911=DIRECTION('center_axis',(-3.85185988875507E-34,1.,0.));
#112912=DIRECTION('ref_axis',(0.,0.,1.));
#112913=DIRECTION('center_axis',(-3.85185988875507E-34,1.,0.));
#112914=DIRECTION('ref_axis',(0.,0.,1.));
#112915=DIRECTION('center_axis',(-3.85185988875507E-34,1.,0.));
#112916=DIRECTION('ref_axis',(0.,0.,1.));
#112917=DIRECTION('center_axis',(-3.85185988875507E-34,1.,0.));
#112918=DIRECTION('ref_axis',(0.,0.,1.));
#112919=DIRECTION('center_axis',(-3.85185988875507E-34,1.,0.));
#112920=DIRECTION('ref_axis',(0.,0.,1.));
#112921=DIRECTION('center_axis',(-3.85185988875507E-34,1.,0.));
#112922=DIRECTION('ref_axis',(0.,0.,1.));
#112923=DIRECTION('center_axis',(-3.85185988875507E-34,1.,0.));
#112924=DIRECTION('ref_axis',(0.,0.,1.));
#112925=DIRECTION('center_axis',(-3.85185988875507E-34,1.,0.));
#112926=DIRECTION('ref_axis',(0.,0.,1.));
#112927=DIRECTION('center_axis',(-3.85185988875507E-34,1.,0.));
#112928=DIRECTION('ref_axis',(0.,0.,1.));
#112929=DIRECTION('center_axis',(-3.85185988875507E-34,1.,0.));
#112930=DIRECTION('ref_axis',(0.,0.,1.));
#112931=DIRECTION('center_axis',(-3.85185988875507E-34,1.,0.));
#112932=DIRECTION('ref_axis',(0.,0.,1.));
#112933=DIRECTION('center_axis',(-3.85185988875507E-34,1.,0.));
#112934=DIRECTION('ref_axis',(0.,0.,1.));
#112935=DIRECTION('center_axis',(-3.85185988875507E-34,1.,0.));
#112936=DIRECTION('ref_axis',(0.,0.,1.));
#112937=DIRECTION('center_axis',(-3.85185988875507E-34,1.,0.));
#112938=DIRECTION('ref_axis',(0.,0.,1.));
#112939=DIRECTION('center_axis',(-3.85185988875507E-34,1.,0.));
#112940=DIRECTION('ref_axis',(0.,0.,1.));
#112941=DIRECTION('center_axis',(-3.85185988875507E-34,1.,0.));
#112942=DIRECTION('ref_axis',(0.,0.,1.));
#112943=DIRECTION('center_axis',(-3.85185988875507E-34,1.,0.));
#112944=DIRECTION('ref_axis',(0.,0.,1.));
#112945=DIRECTION('center_axis',(-3.85185988875507E-34,1.,0.));
#112946=DIRECTION('ref_axis',(0.,0.,1.));
#112947=DIRECTION('center_axis',(-3.85185988875507E-34,1.,0.));
#112948=DIRECTION('ref_axis',(0.,0.,1.));
#112949=DIRECTION('center_axis',(-3.85185988875507E-34,1.,0.));
#112950=DIRECTION('ref_axis',(0.,0.,1.));
#112951=DIRECTION('center_axis',(-3.85185988875507E-34,1.,0.));
#112952=DIRECTION('ref_axis',(0.,0.,1.));
#112953=DIRECTION('center_axis',(-3.85185988875507E-34,1.,0.));
#112954=DIRECTION('ref_axis',(0.,0.,1.));
#112955=DIRECTION('center_axis',(-3.85185988875507E-34,1.,0.));
#112956=DIRECTION('ref_axis',(0.,0.,1.));
#112957=DIRECTION('center_axis',(-3.85185988875507E-34,1.,0.));
#112958=DIRECTION('ref_axis',(0.,0.,1.));
#112959=DIRECTION('center_axis',(-3.85185988875507E-34,1.,0.));
#112960=DIRECTION('ref_axis',(0.,0.,1.));
#112961=DIRECTION('center_axis',(-3.85185988875507E-34,1.,0.));
#112962=DIRECTION('ref_axis',(0.,0.,1.));
#112963=DIRECTION('center_axis',(-3.85185988875507E-34,1.,0.));
#112964=DIRECTION('ref_axis',(0.,0.,1.));
#112965=DIRECTION('center_axis',(-3.85185988875507E-34,1.,0.));
#112966=DIRECTION('ref_axis',(0.,0.,1.));
#112967=DIRECTION('center_axis',(-3.85185988875507E-34,1.,0.));
#112968=DIRECTION('ref_axis',(0.,0.,1.));
#112969=DIRECTION('center_axis',(-3.85185988875507E-34,1.,0.));
#112970=DIRECTION('ref_axis',(0.,0.,1.));
#112971=DIRECTION('center_axis',(-3.85185988875507E-34,1.,0.));
#112972=DIRECTION('ref_axis',(0.,0.,1.));
#112973=DIRECTION('center_axis',(-3.85185988875507E-34,1.,0.));
#112974=DIRECTION('ref_axis',(0.,0.,1.));
#112975=DIRECTION('center_axis',(-3.85185988875507E-34,1.,0.));
#112976=DIRECTION('ref_axis',(0.,0.,1.));
#112977=DIRECTION('center_axis',(-3.85185988875507E-34,1.,0.));
#112978=DIRECTION('ref_axis',(0.,0.,1.));
#112979=DIRECTION('center_axis',(-3.85185988875507E-34,1.,0.));
#112980=DIRECTION('ref_axis',(0.,0.,1.));
#112981=DIRECTION('center_axis',(-3.85185988875507E-34,1.,0.));
#112982=DIRECTION('ref_axis',(0.,0.,1.));
#112983=DIRECTION('center_axis',(-3.85185988875507E-34,1.,0.));
#112984=DIRECTION('ref_axis',(0.,0.,1.));
#112985=DIRECTION('center_axis',(-3.85185988875507E-34,1.,0.));
#112986=DIRECTION('ref_axis',(0.,0.,1.));
#112987=DIRECTION('center_axis',(-3.85185988875507E-34,1.,0.));
#112988=DIRECTION('ref_axis',(0.,0.,1.));
#112989=DIRECTION('center_axis',(-3.85185988875507E-34,1.,0.));
#112990=DIRECTION('ref_axis',(0.,0.,1.));
#112991=DIRECTION('center_axis',(-3.85185988875507E-34,1.,0.));
#112992=DIRECTION('ref_axis',(0.,0.,1.));
#112993=DIRECTION('center_axis',(-3.85185988875507E-34,1.,0.));
#112994=DIRECTION('ref_axis',(0.,0.,1.));
#112995=DIRECTION('center_axis',(-3.85185988875507E-34,1.,0.));
#112996=DIRECTION('ref_axis',(0.,0.,1.));
#112997=DIRECTION('center_axis',(-3.85185988875507E-34,1.,0.));
#112998=DIRECTION('ref_axis',(0.,0.,1.));
#112999=DIRECTION('center_axis',(-3.85185988875507E-34,1.,0.));
#113000=DIRECTION('ref_axis',(0.,0.,1.));
#113001=DIRECTION('center_axis',(-3.85185988875507E-34,1.,0.));
#113002=DIRECTION('ref_axis',(0.,0.,1.));
#113003=DIRECTION('center_axis',(-3.85185988875507E-34,1.,0.));
#113004=DIRECTION('ref_axis',(0.,0.,1.));
#113005=DIRECTION('center_axis',(-3.85185988875507E-34,1.,0.));
#113006=DIRECTION('ref_axis',(0.,0.,1.));
#113007=DIRECTION('center_axis',(-3.85185988875507E-34,1.,0.));
#113008=DIRECTION('ref_axis',(0.,0.,1.));
#113009=DIRECTION('center_axis',(-3.85185988875507E-34,1.,0.));
#113010=DIRECTION('ref_axis',(0.,0.,1.));
#113011=DIRECTION('center_axis',(-3.85185988875507E-34,1.,0.));
#113012=DIRECTION('ref_axis',(0.,0.,1.));
#113013=DIRECTION('center_axis',(-3.85185988875507E-34,1.,0.));
#113014=DIRECTION('ref_axis',(0.,0.,1.));
#113015=DIRECTION('center_axis',(-3.85185988875507E-34,1.,0.));
#113016=DIRECTION('ref_axis',(0.,0.,1.));
#113017=DIRECTION('center_axis',(-3.85185988875507E-34,1.,0.));
#113018=DIRECTION('ref_axis',(0.,0.,1.));
#113019=DIRECTION('center_axis',(-3.85185988875507E-34,1.,0.));
#113020=DIRECTION('ref_axis',(0.,0.,1.));
#113021=DIRECTION('center_axis',(-3.85185988875507E-34,1.,0.));
#113022=DIRECTION('ref_axis',(0.,0.,1.));
#113023=DIRECTION('center_axis',(-3.85185988875507E-34,1.,0.));
#113024=DIRECTION('ref_axis',(0.,0.,1.));
#113025=DIRECTION('center_axis',(-3.85185988875507E-34,1.,0.));
#113026=DIRECTION('ref_axis',(0.,0.,1.));
#113027=DIRECTION('center_axis',(-3.85185988875507E-34,1.,0.));
#113028=DIRECTION('ref_axis',(0.,0.,1.));
#113029=DIRECTION('center_axis',(-3.85185988875507E-34,1.,0.));
#113030=DIRECTION('ref_axis',(0.,0.,1.));
#113031=DIRECTION('center_axis',(-3.85185988875507E-34,1.,0.));
#113032=DIRECTION('ref_axis',(0.,0.,1.));
#113033=DIRECTION('center_axis',(-3.85185988875507E-34,1.,0.));
#113034=DIRECTION('ref_axis',(0.,0.,1.));
#113035=DIRECTION('center_axis',(-3.85185988875507E-34,1.,0.));
#113036=DIRECTION('ref_axis',(0.,0.,1.));
#113037=DIRECTION('center_axis',(-3.85185988875507E-34,1.,0.));
#113038=DIRECTION('ref_axis',(0.,0.,1.));
#113039=DIRECTION('center_axis',(-3.85185988875507E-34,1.,0.));
#113040=DIRECTION('ref_axis',(0.,0.,1.));
#113041=DIRECTION('center_axis',(-3.85185988875507E-34,1.,0.));
#113042=DIRECTION('ref_axis',(0.,0.,1.));
#113043=DIRECTION('center_axis',(-3.85185988875507E-34,1.,0.));
#113044=DIRECTION('ref_axis',(0.,0.,1.));
#113045=DIRECTION('center_axis',(-3.85185988875507E-34,1.,0.));
#113046=DIRECTION('ref_axis',(0.,0.,1.));
#113047=DIRECTION('center_axis',(-3.85185988875507E-34,1.,0.));
#113048=DIRECTION('ref_axis',(0.,0.,1.));
#113049=DIRECTION('center_axis',(-3.85185988875507E-34,1.,0.));
#113050=DIRECTION('ref_axis',(0.,0.,1.));
#113051=DIRECTION('center_axis',(-3.85185988875507E-34,1.,0.));
#113052=DIRECTION('ref_axis',(0.,0.,1.));
#113053=DIRECTION('center_axis',(-3.85185988875507E-34,1.,0.));
#113054=DIRECTION('ref_axis',(0.,0.,1.));
#113055=DIRECTION('center_axis',(-3.85185988875507E-34,1.,0.));
#113056=DIRECTION('ref_axis',(0.,0.,1.));
#113057=DIRECTION('center_axis',(-3.85185988875507E-34,1.,0.));
#113058=DIRECTION('ref_axis',(0.,0.,1.));
#113059=DIRECTION('center_axis',(-3.85185988875507E-34,1.,0.));
#113060=DIRECTION('ref_axis',(0.,0.,1.));
#113061=DIRECTION('center_axis',(-3.85185988875507E-34,1.,0.));
#113062=DIRECTION('ref_axis',(0.,0.,1.));
#113063=DIRECTION('center_axis',(-3.85185988875507E-34,1.,0.));
#113064=DIRECTION('ref_axis',(0.,0.,1.));
#113065=DIRECTION('center_axis',(-3.85185988875507E-34,1.,0.));
#113066=DIRECTION('ref_axis',(0.,0.,1.));
#113067=DIRECTION('center_axis',(-3.85185988875507E-34,1.,0.));
#113068=DIRECTION('ref_axis',(0.,0.,1.));
#113069=DIRECTION('center_axis',(-3.85185988875507E-34,1.,0.));
#113070=DIRECTION('ref_axis',(0.,0.,1.));
#113071=DIRECTION('center_axis',(-3.85185988875507E-34,1.,0.));
#113072=DIRECTION('ref_axis',(0.,0.,1.));
#113073=DIRECTION('center_axis',(-3.85185988875507E-34,1.,0.));
#113074=DIRECTION('ref_axis',(0.,0.,1.));
#113075=DIRECTION('center_axis',(-3.85185988875507E-34,1.,0.));
#113076=DIRECTION('ref_axis',(0.,0.,1.));
#113077=DIRECTION('center_axis',(-3.85185988875507E-34,1.,0.));
#113078=DIRECTION('ref_axis',(0.,0.,1.));
#113079=DIRECTION('center_axis',(-3.85185988875507E-34,1.,0.));
#113080=DIRECTION('ref_axis',(0.,0.,1.));
#113081=DIRECTION('center_axis',(-3.85185988875507E-34,1.,0.));
#113082=DIRECTION('ref_axis',(0.,0.,1.));
#113083=DIRECTION('center_axis',(-3.85185988875507E-34,1.,0.));
#113084=DIRECTION('ref_axis',(0.,0.,1.));
#113085=DIRECTION('center_axis',(-3.85185988875507E-34,1.,0.));
#113086=DIRECTION('ref_axis',(0.,0.,1.));
#113087=DIRECTION('center_axis',(-3.85185988875507E-34,1.,0.));
#113088=DIRECTION('ref_axis',(0.,0.,1.));
#113089=DIRECTION('center_axis',(-3.85185988875507E-34,1.,0.));
#113090=DIRECTION('ref_axis',(0.,0.,1.));
#113091=DIRECTION('center_axis',(-3.85185988875507E-34,1.,0.));
#113092=DIRECTION('ref_axis',(0.,0.,1.));
#113093=DIRECTION('center_axis',(-3.85185988875507E-34,1.,0.));
#113094=DIRECTION('ref_axis',(0.,0.,1.));
#113095=DIRECTION('center_axis',(-3.85185988875507E-34,1.,0.));
#113096=DIRECTION('ref_axis',(0.,0.,1.));
#113097=DIRECTION('center_axis',(-3.85185988875507E-34,1.,0.));
#113098=DIRECTION('ref_axis',(0.,0.,1.));
#113099=DIRECTION('center_axis',(-3.85185988875507E-34,1.,0.));
#113100=DIRECTION('ref_axis',(0.,0.,1.));
#113101=DIRECTION('center_axis',(-3.85185988875507E-34,1.,0.));
#113102=DIRECTION('ref_axis',(0.,0.,1.));
#113103=DIRECTION('center_axis',(-3.85185988875507E-34,1.,0.));
#113104=DIRECTION('ref_axis',(0.,0.,1.));
#113105=DIRECTION('center_axis',(-3.85185988875507E-34,1.,0.));
#113106=DIRECTION('ref_axis',(0.,0.,1.));
#113107=DIRECTION('center_axis',(-3.85185988875507E-34,1.,0.));
#113108=DIRECTION('ref_axis',(0.,0.,1.));
#113109=DIRECTION('center_axis',(-3.85185988875507E-34,1.,0.));
#113110=DIRECTION('ref_axis',(0.,0.,1.));
#113111=DIRECTION('center_axis',(-3.85185988875507E-34,1.,0.));
#113112=DIRECTION('ref_axis',(0.,0.,1.));
#113113=DIRECTION('center_axis',(-3.85185988875507E-34,1.,0.));
#113114=DIRECTION('ref_axis',(0.,0.,1.));
#113115=DIRECTION('center_axis',(-3.85185988875507E-34,1.,0.));
#113116=DIRECTION('ref_axis',(0.,0.,1.));
#113117=DIRECTION('center_axis',(-3.85185988875507E-34,1.,0.));
#113118=DIRECTION('ref_axis',(0.,0.,1.));
#113119=DIRECTION('center_axis',(-3.85185988875507E-34,1.,0.));
#113120=DIRECTION('ref_axis',(0.,0.,1.));
#113121=DIRECTION('center_axis',(-3.85185988875507E-34,1.,0.));
#113122=DIRECTION('ref_axis',(0.,0.,1.));
#113123=DIRECTION('center_axis',(-3.85185988875507E-34,1.,0.));
#113124=DIRECTION('ref_axis',(0.,0.,1.));
#113125=DIRECTION('center_axis',(-3.85185988875507E-34,1.,0.));
#113126=DIRECTION('ref_axis',(0.,0.,1.));
#113127=DIRECTION('center_axis',(-3.85185988875507E-34,1.,0.));
#113128=DIRECTION('ref_axis',(0.,0.,1.));
#113129=DIRECTION('center_axis',(-3.85185988875507E-34,1.,0.));
#113130=DIRECTION('ref_axis',(0.,0.,1.));
#113131=DIRECTION('center_axis',(-3.85185988875507E-34,1.,0.));
#113132=DIRECTION('ref_axis',(0.,0.,1.));
#113133=DIRECTION('center_axis',(-3.85185988875507E-34,1.,0.));
#113134=DIRECTION('ref_axis',(0.,0.,1.));
#113135=DIRECTION('center_axis',(-3.85185988875507E-34,1.,0.));
#113136=DIRECTION('ref_axis',(0.,0.,1.));
#113137=DIRECTION('center_axis',(-3.85185988875507E-34,1.,0.));
#113138=DIRECTION('ref_axis',(0.,0.,1.));
#113139=DIRECTION('center_axis',(-3.85185988875507E-34,1.,0.));
#113140=DIRECTION('ref_axis',(0.,0.,1.));
#113141=DIRECTION('center_axis',(-3.85185988875507E-34,1.,0.));
#113142=DIRECTION('ref_axis',(0.,0.,1.));
#113143=DIRECTION('center_axis',(-3.85185988875507E-34,1.,0.));
#113144=DIRECTION('ref_axis',(0.,0.,1.));
#113145=DIRECTION('center_axis',(-3.85185988875507E-34,1.,0.));
#113146=DIRECTION('ref_axis',(0.,0.,1.));
#113147=DIRECTION('center_axis',(-3.85185988875507E-34,1.,0.));
#113148=DIRECTION('ref_axis',(0.,0.,1.));
#113149=DIRECTION('center_axis',(-3.85185988875507E-34,1.,0.));
#113150=DIRECTION('ref_axis',(0.,0.,1.));
#113151=DIRECTION('center_axis',(-3.85185988875507E-34,1.,0.));
#113152=DIRECTION('ref_axis',(0.,0.,1.));
#113153=DIRECTION('center_axis',(-3.85185988875507E-34,1.,0.));
#113154=DIRECTION('ref_axis',(0.,0.,1.));
#113155=DIRECTION('center_axis',(-3.85185988875507E-34,1.,0.));
#113156=DIRECTION('ref_axis',(0.,0.,1.));
#113157=DIRECTION('center_axis',(-3.85185988875507E-34,1.,0.));
#113158=DIRECTION('ref_axis',(0.,0.,1.));
#113159=DIRECTION('center_axis',(-3.85185988875507E-34,1.,0.));
#113160=DIRECTION('ref_axis',(0.,0.,1.));
#113161=DIRECTION('center_axis',(-3.85185988875507E-34,1.,0.));
#113162=DIRECTION('ref_axis',(0.,0.,1.));
#113163=DIRECTION('center_axis',(-3.85185988875507E-34,1.,0.));
#113164=DIRECTION('ref_axis',(0.,0.,1.));
#113165=DIRECTION('center_axis',(-3.85185988875507E-34,1.,0.));
#113166=DIRECTION('ref_axis',(0.,0.,1.));
#113167=DIRECTION('center_axis',(-3.85185988875507E-34,1.,0.));
#113168=DIRECTION('ref_axis',(0.,0.,1.));
#113169=DIRECTION('center_axis',(-3.85185988875507E-34,1.,0.));
#113170=DIRECTION('ref_axis',(0.,0.,1.));
#113171=DIRECTION('center_axis',(-3.85185988875507E-34,1.,0.));
#113172=DIRECTION('ref_axis',(0.,0.,1.));
#113173=DIRECTION('center_axis',(-3.85185988875507E-34,1.,0.));
#113174=DIRECTION('ref_axis',(0.,0.,1.));
#113175=DIRECTION('center_axis',(-3.85185988875507E-34,1.,0.));
#113176=DIRECTION('ref_axis',(0.,0.,1.));
#113177=DIRECTION('center_axis',(3.85185988875507E-34,-1.,0.));
#113178=DIRECTION('ref_axis',(0.,0.,1.));
#113179=DIRECTION('center_axis',(-3.85185988875507E-34,1.,0.));
#113180=DIRECTION('ref_axis',(0.,0.,1.));
#113181=DIRECTION('',(0.942809041733257,3.63156833060794E-34,-0.333333332905692));
#113182=DIRECTION('center_axis',(-3.85185988875507E-34,1.,0.));
#113183=DIRECTION('ref_axis',(0.,0.,1.));
#113184=DIRECTION('center_axis',(-3.85185988875507E-34,1.,0.));
#113185=DIRECTION('ref_axis',(0.,0.,1.));
#113186=DIRECTION('',(0.942809041733257,3.63156833060794E-34,0.333333332905692));
#113187=DIRECTION('center_axis',(-3.85185988875507E-34,1.,0.));
#113188=DIRECTION('ref_axis',(0.,0.,1.));
#113189=DIRECTION('',(-0.942809041733257,-3.63156833060794E-34,0.333333332905692));
#113190=DIRECTION('center_axis',(-3.85185988875507E-34,1.,0.));
#113191=DIRECTION('ref_axis',(0.,0.,1.));
#113192=DIRECTION('center_axis',(-3.85185988875507E-34,1.,0.));
#113193=DIRECTION('ref_axis',(0.,0.,1.));
#113194=DIRECTION('',(-0.942809041733257,-3.63156833060794E-34,-0.333333332905692));
#113195=DIRECTION('center_axis',(-3.85185988875507E-34,1.,0.));
#113196=DIRECTION('ref_axis',(0.,0.,1.));
#113197=DIRECTION('center_axis',(3.85185988875507E-34,-1.,0.));
#113198=DIRECTION('ref_axis',(0.,0.,1.));
#113199=DIRECTION('center_axis',(-3.85185988875507E-34,1.,0.));
#113200=DIRECTION('ref_axis',(0.,0.,1.));
#113201=DIRECTION('center_axis',(-3.85185988875507E-34,1.,0.));
#113202=DIRECTION('ref_axis',(1.,3.85185988875507E-34,0.));
#113203=DIRECTION('',(-3.85185988875507E-34,1.,0.));
#113204=DIRECTION('',(3.85185988875507E-34,-1.,0.));
#113205=DIRECTION('center_axis',(-3.85185988875507E-34,1.,0.));
#113206=DIRECTION('ref_axis',(0.,0.,1.));
#113207=DIRECTION('center_axis',(-3.85185988875507E-34,1.,0.));
#113208=DIRECTION('ref_axis',(1.,3.85185988875507E-34,0.));
#113209=DIRECTION('',(3.85185988875507E-34,-1.,0.));
#113210=DIRECTION('center_axis',(-3.85185988875507E-34,1.,0.));
#113211=DIRECTION('ref_axis',(0.,0.,1.));
#113212=DIRECTION('',(-3.85185988875507E-34,1.,0.));
#113213=DIRECTION('center_axis',(-3.85185988875507E-34,1.,0.));
#113214=DIRECTION('ref_axis',(1.,3.85185988875507E-34,0.));
#113215=DIRECTION('',(-3.85185988875507E-34,1.,0.));
#113216=DIRECTION('',(3.85185988875507E-34,-1.,0.));
#113217=DIRECTION('center_axis',(-3.85185988875507E-34,1.,0.));
#113218=DIRECTION('ref_axis',(0.,0.,1.));
#113219=DIRECTION('center_axis',(-3.85185988875507E-34,1.,0.));
#113220=DIRECTION('ref_axis',(1.,3.85185988875507E-34,0.));
#113221=DIRECTION('',(-3.85185988875507E-34,1.,0.));
#113222=DIRECTION('',(3.85185988875507E-34,-1.,0.));
#113223=DIRECTION('center_axis',(-3.85185988875507E-34,1.,0.));
#113224=DIRECTION('ref_axis',(0.,0.,1.));
#113225=DIRECTION('center_axis',(-3.85185988875507E-34,1.,0.));
#113226=DIRECTION('ref_axis',(1.,3.85185988875507E-34,0.));
#113227=DIRECTION('',(-3.85185988875507E-34,1.,0.));
#113228=DIRECTION('',(3.85185988875507E-34,-1.,0.));
#113229=DIRECTION('center_axis',(-3.85185988875507E-34,1.,0.));
#113230=DIRECTION('ref_axis',(0.,0.,1.));
#113231=DIRECTION('center_axis',(-3.85185988875507E-34,1.,0.));
#113232=DIRECTION('ref_axis',(1.,3.85185988875507E-34,0.));
#113233=DIRECTION('',(3.85185988875507E-34,-1.,0.));
#113234=DIRECTION('center_axis',(-3.85185988875507E-34,1.,0.));
#113235=DIRECTION('ref_axis',(0.,0.,1.));
#113236=DIRECTION('center_axis',(-3.85185988875507E-34,1.,0.));
#113237=DIRECTION('ref_axis',(1.,3.85185988875507E-34,0.));
#113238=DIRECTION('',(3.85185988875507E-34,-1.,0.));
#113239=DIRECTION('center_axis',(-3.85185988875507E-34,1.,0.));
#113240=DIRECTION('ref_axis',(0.,0.,1.));
#113241=DIRECTION('center_axis',(-3.85185988875507E-34,1.,0.));
#113242=DIRECTION('ref_axis',(1.,3.85185988875507E-34,0.));
#113243=DIRECTION('',(3.85185988875507E-34,-1.,0.));
#113244=DIRECTION('center_axis',(-3.85185988875507E-34,1.,0.));
#113245=DIRECTION('ref_axis',(0.,0.,1.));
#113246=DIRECTION('',(-3.85185988875507E-34,1.,0.));
#113247=DIRECTION('center_axis',(-3.85185988875507E-34,1.,0.));
#113248=DIRECTION('ref_axis',(1.,3.85185988875507E-34,0.));
#113249=DIRECTION('',(-3.85185988875507E-34,1.,0.));
#113250=DIRECTION('',(3.85185988875507E-34,-1.,0.));
#113251=DIRECTION('center_axis',(-3.85185988875507E-34,1.,0.));
#113252=DIRECTION('ref_axis',(0.,0.,1.));
#113253=DIRECTION('center_axis',(-3.85185988875507E-34,1.,0.));
#113254=DIRECTION('ref_axis',(1.,3.85185988875507E-34,0.));
#113255=DIRECTION('',(-3.85185988875507E-34,1.,0.));
#113256=DIRECTION('',(3.85185988875507E-34,-1.,0.));
#113257=DIRECTION('center_axis',(-3.85185988875507E-34,1.,0.));
#113258=DIRECTION('ref_axis',(0.,0.,1.));
#113259=DIRECTION('center_axis',(-3.85185988875507E-34,1.,0.));
#113260=DIRECTION('ref_axis',(1.,3.85185988875507E-34,0.));
#113261=DIRECTION('',(3.85185988875507E-34,-1.,0.));
#113262=DIRECTION('center_axis',(-3.85185988875507E-34,1.,0.));
#113263=DIRECTION('ref_axis',(0.,0.,1.));
#113264=DIRECTION('',(-3.85185988875507E-34,1.,0.));
#113265=DIRECTION('center_axis',(-3.85185988875507E-34,1.,0.));
#113266=DIRECTION('ref_axis',(1.,3.85185988875507E-34,0.));
#113267=DIRECTION('',(-3.85185988875507E-34,1.,0.));
#113268=DIRECTION('',(3.85185988875507E-34,-1.,0.));
#113269=DIRECTION('center_axis',(-3.85185988875507E-34,1.,0.));
#113270=DIRECTION('ref_axis',(0.,0.,1.));
#113271=DIRECTION('center_axis',(-3.85185988875507E-34,1.,0.));
#113272=DIRECTION('ref_axis',(1.,3.85185988875507E-34,0.));
#113273=DIRECTION('center_axis',(-3.85185988875507E-34,1.,0.));
#113274=DIRECTION('ref_axis',(0.,0.,1.));
#113275=DIRECTION('',(-3.85185988875507E-34,1.,0.));
#113276=DIRECTION('center_axis',(-3.85185988875507E-34,1.,0.));
#113277=DIRECTION('ref_axis',(1.,3.85185988875507E-34,0.));
#113278=DIRECTION('center_axis',(-3.85185988875507E-34,1.,0.));
#113279=DIRECTION('ref_axis',(0.,0.,1.));
#113280=DIRECTION('',(-3.85185988875507E-34,1.,0.));
#113281=DIRECTION('center_axis',(-3.85185988875507E-34,1.,0.));
#113282=DIRECTION('ref_axis',(1.,3.85185988875507E-34,0.));
#113283=DIRECTION('',(3.85185988875507E-34,-1.,0.));
#113284=DIRECTION('center_axis',(-3.85185988875507E-34,1.,0.));
#113285=DIRECTION('ref_axis',(0.,0.,1.));
#113286=DIRECTION('',(-3.85185988875507E-34,1.,0.));
#113287=DIRECTION('center_axis',(-3.85185988875507E-34,1.,0.));
#113288=DIRECTION('ref_axis',(1.,3.85185988875507E-34,0.));
#113289=DIRECTION('',(-3.85185988875507E-34,1.,0.));
#113290=DIRECTION('',(3.85185988875507E-34,-1.,0.));
#113291=DIRECTION('center_axis',(-3.85185988875507E-34,1.,0.));
#113292=DIRECTION('ref_axis',(0.,0.,1.));
#113293=DIRECTION('center_axis',(-3.85185988875507E-34,1.,0.));
#113294=DIRECTION('ref_axis',(1.,3.85185988875507E-34,0.));
#113295=DIRECTION('',(3.85185988875507E-34,-1.,0.));
#113296=DIRECTION('center_axis',(-3.85185988875507E-34,1.,0.));
#113297=DIRECTION('ref_axis',(0.,0.,1.));
#113298=DIRECTION('',(-3.85185988875507E-34,1.,0.));
#113299=DIRECTION('center_axis',(-3.85185988875507E-34,1.,0.));
#113300=DIRECTION('ref_axis',(1.,3.85185988875507E-34,0.));
#113301=DIRECTION('',(-3.85185988875507E-34,1.,0.));
#113302=DIRECTION('',(3.85185988875507E-34,-1.,0.));
#113303=DIRECTION('center_axis',(-3.85185988875507E-34,1.,0.));
#113304=DIRECTION('ref_axis',(0.,0.,1.));
#113305=DIRECTION('center_axis',(-3.85185988875507E-34,1.,0.));
#113306=DIRECTION('ref_axis',(1.,3.85185988875507E-34,0.));
#113307=DIRECTION('',(-3.85185988875507E-34,1.,0.));
#113308=DIRECTION('',(3.85185988875507E-34,-1.,0.));
#113309=DIRECTION('center_axis',(-3.85185988875507E-34,1.,0.));
#113310=DIRECTION('ref_axis',(0.,0.,1.));
#113311=DIRECTION('center_axis',(-3.85185988875507E-34,1.,0.));
#113312=DIRECTION('ref_axis',(1.,3.85185988875507E-34,0.));
#113313=DIRECTION('',(3.85185988875507E-34,-1.,0.));
#113314=DIRECTION('center_axis',(-3.85185988875507E-34,1.,0.));
#113315=DIRECTION('ref_axis',(0.,0.,1.));
#113316=DIRECTION('',(-3.85185988875507E-34,1.,0.));
#113317=DIRECTION('center_axis',(-3.85185988875507E-34,1.,0.));
#113318=DIRECTION('ref_axis',(1.,3.85185988875507E-34,0.));
#113319=DIRECTION('',(-3.85185988875507E-34,1.,0.));
#113320=DIRECTION('',(3.85185988875507E-34,-1.,0.));
#113321=DIRECTION('center_axis',(-3.85185988875507E-34,1.,0.));
#113322=DIRECTION('ref_axis',(0.,0.,1.));
#113323=DIRECTION('center_axis',(-3.85185988875507E-34,1.,0.));
#113324=DIRECTION('ref_axis',(1.,3.85185988875507E-34,0.));
#113325=DIRECTION('',(3.85185988875507E-34,-1.,0.));
#113326=DIRECTION('center_axis',(-3.85185988875507E-34,1.,0.));
#113327=DIRECTION('ref_axis',(0.,0.,1.));
#113328=DIRECTION('',(-3.85185988875507E-34,1.,0.));
#113329=DIRECTION('center_axis',(-3.85185988875507E-34,1.,0.));
#113330=DIRECTION('ref_axis',(1.,3.85185988875507E-34,0.));
#113331=DIRECTION('',(3.85185988875507E-34,-1.,0.));
#113332=DIRECTION('center_axis',(-3.85185988875507E-34,1.,0.));
#113333=DIRECTION('ref_axis',(0.,0.,1.));
#113334=DIRECTION('',(-3.85185988875507E-34,1.,0.));
#113335=DIRECTION('center_axis',(-3.85185988875507E-34,1.,0.));
#113336=DIRECTION('ref_axis',(1.,3.85185988875507E-34,0.));
#113337=DIRECTION('',(3.85185988875507E-34,-1.,0.));
#113338=DIRECTION('center_axis',(-3.85185988875507E-34,1.,0.));
#113339=DIRECTION('ref_axis',(0.,0.,1.));
#113340=DIRECTION('',(-3.85185988875507E-34,1.,0.));
#113341=DIRECTION('center_axis',(-3.85185988875507E-34,1.,0.));
#113342=DIRECTION('ref_axis',(1.,3.85185988875507E-34,0.));
#113343=DIRECTION('',(-3.85185988875507E-34,1.,0.));
#113344=DIRECTION('',(3.85185988875507E-34,-1.,0.));
#113345=DIRECTION('center_axis',(-3.85185988875507E-34,1.,0.));
#113346=DIRECTION('ref_axis',(0.,0.,1.));
#113347=DIRECTION('center_axis',(-3.85185988875507E-34,1.,0.));
#113348=DIRECTION('ref_axis',(1.,3.85185988875507E-34,0.));
#113349=DIRECTION('',(3.85185988875507E-34,-1.,0.));
#113350=DIRECTION('center_axis',(-3.85185988875507E-34,1.,0.));
#113351=DIRECTION('ref_axis',(0.,0.,1.));
#113352=DIRECTION('',(-3.85185988875507E-34,1.,0.));
#113353=DIRECTION('center_axis',(-3.85185988875507E-34,1.,0.));
#113354=DIRECTION('ref_axis',(1.,3.85185988875507E-34,0.));
#113355=DIRECTION('',(-3.85185988875507E-34,1.,0.));
#113356=DIRECTION('',(3.85185988875507E-34,-1.,0.));
#113357=DIRECTION('center_axis',(-3.85185988875507E-34,1.,0.));
#113358=DIRECTION('ref_axis',(0.,0.,1.));
#113359=DIRECTION('center_axis',(-3.85185988875507E-34,1.,0.));
#113360=DIRECTION('ref_axis',(1.,3.85185988875507E-34,0.));
#113361=DIRECTION('',(-3.85185988875507E-34,1.,0.));
#113362=DIRECTION('',(3.85185988875507E-34,-1.,0.));
#113363=DIRECTION('center_axis',(-3.85185988875507E-34,1.,0.));
#113364=DIRECTION('ref_axis',(0.,0.,1.));
#113365=DIRECTION('center_axis',(-3.85185988875507E-34,1.,0.));
#113366=DIRECTION('ref_axis',(1.,3.85185988875507E-34,0.));
#113367=DIRECTION('',(3.85185988875507E-34,-1.,0.));
#113368=DIRECTION('center_axis',(-3.85185988875507E-34,1.,0.));
#113369=DIRECTION('ref_axis',(0.,0.,1.));
#113370=DIRECTION('',(-3.85185988875507E-34,1.,0.));
#113371=DIRECTION('center_axis',(-3.85185988875507E-34,1.,0.));
#113372=DIRECTION('ref_axis',(1.,3.85185988875507E-34,0.));
#113373=DIRECTION('',(-3.85185988875507E-34,1.,0.));
#113374=DIRECTION('',(3.85185988875507E-34,-1.,0.));
#113375=DIRECTION('center_axis',(-3.85185988875507E-34,1.,0.));
#113376=DIRECTION('ref_axis',(0.,0.,1.));
#113377=DIRECTION('center_axis',(-3.85185988875507E-34,1.,0.));
#113378=DIRECTION('ref_axis',(1.,3.85185988875507E-34,0.));
#113379=DIRECTION('',(3.85185988875507E-34,-1.,0.));
#113380=DIRECTION('center_axis',(-3.85185988875507E-34,1.,0.));
#113381=DIRECTION('ref_axis',(0.,0.,1.));
#113382=DIRECTION('',(-3.85185988875507E-34,1.,0.));
#113383=DIRECTION('center_axis',(-3.85185988875507E-34,1.,0.));
#113384=DIRECTION('ref_axis',(1.,3.85185988875507E-34,0.));
#113385=DIRECTION('',(3.85185988875507E-34,-1.,0.));
#113386=DIRECTION('center_axis',(-3.85185988875507E-34,1.,0.));
#113387=DIRECTION('ref_axis',(0.,0.,1.));
#113388=DIRECTION('',(-3.85185988875507E-34,1.,0.));
#113389=DIRECTION('center_axis',(-3.85185988875507E-34,1.,0.));
#113390=DIRECTION('ref_axis',(1.,3.85185988875507E-34,0.));
#113391=DIRECTION('',(3.85185988875507E-34,-1.,0.));
#113392=DIRECTION('center_axis',(-3.85185988875507E-34,1.,0.));
#113393=DIRECTION('ref_axis',(0.,0.,1.));
#113394=DIRECTION('',(-3.85185988875507E-34,1.,0.));
#113395=DIRECTION('center_axis',(-3.85185988875507E-34,1.,0.));
#113396=DIRECTION('ref_axis',(1.,3.85185988875507E-34,0.));
#113397=DIRECTION('',(-3.85185988875507E-34,1.,0.));
#113398=DIRECTION('',(3.85185988875507E-34,-1.,0.));
#113399=DIRECTION('center_axis',(-3.85185988875507E-34,1.,0.));
#113400=DIRECTION('ref_axis',(0.,0.,1.));
#113401=DIRECTION('center_axis',(-3.85185988875507E-34,1.,0.));
#113402=DIRECTION('ref_axis',(1.,3.85185988875507E-34,0.));
#113403=DIRECTION('',(-3.85185988875507E-34,1.,0.));
#113404=DIRECTION('',(3.85185988875507E-34,-1.,0.));
#113405=DIRECTION('center_axis',(-3.85185988875507E-34,1.,0.));
#113406=DIRECTION('ref_axis',(0.,0.,1.));
#113407=DIRECTION('center_axis',(-3.85185988875507E-34,1.,0.));
#113408=DIRECTION('ref_axis',(1.,3.85185988875507E-34,0.));
#113409=DIRECTION('',(-3.85185988875507E-34,1.,0.));
#113410=DIRECTION('',(3.85185988875507E-34,-1.,0.));
#113411=DIRECTION('center_axis',(-3.85185988875507E-34,1.,0.));
#113412=DIRECTION('ref_axis',(0.,0.,1.));
#113413=DIRECTION('center_axis',(3.85185988875507E-34,-1.,0.));
#113414=DIRECTION('ref_axis',(-1.,-3.85185988875507E-34,0.));
#113415=DIRECTION('center_axis',(-3.85185988875507E-34,1.,0.));
#113416=DIRECTION('ref_axis',(0.,0.,1.));
#113417=DIRECTION('center_axis',(3.85185988875507E-34,-1.,0.));
#113418=DIRECTION('ref_axis',(0.,0.,1.));
#113419=DIRECTION('center_axis',(-3.85185988875507E-34,1.,0.));
#113420=DIRECTION('ref_axis',(0.,0.,1.));
#113421=DIRECTION('center_axis',(-3.85185988875507E-34,1.,0.));
#113422=DIRECTION('ref_axis',(0.,0.,1.));
#113423=DIRECTION('center_axis',(3.85185988875507E-34,-1.,0.));
#113424=DIRECTION('ref_axis',(0.,0.,1.));
#113425=DIRECTION('center_axis',(-3.85185988875507E-34,1.,0.));
#113426=DIRECTION('ref_axis',(0.,0.,1.));
#113427=DIRECTION('center_axis',(-3.85185988875507E-34,1.,0.));
#113428=DIRECTION('ref_axis',(0.,0.,1.));
#113429=DIRECTION('center_axis',(3.85185988875507E-34,-1.,0.));
#113430=DIRECTION('ref_axis',(0.,0.,1.));
#113431=DIRECTION('center_axis',(-3.85185988875507E-34,1.,0.));
#113432=DIRECTION('ref_axis',(0.,0.,1.));
#113433=DIRECTION('center_axis',(-3.85185988875507E-34,1.,0.));
#113434=DIRECTION('ref_axis',(0.,0.,1.));
#113435=DIRECTION('center_axis',(3.85185988875507E-34,-1.,0.));
#113436=DIRECTION('ref_axis',(0.,0.,1.));
#113437=DIRECTION('center_axis',(-3.85185988875507E-34,1.,0.));
#113438=DIRECTION('ref_axis',(0.,0.,1.));
#113439=DIRECTION('center_axis',(-3.85185988875507E-34,1.,0.));
#113440=DIRECTION('ref_axis',(0.,0.,1.));
#113441=DIRECTION('center_axis',(3.85185988875507E-34,-1.,0.));
#113442=DIRECTION('ref_axis',(0.,0.,1.));
#113443=DIRECTION('center_axis',(-3.85185988875507E-34,1.,0.));
#113444=DIRECTION('ref_axis',(0.,0.,1.));
#113445=DIRECTION('center_axis',(-3.85185988875507E-34,1.,0.));
#113446=DIRECTION('ref_axis',(0.,0.,1.));
#113447=DIRECTION('center_axis',(3.85185988875507E-34,-1.,0.));
#113448=DIRECTION('ref_axis',(0.,0.,1.));
#113449=DIRECTION('center_axis',(-3.85185988875507E-34,1.,0.));
#113450=DIRECTION('ref_axis',(0.,0.,1.));
#113451=DIRECTION('center_axis',(3.85185988875507E-34,-1.,0.));
#113452=DIRECTION('ref_axis',(0.,0.,1.));
#113453=DIRECTION('center_axis',(-3.85185988875507E-34,1.,0.));
#113454=DIRECTION('ref_axis',(0.,0.,1.));
#113455=DIRECTION('center_axis',(3.85185988875507E-34,-1.,0.));
#113456=DIRECTION('ref_axis',(0.,0.,1.));
#113457=DIRECTION('center_axis',(-3.85185988875507E-34,1.,0.));
#113458=DIRECTION('ref_axis',(0.,0.,1.));
#113459=DIRECTION('center_axis',(-3.85185988875507E-34,1.,0.));
#113460=DIRECTION('ref_axis',(0.,0.,1.));
#113461=DIRECTION('center_axis',(-3.85185988875507E-34,1.,0.));
#113462=DIRECTION('ref_axis',(0.,0.,1.));
#113463=DIRECTION('center_axis',(3.85185988875507E-34,-1.,0.));
#113464=DIRECTION('ref_axis',(0.,0.,1.));
#113465=DIRECTION('center_axis',(-3.85185988875507E-34,1.,0.));
#113466=DIRECTION('ref_axis',(0.,0.,1.));
#113467=DIRECTION('center_axis',(-3.85185988875507E-34,1.,0.));
#113468=DIRECTION('ref_axis',(0.,0.,1.));
#113469=DIRECTION('center_axis',(3.85185988875507E-34,-1.,0.));
#113470=DIRECTION('ref_axis',(0.,0.,1.));
#113471=DIRECTION('center_axis',(-3.85185988875507E-34,1.,0.));
#113472=DIRECTION('ref_axis',(0.,0.,1.));
#113473=DIRECTION('center_axis',(-3.85185988875507E-34,1.,0.));
#113474=DIRECTION('ref_axis',(0.,0.,1.));
#113475=DIRECTION('center_axis',(3.85185988875507E-34,-1.,0.));
#113476=DIRECTION('ref_axis',(0.,0.,1.));
#113477=DIRECTION('center_axis',(-3.85185988875507E-34,1.,0.));
#113478=DIRECTION('ref_axis',(0.,0.,1.));
#113479=DIRECTION('center_axis',(-3.85185988875507E-34,1.,0.));
#113480=DIRECTION('ref_axis',(0.,0.,1.));
#113481=DIRECTION('center_axis',(3.85185988875507E-34,-1.,0.));
#113482=DIRECTION('ref_axis',(0.,0.,1.));
#113483=DIRECTION('center_axis',(-3.85185988875507E-34,1.,0.));
#113484=DIRECTION('ref_axis',(0.,0.,1.));
#113485=DIRECTION('center_axis',(-3.85185988875507E-34,1.,0.));
#113486=DIRECTION('ref_axis',(0.,0.,1.));
#113487=DIRECTION('center_axis',(3.85185988875507E-34,-1.,0.));
#113488=DIRECTION('ref_axis',(0.,0.,1.));
#113489=DIRECTION('center_axis',(-3.85185988875507E-34,1.,0.));
#113490=DIRECTION('ref_axis',(0.,0.,1.));
#113491=DIRECTION('center_axis',(-3.85185988875507E-34,1.,0.));
#113492=DIRECTION('ref_axis',(0.,0.,1.));
#113493=DIRECTION('center_axis',(3.85185988875507E-34,-1.,0.));
#113494=DIRECTION('ref_axis',(0.,0.,1.));
#113495=DIRECTION('center_axis',(-3.85185988875507E-34,1.,0.));
#113496=DIRECTION('ref_axis',(0.,0.,1.));
#113497=DIRECTION('center_axis',(-3.85185988875507E-34,1.,0.));
#113498=DIRECTION('ref_axis',(0.,0.,1.));
#113499=DIRECTION('center_axis',(3.85185988875507E-34,-1.,0.));
#113500=DIRECTION('ref_axis',(0.,0.,1.));
#113501=DIRECTION('center_axis',(-3.85185988875507E-34,1.,0.));
#113502=DIRECTION('ref_axis',(0.,0.,1.));
#113503=DIRECTION('center_axis',(-3.85185988875507E-34,1.,0.));
#113504=DIRECTION('ref_axis',(0.,0.,1.));
#113505=DIRECTION('center_axis',(3.85185988875507E-34,-1.,0.));
#113506=DIRECTION('ref_axis',(0.,0.,1.));
#113507=DIRECTION('center_axis',(-3.85185988875507E-34,1.,0.));
#113508=DIRECTION('ref_axis',(0.,0.,1.));
#113509=DIRECTION('center_axis',(-3.85185988875507E-34,1.,0.));
#113510=DIRECTION('ref_axis',(0.,0.,1.));
#113511=DIRECTION('center_axis',(3.85185988875507E-34,-1.,0.));
#113512=DIRECTION('ref_axis',(0.,0.,1.));
#113513=DIRECTION('center_axis',(-3.85185988875507E-34,1.,0.));
#113514=DIRECTION('ref_axis',(0.,0.,1.));
#113515=DIRECTION('center_axis',(-3.85185988875507E-34,1.,0.));
#113516=DIRECTION('ref_axis',(0.,0.,1.));
#113517=DIRECTION('center_axis',(3.85185988875507E-34,-1.,0.));
#113518=DIRECTION('ref_axis',(0.,0.,1.));
#113519=DIRECTION('center_axis',(-3.85185988875507E-34,1.,0.));
#113520=DIRECTION('ref_axis',(0.,0.,1.));
#113521=DIRECTION('center_axis',(-3.85185988875507E-34,1.,0.));
#113522=DIRECTION('ref_axis',(0.,0.,1.));
#113523=DIRECTION('center_axis',(3.85185988875507E-34,-1.,0.));
#113524=DIRECTION('ref_axis',(0.,0.,1.));
#113525=DIRECTION('center_axis',(-3.85185988875507E-34,1.,0.));
#113526=DIRECTION('ref_axis',(0.,0.,1.));
#113527=DIRECTION('center_axis',(-3.85185988875507E-34,1.,0.));
#113528=DIRECTION('ref_axis',(0.,0.,1.));
#113529=DIRECTION('center_axis',(3.85185988875507E-34,-1.,0.));
#113530=DIRECTION('ref_axis',(0.,0.,1.));
#113531=DIRECTION('center_axis',(-3.85185988875507E-34,1.,0.));
#113532=DIRECTION('ref_axis',(0.,0.,1.));
#113533=DIRECTION('center_axis',(-3.85185988875507E-34,1.,0.));
#113534=DIRECTION('ref_axis',(0.,0.,1.));
#113535=DIRECTION('center_axis',(3.85185988875507E-34,-1.,0.));
#113536=DIRECTION('ref_axis',(0.,0.,1.));
#113537=DIRECTION('center_axis',(-3.85185988875507E-34,1.,0.));
#113538=DIRECTION('ref_axis',(0.,0.,1.));
#113539=DIRECTION('center_axis',(-3.85185988875507E-34,1.,0.));
#113540=DIRECTION('ref_axis',(0.,0.,1.));
#113541=DIRECTION('center_axis',(3.85185988875507E-34,-1.,0.));
#113542=DIRECTION('ref_axis',(0.,0.,1.));
#113543=DIRECTION('center_axis',(-3.85185988875507E-34,1.,0.));
#113544=DIRECTION('ref_axis',(0.,0.,1.));
#113545=DIRECTION('center_axis',(-3.85185988875507E-34,1.,0.));
#113546=DIRECTION('ref_axis',(0.,0.,1.));
#113547=DIRECTION('center_axis',(3.85185988875507E-34,-1.,0.));
#113548=DIRECTION('ref_axis',(0.,0.,1.));
#113549=DIRECTION('center_axis',(-3.85185988875507E-34,1.,0.));
#113550=DIRECTION('ref_axis',(0.,0.,1.));
#113551=DIRECTION('center_axis',(-3.85185988875507E-34,1.,0.));
#113552=DIRECTION('ref_axis',(0.,0.,1.));
#113553=DIRECTION('center_axis',(3.85185988875507E-34,-1.,0.));
#113554=DIRECTION('ref_axis',(0.,0.,1.));
#113555=DIRECTION('center_axis',(-3.85185988875507E-34,1.,0.));
#113556=DIRECTION('ref_axis',(0.,0.,1.));
#113557=DIRECTION('center_axis',(-3.85185988875507E-34,1.,0.));
#113558=DIRECTION('ref_axis',(0.,0.,1.));
#113559=DIRECTION('center_axis',(3.85185988875507E-34,-1.,0.));
#113560=DIRECTION('ref_axis',(0.,0.,1.));
#113561=DIRECTION('center_axis',(-3.85185988875507E-34,1.,0.));
#113562=DIRECTION('ref_axis',(0.,0.,1.));
#113563=DIRECTION('center_axis',(-3.85185988875507E-34,1.,0.));
#113564=DIRECTION('ref_axis',(0.,0.,1.));
#113565=DIRECTION('center_axis',(3.85185988875507E-34,-1.,0.));
#113566=DIRECTION('ref_axis',(0.,0.,1.));
#113567=DIRECTION('center_axis',(-3.85185988875507E-34,1.,0.));
#113568=DIRECTION('ref_axis',(0.,0.,1.));
#113569=DIRECTION('center_axis',(-3.85185988875507E-34,1.,0.));
#113570=DIRECTION('ref_axis',(0.,0.,1.));
#113571=DIRECTION('center_axis',(3.85185988875507E-34,-1.,0.));
#113572=DIRECTION('ref_axis',(0.,0.,1.));
#113573=DIRECTION('center_axis',(-3.85185988875507E-34,1.,0.));
#113574=DIRECTION('ref_axis',(0.,0.,1.));
#113575=DIRECTION('center_axis',(-3.85185988875507E-34,1.,0.));
#113576=DIRECTION('ref_axis',(0.,0.,1.));
#113577=DIRECTION('center_axis',(3.85185988875507E-34,-1.,0.));
#113578=DIRECTION('ref_axis',(0.,0.,1.));
#113579=DIRECTION('center_axis',(-3.85185988875507E-34,1.,0.));
#113580=DIRECTION('ref_axis',(0.,0.,1.));
#113581=DIRECTION('center_axis',(-3.85185988875507E-34,1.,0.));
#113582=DIRECTION('ref_axis',(0.,0.,1.));
#113583=DIRECTION('center_axis',(-3.85185988875507E-34,1.,0.));
#113584=DIRECTION('ref_axis',(0.,0.,1.));
#113585=DIRECTION('center_axis',(-3.85185988875507E-34,1.,0.));
#113586=DIRECTION('ref_axis',(0.,0.,1.));
#113587=DIRECTION('center_axis',(-3.85185988875507E-34,1.,0.));
#113588=DIRECTION('ref_axis',(0.,0.,1.));
#113589=DIRECTION('center_axis',(-3.85185988875507E-34,1.,0.));
#113590=DIRECTION('ref_axis',(0.,0.,1.));
#113591=DIRECTION('center_axis',(3.85185988875507E-34,-1.,0.));
#113592=DIRECTION('ref_axis',(0.,0.,1.));
#113593=DIRECTION('center_axis',(-3.85185988875507E-34,1.,0.));
#113594=DIRECTION('ref_axis',(0.,0.,1.));
#113595=DIRECTION('center_axis',(-3.85185988875507E-34,1.,0.));
#113596=DIRECTION('ref_axis',(0.,0.,1.));
#113597=DIRECTION('center_axis',(3.85185988875507E-34,-1.,0.));
#113598=DIRECTION('ref_axis',(0.,0.,1.));
#113599=DIRECTION('center_axis',(-3.85185988875507E-34,1.,0.));
#113600=DIRECTION('ref_axis',(0.,0.,1.));
#113601=DIRECTION('center_axis',(-3.85185988875507E-34,1.,0.));
#113602=DIRECTION('ref_axis',(0.,0.,1.));
#113603=DIRECTION('center_axis',(3.85185988875507E-34,-1.,0.));
#113604=DIRECTION('ref_axis',(0.,0.,1.));
#113605=DIRECTION('center_axis',(-3.85185988875507E-34,1.,0.));
#113606=DIRECTION('ref_axis',(0.,0.,1.));
#113607=DIRECTION('center_axis',(-3.85185988875507E-34,1.,0.));
#113608=DIRECTION('ref_axis',(0.,0.,1.));
#113609=DIRECTION('center_axis',(3.85185988875507E-34,-1.,0.));
#113610=DIRECTION('ref_axis',(0.,0.,1.));
#113611=DIRECTION('center_axis',(-3.85185988875507E-34,1.,0.));
#113612=DIRECTION('ref_axis',(0.,0.,1.));
#113613=DIRECTION('center_axis',(-3.85185988875507E-34,1.,0.));
#113614=DIRECTION('ref_axis',(0.,0.,1.));
#113615=DIRECTION('center_axis',(3.85185988875507E-34,-1.,0.));
#113616=DIRECTION('ref_axis',(0.,0.,1.));
#113617=DIRECTION('center_axis',(-3.85185988875507E-34,1.,0.));
#113618=DIRECTION('ref_axis',(0.,0.,1.));
#113619=DIRECTION('center_axis',(-3.85185988875507E-34,1.,0.));
#113620=DIRECTION('ref_axis',(0.,0.,1.));
#113621=DIRECTION('center_axis',(3.85185988875507E-34,-1.,0.));
#113622=DIRECTION('ref_axis',(0.,0.,1.));
#113623=DIRECTION('center_axis',(-3.85185988875507E-34,1.,0.));
#113624=DIRECTION('ref_axis',(0.,0.,1.));
#113625=DIRECTION('center_axis',(-3.85185988875507E-34,1.,0.));
#113626=DIRECTION('ref_axis',(0.,0.,1.));
#113627=DIRECTION('center_axis',(3.85185988875507E-34,-1.,0.));
#113628=DIRECTION('ref_axis',(0.,0.,1.));
#113629=DIRECTION('center_axis',(-3.85185988875507E-34,1.,0.));
#113630=DIRECTION('ref_axis',(0.,0.,1.));
#113631=DIRECTION('center_axis',(-3.85185988875507E-34,1.,0.));
#113632=DIRECTION('ref_axis',(1.,3.85185988875507E-34,0.));
#113633=DIRECTION('',(-3.85185988875507E-34,1.,0.));
#113634=DIRECTION('',(3.85185988875507E-34,-1.,0.));
#113635=DIRECTION('center_axis',(-3.85185988875507E-34,1.,0.));
#113636=DIRECTION('ref_axis',(1.,3.85185988875507E-34,0.));
#113637=DIRECTION('',(-3.85185988875507E-34,1.,0.));
#113638=DIRECTION('center_axis',(-3.85185988875507E-34,1.,0.));
#113639=DIRECTION('ref_axis',(1.,3.85185988875507E-34,0.));
#113640=DIRECTION('',(-3.85185988875507E-34,1.,0.));
#113641=DIRECTION('center_axis',(-3.85185988875507E-34,1.,0.));
#113642=DIRECTION('ref_axis',(1.,3.85185988875507E-34,0.));
#113643=DIRECTION('center_axis',(-3.85185988875507E-34,1.,0.));
#113644=DIRECTION('ref_axis',(1.,3.85185988875507E-34,0.));
#113645=DIRECTION('',(-3.85185988875507E-34,1.,0.));
#113646=DIRECTION('center_axis',(-3.85185988875507E-34,1.,0.));
#113647=DIRECTION('ref_axis',(1.,3.85185988875507E-34,0.));
#113648=DIRECTION('',(-3.85185988875507E-34,1.,0.));
#113649=DIRECTION('center_axis',(-3.85185988875507E-34,1.,0.));
#113650=DIRECTION('ref_axis',(1.,3.85185988875507E-34,0.));
#113651=DIRECTION('center_axis',(-3.85185988875507E-34,1.,0.));
#113652=DIRECTION('ref_axis',(1.,3.85185988875507E-34,0.));
#113653=DIRECTION('',(-3.85185988875507E-34,1.,0.));
#113654=DIRECTION('center_axis',(-3.85185988875507E-34,1.,0.));
#113655=DIRECTION('ref_axis',(1.,3.85185988875507E-34,0.));
#113656=DIRECTION('',(-3.85185988875507E-34,1.,0.));
#113657=DIRECTION('center_axis',(-3.85185988875507E-34,1.,0.));
#113658=DIRECTION('ref_axis',(1.,3.85185988875507E-34,0.));
#113659=DIRECTION('center_axis',(-3.85185988875507E-34,1.,0.));
#113660=DIRECTION('ref_axis',(1.,3.85185988875507E-34,0.));
#113661=DIRECTION('',(-3.85185988875507E-34,1.,0.));
#113662=DIRECTION('center_axis',(-3.85185988875507E-34,1.,0.));
#113663=DIRECTION('ref_axis',(1.,3.85185988875507E-34,0.));
#113664=DIRECTION('',(-3.85185988875507E-34,1.,0.));
#113665=DIRECTION('center_axis',(-3.85185988875507E-34,1.,0.));
#113666=DIRECTION('ref_axis',(1.,3.85185988875507E-34,0.));
#113667=DIRECTION('center_axis',(-3.85185988875507E-34,1.,0.));
#113668=DIRECTION('ref_axis',(1.,3.85185988875507E-34,0.));
#113669=DIRECTION('',(-3.85185988875507E-34,1.,0.));
#113670=DIRECTION('center_axis',(-3.85185988875507E-34,1.,0.));
#113671=DIRECTION('ref_axis',(1.,3.85185988875507E-34,0.));
#113672=DIRECTION('',(-3.85185988875507E-34,1.,0.));
#113673=DIRECTION('center_axis',(-3.85185988875507E-34,1.,0.));
#113674=DIRECTION('ref_axis',(1.,3.85185988875507E-34,0.));
#113675=DIRECTION('center_axis',(-3.85185988875507E-34,1.,0.));
#113676=DIRECTION('ref_axis',(1.,3.85185988875507E-34,0.));
#113677=DIRECTION('',(-3.85185988875507E-34,1.,0.));
#113678=DIRECTION('center_axis',(-3.85185988875507E-34,1.,0.));
#113679=DIRECTION('ref_axis',(1.,3.85185988875507E-34,0.));
#113680=DIRECTION('',(-3.85185988875507E-34,1.,0.));
#113681=DIRECTION('center_axis',(-3.85185988875507E-34,1.,0.));
#113682=DIRECTION('ref_axis',(1.,3.85185988875507E-34,0.));
#113683=DIRECTION('center_axis',(-3.85185988875507E-34,1.,0.));
#113684=DIRECTION('ref_axis',(1.,3.85185988875507E-34,0.));
#113685=DIRECTION('',(-3.85185988875507E-34,1.,0.));
#113686=DIRECTION('center_axis',(-3.85185988875507E-34,1.,0.));
#113687=DIRECTION('ref_axis',(1.,3.85185988875507E-34,0.));
#113688=DIRECTION('',(-3.85185988875507E-34,1.,0.));
#113689=DIRECTION('center_axis',(-3.85185988875507E-34,1.,0.));
#113690=DIRECTION('ref_axis',(1.,3.85185988875507E-34,0.));
#113691=DIRECTION('center_axis',(-3.85185988875507E-34,1.,0.));
#113692=DIRECTION('ref_axis',(1.,3.85185988875507E-34,0.));
#113693=DIRECTION('',(-3.85185988875507E-34,1.,0.));
#113694=DIRECTION('center_axis',(-3.85185988875507E-34,1.,0.));
#113695=DIRECTION('ref_axis',(-0.998948206426938,-3.84780852727974E-34,
-0.0458528175405152));
#113696=DIRECTION('',(-3.85185988875507E-34,1.,0.));
#113697=DIRECTION('center_axis',(-3.85185988875507E-34,1.,0.));
#113698=DIRECTION('ref_axis',(1.,3.85185988875507E-34,0.));
#113699=DIRECTION('center_axis',(-3.85185988875507E-34,1.,0.));
#113700=DIRECTION('ref_axis',(1.,3.85185988875507E-34,0.));
#113701=DIRECTION('',(-3.85185988875507E-34,1.,0.));
#113702=DIRECTION('center_axis',(-3.85185988875507E-34,1.,0.));
#113703=DIRECTION('ref_axis',(-0.992328409627066,-3.8223099975146E-34,0.123629799995869));
#113704=DIRECTION('',(-3.85185988875507E-34,1.,0.));
#113705=DIRECTION('center_axis',(-3.85185988875507E-34,1.,0.));
#113706=DIRECTION('ref_axis',(1.,3.85185988875507E-34,0.));
#113707=DIRECTION('center_axis',(-3.85185988875507E-34,1.,0.));
#113708=DIRECTION('ref_axis',(1.,3.85185988875507E-34,0.));
#113709=DIRECTION('',(-3.85185988875507E-34,1.,0.));
#113710=DIRECTION('center_axis',(-3.85185988875507E-34,1.,0.));
#113711=DIRECTION('ref_axis',(1.,3.85185988875507E-34,0.));
#113712=DIRECTION('',(-3.85185988875507E-34,1.,0.));
#113713=DIRECTION('center_axis',(-3.85185988875507E-34,1.,0.));
#113714=DIRECTION('ref_axis',(1.,3.85185988875507E-34,0.));
#113715=DIRECTION('center_axis',(-3.85185988875507E-34,1.,0.));
#113716=DIRECTION('ref_axis',(1.,3.85185988875507E-34,0.));
#113717=DIRECTION('',(-3.85185988875507E-34,1.,0.));
#113718=DIRECTION('center_axis',(-3.85185988875507E-34,1.,0.));
#113719=DIRECTION('ref_axis',(1.,3.85185988875507E-34,0.));
#113720=DIRECTION('',(-3.85185988875507E-34,1.,0.));
#113721=DIRECTION('center_axis',(-3.85185988875507E-34,1.,0.));
#113722=DIRECTION('ref_axis',(1.,3.85185988875507E-34,0.));
#113723=DIRECTION('center_axis',(-3.85185988875507E-34,1.,0.));
#113724=DIRECTION('ref_axis',(1.,3.85185988875507E-34,0.));
#113725=DIRECTION('',(-3.85185988875507E-34,1.,0.));
#113726=DIRECTION('center_axis',(-3.85185988875507E-34,1.,0.));
#113727=DIRECTION('ref_axis',(1.,3.85185988875507E-34,0.));
#113728=DIRECTION('',(-3.85185988875507E-34,1.,0.));
#113729=DIRECTION('center_axis',(-3.85185988875507E-34,1.,0.));
#113730=DIRECTION('ref_axis',(1.,3.85185988875507E-34,0.));
#113731=DIRECTION('center_axis',(-3.85185988875507E-34,1.,0.));
#113732=DIRECTION('ref_axis',(-0.991460893518391,-3.81896844701275E-34,
0.130404358146931));
#113733=DIRECTION('',(-3.85185988875507E-34,1.,0.));
#113734=DIRECTION('center_axis',(-3.85185988875507E-34,1.,0.));
#113735=DIRECTION('ref_axis',(1.,3.85185988875507E-34,0.));
#113736=DIRECTION('',(-3.85185988875507E-34,1.,0.));
#113737=DIRECTION('center_axis',(-3.85185988875507E-34,1.,0.));
#113738=DIRECTION('ref_axis',(1.,3.85185988875507E-34,0.));
#113739=DIRECTION('center_axis',(-3.85185988875507E-34,1.,0.));
#113740=DIRECTION('ref_axis',(1.,3.85185988875507E-34,0.));
#113741=DIRECTION('',(-3.85185988875507E-34,1.,0.));
#113742=DIRECTION('center_axis',(-3.85185988875507E-34,1.,0.));
#113743=DIRECTION('ref_axis',(1.,3.85185988875507E-34,0.));
#113744=DIRECTION('',(-3.85185988875507E-34,1.,0.));
#113745=DIRECTION('center_axis',(-3.85185988875507E-34,1.,0.));
#113746=DIRECTION('ref_axis',(1.,3.85185988875507E-34,0.));
#113747=DIRECTION('center_axis',(-3.85185988875507E-34,1.,0.));
#113748=DIRECTION('ref_axis',(-0.999238074648388,-3.84892505905497E-34,
-0.0390290939298224));
#113749=DIRECTION('',(-3.85185988875507E-34,1.,0.));
#113750=DIRECTION('center_axis',(-3.85185988875507E-34,1.,0.));
#113751=DIRECTION('ref_axis',(1.,3.85185988875507E-34,0.));
#113752=DIRECTION('',(-3.85185988875507E-34,1.,0.));
#113753=DIRECTION('center_axis',(-3.85185988875507E-34,1.,0.));
#113754=DIRECTION('ref_axis',(1.,3.85185988875507E-34,0.));
#113755=DIRECTION('center_axis',(-3.85185988875507E-34,1.,0.));
#113756=DIRECTION('ref_axis',(1.,3.85185988875507E-34,0.));
#113757=DIRECTION('',(-3.85185988875507E-34,1.,0.));
#113758=DIRECTION('center_axis',(-3.85185988875507E-34,1.,0.));
#113759=DIRECTION('ref_axis',(1.,3.85185988875507E-34,0.));
#113760=DIRECTION('',(-3.85185988875507E-34,1.,0.));
#113761=DIRECTION('center_axis',(-3.85185988875507E-34,1.,0.));
#113762=DIRECTION('ref_axis',(1.,3.85185988875507E-34,0.));
#113763=DIRECTION('center_axis',(-3.85185988875507E-34,1.,0.));
#113764=DIRECTION('ref_axis',(1.,3.85185988875507E-34,0.));
#113765=DIRECTION('',(-3.85185988875507E-34,1.,0.));
#113766=DIRECTION('center_axis',(-3.85185988875507E-34,1.,0.));
#113767=DIRECTION('ref_axis',(1.,3.85185988875507E-34,0.));
#113768=DIRECTION('',(-3.85185988875507E-34,1.,0.));
#113769=DIRECTION('center_axis',(-3.85185988875507E-34,1.,0.));
#113770=DIRECTION('ref_axis',(1.,3.85185988875507E-34,0.));
#113771=DIRECTION('center_axis',(-3.85185988875507E-34,1.,0.));
#113772=DIRECTION('ref_axis',(1.,3.85185988875507E-34,0.));
#113773=DIRECTION('',(-3.85185988875507E-34,1.,0.));
#113774=DIRECTION('center_axis',(-3.85185988875507E-34,1.,0.));
#113775=DIRECTION('ref_axis',(1.,3.85185988875507E-34,0.));
#113776=DIRECTION('',(-3.85185988875507E-34,1.,0.));
#113777=DIRECTION('center_axis',(-3.85185988875507E-34,1.,0.));
#113778=DIRECTION('ref_axis',(1.,3.85185988875507E-34,0.));
#113779=DIRECTION('center_axis',(-3.85185988875507E-34,1.,0.));
#113780=DIRECTION('ref_axis',(1.,3.85185988875507E-34,0.));
#113781=DIRECTION('',(-3.85185988875507E-34,1.,0.));
#113782=DIRECTION('center_axis',(-3.85185988875507E-34,1.,0.));
#113783=DIRECTION('ref_axis',(1.,3.85185988875507E-34,0.));
#113784=DIRECTION('',(-3.85185988875507E-34,1.,0.));
#113785=DIRECTION('center_axis',(-3.85185988875507E-34,1.,0.));
#113786=DIRECTION('ref_axis',(1.,3.85185988875507E-34,0.));
#113787=DIRECTION('center_axis',(-3.85185988875507E-34,1.,0.));
#113788=DIRECTION('ref_axis',(1.,3.85185988875507E-34,0.));
#113789=DIRECTION('',(-3.85185988875507E-34,1.,0.));
#113790=DIRECTION('center_axis',(-3.85185988875507E-34,1.,0.));
#113791=DIRECTION('ref_axis',(1.,3.85185988875507E-34,0.));
#113792=DIRECTION('',(-3.85185988875507E-34,1.,0.));
#113793=DIRECTION('center_axis',(-3.85185988875507E-34,1.,0.));
#113794=DIRECTION('ref_axis',(1.,3.85185988875507E-34,0.));
#113795=DIRECTION('center_axis',(-3.85185988875507E-34,1.,0.));
#113796=DIRECTION('ref_axis',(1.,3.85185988875507E-34,0.));
#113797=DIRECTION('',(-3.85185988875507E-34,1.,0.));
#113798=DIRECTION('center_axis',(-3.85185988875507E-34,1.,0.));
#113799=DIRECTION('ref_axis',(1.,3.85185988875507E-34,0.));
#113800=DIRECTION('',(-3.85185988875507E-34,1.,0.));
#113801=DIRECTION('center_axis',(-3.85185988875507E-34,1.,0.));
#113802=DIRECTION('ref_axis',(1.,3.85185988875507E-34,0.));
#113803=DIRECTION('center_axis',(-3.85185988875507E-34,1.,0.));
#113804=DIRECTION('ref_axis',(1.,3.85185988875507E-34,0.));
#113805=DIRECTION('',(-3.85185988875507E-34,1.,0.));
#113806=DIRECTION('center_axis',(-3.85185988875507E-34,1.,0.));
#113807=DIRECTION('ref_axis',(1.,3.85185988875507E-34,0.));
#113808=DIRECTION('',(-3.85185988875507E-34,1.,0.));
#113809=DIRECTION('center_axis',(-3.85185988875507E-34,1.,0.));
#113810=DIRECTION('ref_axis',(1.,3.85185988875507E-34,0.));
#113811=DIRECTION('center_axis',(-3.85185988875507E-34,1.,0.));
#113812=DIRECTION('ref_axis',(1.,3.85185988875507E-34,0.));
#113813=DIRECTION('',(-3.85185988875507E-34,1.,0.));
#113814=DIRECTION('center_axis',(-3.85185988875507E-34,1.,0.));
#113815=DIRECTION('ref_axis',(1.,3.85185988875507E-34,0.));
#113816=DIRECTION('',(-3.85185988875507E-34,1.,0.));
#113817=DIRECTION('center_axis',(-3.85185988875507E-34,1.,0.));
#113818=DIRECTION('ref_axis',(1.,3.85185988875507E-34,0.));
#113819=DIRECTION('center_axis',(-3.85185988875507E-34,1.,0.));
#113820=DIRECTION('ref_axis',(1.,3.85185988875507E-34,0.));
#113821=DIRECTION('',(-3.85185988875507E-34,1.,0.));
#113822=DIRECTION('center_axis',(-3.85185988875507E-34,1.,0.));
#113823=DIRECTION('ref_axis',(1.,3.85185988875507E-34,0.));
#113824=DIRECTION('',(-3.85185988875507E-34,1.,0.));
#113825=DIRECTION('center_axis',(-3.85185988875507E-34,1.,0.));
#113826=DIRECTION('ref_axis',(1.,3.85185988875507E-34,0.));
#113827=DIRECTION('center_axis',(-3.85185988875507E-34,1.,0.));
#113828=DIRECTION('ref_axis',(1.,3.85185988875507E-34,0.));
#113829=DIRECTION('',(-3.85185988875507E-34,1.,0.));
#113830=DIRECTION('center_axis',(-3.85185988875507E-34,1.,0.));
#113831=DIRECTION('ref_axis',(1.,3.85185988875507E-34,0.));
#113832=DIRECTION('',(-3.85185988875507E-34,1.,0.));
#113833=DIRECTION('center_axis',(-3.85185988875507E-34,1.,0.));
#113834=DIRECTION('ref_axis',(1.,3.85185988875507E-34,0.));
#113835=DIRECTION('center_axis',(-3.85185988875507E-34,1.,0.));
#113836=DIRECTION('ref_axis',(1.,3.85185988875507E-34,0.));
#113837=DIRECTION('',(-3.85185988875507E-34,1.,0.));
#113838=DIRECTION('center_axis',(-3.85185988875507E-34,1.,0.));
#113839=DIRECTION('ref_axis',(1.,3.85185988875507E-34,0.));
#113840=DIRECTION('center_axis',(-3.85185988875507E-34,1.,0.));
#113841=DIRECTION('ref_axis',(1.,3.85185988875507E-34,0.));
#113842=DIRECTION('',(-3.85185988875507E-34,1.,0.));
#113843=DIRECTION('center_axis',(-3.85185988875507E-34,1.,0.));
#113844=DIRECTION('ref_axis',(1.,3.85185988875507E-34,0.));
#113845=DIRECTION('center_axis',(-3.85185988875507E-34,1.,0.));
#113846=DIRECTION('ref_axis',(1.,3.85185988875507E-34,0.));
#113847=DIRECTION('',(-3.85185988875507E-34,1.,0.));
#113848=DIRECTION('center_axis',(-3.85185988875507E-34,1.,0.));
#113849=DIRECTION('ref_axis',(1.,3.85185988875507E-34,0.));
#113850=DIRECTION('',(-3.85185988875507E-34,1.,0.));
#113851=DIRECTION('center_axis',(-3.85185988875507E-34,1.,0.));
#113852=DIRECTION('ref_axis',(1.,3.85185988875507E-34,0.));
#113853=DIRECTION('center_axis',(-3.85185988875507E-34,1.,0.));
#113854=DIRECTION('ref_axis',(1.,3.85185988875507E-34,0.));
#113855=DIRECTION('',(-3.85185988875507E-34,1.,0.));
#113856=DIRECTION('center_axis',(-3.85185988875507E-34,1.,0.));
#113857=DIRECTION('ref_axis',(1.,3.85185988875507E-34,0.));
#113858=DIRECTION('',(-3.85185988875507E-34,1.,0.));
#113859=DIRECTION('center_axis',(-3.85185988875507E-34,1.,0.));
#113860=DIRECTION('ref_axis',(1.,3.85185988875507E-34,0.));
#113861=DIRECTION('center_axis',(-3.85185988875507E-34,1.,0.));
#113862=DIRECTION('ref_axis',(1.,3.85185988875507E-34,0.));
#113863=DIRECTION('',(-3.85185988875507E-34,1.,0.));
#113864=DIRECTION('center_axis',(-3.85185988875507E-34,1.,0.));
#113865=DIRECTION('ref_axis',(1.,3.85185988875507E-34,0.));
#113866=DIRECTION('',(-3.85185988875507E-34,1.,0.));
#113867=DIRECTION('center_axis',(-3.85185988875507E-34,1.,0.));
#113868=DIRECTION('ref_axis',(1.,3.85185988875507E-34,0.));
#113869=DIRECTION('center_axis',(-3.85185988875507E-34,1.,0.));
#113870=DIRECTION('ref_axis',(1.,3.85185988875507E-34,0.));
#113871=DIRECTION('',(-3.85185988875507E-34,1.,0.));
#113872=DIRECTION('center_axis',(-3.85185988875507E-34,1.,0.));
#113873=DIRECTION('ref_axis',(1.,3.85185988875507E-34,0.));
#113874=DIRECTION('',(-3.85185988875507E-34,1.,0.));
#113875=DIRECTION('center_axis',(-3.85185988875507E-34,1.,0.));
#113876=DIRECTION('ref_axis',(1.,3.85185988875507E-34,0.));
#113877=DIRECTION('center_axis',(-3.85185988875507E-34,1.,0.));
#113878=DIRECTION('ref_axis',(1.,3.85185988875507E-34,0.));
#113879=DIRECTION('',(-3.85185988875507E-34,1.,0.));
#113880=DIRECTION('center_axis',(-3.85185988875507E-34,1.,0.));
#113881=DIRECTION('ref_axis',(1.,3.85185988875507E-34,0.));
#113882=DIRECTION('center_axis',(-3.85185988875507E-34,1.,0.));
#113883=DIRECTION('ref_axis',(1.,3.85185988875507E-34,0.));
#113884=DIRECTION('',(-3.85185988875507E-34,1.,0.));
#113885=DIRECTION('center_axis',(-3.85185988875507E-34,1.,0.));
#113886=DIRECTION('ref_axis',(1.,3.85185988875507E-34,0.));
#113887=DIRECTION('center_axis',(-3.85185988875507E-34,1.,0.));
#113888=DIRECTION('ref_axis',(1.,3.85185988875507E-34,0.));
#113889=DIRECTION('',(-3.85185988875507E-34,1.,0.));
#113890=DIRECTION('center_axis',(-3.85185988875507E-34,1.,0.));
#113891=DIRECTION('ref_axis',(1.,3.85185988875507E-34,0.));
#113892=DIRECTION('',(-3.85185988875507E-34,1.,0.));
#113893=DIRECTION('center_axis',(-3.85185988875507E-34,1.,0.));
#113894=DIRECTION('ref_axis',(1.,3.85185988875507E-34,0.));
#113895=DIRECTION('center_axis',(-3.85185988875507E-34,1.,0.));
#113896=DIRECTION('ref_axis',(1.,3.85185988875507E-34,0.));
#113897=DIRECTION('',(-3.85185988875507E-34,1.,0.));
#113898=DIRECTION('center_axis',(-3.85185988875507E-34,1.,0.));
#113899=DIRECTION('ref_axis',(1.,3.85185988875507E-34,0.));
#113900=DIRECTION('',(-3.85185988875507E-34,1.,0.));
#113901=DIRECTION('center_axis',(-3.85185988875507E-34,1.,0.));
#113902=DIRECTION('ref_axis',(1.,3.85185988875507E-34,0.));
#113903=DIRECTION('center_axis',(-3.85185988875507E-34,1.,0.));
#113904=DIRECTION('ref_axis',(1.,3.85185988875507E-34,0.));
#113905=DIRECTION('',(-3.85185988875507E-34,1.,0.));
#113906=DIRECTION('center_axis',(-3.85185988875507E-34,1.,0.));
#113907=DIRECTION('ref_axis',(1.,3.85185988875507E-34,0.));
#113908=DIRECTION('',(-3.85185988875507E-34,1.,0.));
#113909=DIRECTION('center_axis',(-3.85185988875507E-34,1.,0.));
#113910=DIRECTION('ref_axis',(1.,3.85185988875507E-34,0.));
#113911=DIRECTION('center_axis',(-3.85185988875507E-34,1.,0.));
#113912=DIRECTION('ref_axis',(1.,3.85185988875507E-34,0.));
#113913=DIRECTION('',(-3.85185988875507E-34,1.,0.));
#113914=DIRECTION('center_axis',(-3.85185988875507E-34,1.,0.));
#113915=DIRECTION('ref_axis',(1.,3.85185988875507E-34,0.));
#113916=DIRECTION('',(-3.85185988875507E-34,1.,0.));
#113917=DIRECTION('center_axis',(-3.85185988875507E-34,1.,0.));
#113918=DIRECTION('ref_axis',(1.,3.85185988875507E-34,0.));
#113919=DIRECTION('center_axis',(-3.85185988875507E-34,1.,0.));
#113920=DIRECTION('ref_axis',(1.,3.85185988875507E-34,0.));
#113921=DIRECTION('center_axis',(3.85185988875507E-34,-1.,0.));
#113922=DIRECTION('ref_axis',(-1.,-3.85185988875507E-34,0.));
#113923=DIRECTION('center_axis',(3.85185988875507E-34,-1.,0.));
#113924=DIRECTION('ref_axis',(-1.,-3.85185988875507E-34,0.));
#113925=DIRECTION('center_axis',(3.85185988875507E-34,-1.,0.));
#113926=DIRECTION('ref_axis',(-1.,-3.85185988875507E-34,0.));
#113927=DIRECTION('center_axis',(0.333333332905692,1.28395329460448E-34,
-0.942809041733257));
#113928=DIRECTION('ref_axis',(-0.942809041733257,-3.63156833060794E-34,
-0.333333332905692));
#113929=DIRECTION('',(3.85185988875507E-34,-1.,0.));
#113930=DIRECTION('',(-0.942809041733257,-3.63156833060794E-34,-0.333333332905692));
#113931=DIRECTION('',(0.942809041733257,3.63156833060794E-34,0.333333332905692));
#113932=DIRECTION('center_axis',(3.85185988875507E-34,-1.,0.));
#113933=DIRECTION('ref_axis',(-1.,-3.85185988875507E-34,0.));
#113934=DIRECTION('',(3.85185988875507E-34,-1.,0.));
#113935=DIRECTION('center_axis',(3.85185988875507E-34,-1.,0.));
#113936=DIRECTION('ref_axis',(0.,0.,-1.));
#113937=DIRECTION('center_axis',(-3.85185988875507E-34,1.,0.));
#113938=DIRECTION('ref_axis',(0.,0.,-1.));
#113939=DIRECTION('center_axis',(3.85185988875507E-34,-1.,0.));
#113940=DIRECTION('ref_axis',(-1.,-3.85185988875507E-34,0.));
#113941=DIRECTION('',(3.85185988875507E-34,-1.,0.));
#113942=DIRECTION('center_axis',(-3.85185988875507E-34,1.,0.));
#113943=DIRECTION('ref_axis',(0.,0.,-1.));
#113944=DIRECTION('center_axis',(3.85185988875507E-34,-1.,0.));
#113945=DIRECTION('ref_axis',(0.,0.,-1.));
#113946=DIRECTION('center_axis',(3.85185988875507E-34,-1.,0.));
#113947=DIRECTION('ref_axis',(-1.,-3.85185988875507E-34,0.));
#113948=DIRECTION('',(3.85185988875507E-34,-1.,0.));
#113949=DIRECTION('center_axis',(3.85185988875507E-34,-1.,0.));
#113950=DIRECTION('ref_axis',(0.,0.,-1.));
#113951=DIRECTION('center_axis',(-3.85185988875507E-34,1.,0.));
#113952=DIRECTION('ref_axis',(0.,0.,-1.));
#113953=DIRECTION('center_axis',(-0.333333332905692,-1.28395329460448E-34,
-0.942809041733257));
#113954=DIRECTION('ref_axis',(-0.942809041733257,-3.63156833060794E-34,
0.333333332905692));
#113955=DIRECTION('',(3.85185988875507E-34,-1.,0.));
#113956=DIRECTION('',(-0.942809041733257,-3.63156833060794E-34,0.333333332905692));
#113957=DIRECTION('',(0.942809041733257,3.63156833060794E-34,-0.333333332905692));
#113958=DIRECTION('center_axis',(3.85185988875507E-34,-1.,0.));
#113959=DIRECTION('ref_axis',(0.91465912113048,3.52313878056646E-34,0.404226040889028));
#113960=DIRECTION('',(3.85185988875507E-34,-1.,0.));
#113961=DIRECTION('center_axis',(-3.85185988875507E-34,1.,0.));
#113962=DIRECTION('ref_axis',(0.,0.,-1.));
#113963=DIRECTION('center_axis',(3.85185988875507E-34,-1.,0.));
#113964=DIRECTION('ref_axis',(-1.,-3.85185988875507E-34,0.));
#113965=DIRECTION('center_axis',(3.85185988875507E-34,-1.,0.));
#113966=DIRECTION('ref_axis',(0.,0.,-1.));
#113967=DIRECTION('center_axis',(-3.85185988875507E-34,1.,0.));
#113968=DIRECTION('ref_axis',(0.,0.,-1.));
#113969=DIRECTION('center_axis',(-3.85185988875507E-34,1.,0.));
#113970=DIRECTION('ref_axis',(1.,3.85185988875507E-34,0.));
#113971=DIRECTION('center_axis',(3.85185988875507E-34,-1.,0.));
#113972=DIRECTION('ref_axis',(-1.,-3.85185988875507E-34,0.));
#113973=DIRECTION('',(3.85185988875507E-34,-1.,0.));
#113974=DIRECTION('center_axis',(3.85185988875507E-34,-1.,0.));
#113975=DIRECTION('ref_axis',(0.,0.,-1.));
#113976=DIRECTION('',(3.85185988875507E-34,-1.,0.));
#113977=DIRECTION('center_axis',(-3.85185988875507E-34,1.,0.));
#113978=DIRECTION('ref_axis',(0.,0.,-1.));
#113979=DIRECTION('center_axis',(0.333333332905692,1.28395329460448E-34,
0.942809041733257));
#113980=DIRECTION('ref_axis',(0.942809041733257,3.63156833060794E-34,-0.333333332905692));
#113981=DIRECTION('',(0.942809041733257,3.63156833060794E-34,-0.333333332905692));
#113982=DIRECTION('',(-0.942809041733257,-3.63156833060794E-34,0.333333332905692));
#113983=DIRECTION('center_axis',(3.85185988875507E-34,-1.,0.));
#113984=DIRECTION('ref_axis',(-1.,-3.85185988875507E-34,0.));
#113985=DIRECTION('',(3.85185988875507E-34,-1.,0.));
#113986=DIRECTION('center_axis',(3.85185988875507E-34,-1.,0.));
#113987=DIRECTION('ref_axis',(0.,0.,-1.));
#113988=DIRECTION('center_axis',(-3.85185988875507E-34,1.,0.));
#113989=DIRECTION('ref_axis',(0.,0.,-1.));
#113990=DIRECTION('center_axis',(3.85185988875507E-34,-1.,0.));
#113991=DIRECTION('ref_axis',(0.914659120962055,3.52313877991771E-34,-0.40422604127013));
#113992=DIRECTION('',(3.85185988875507E-34,-1.,0.));
#113993=DIRECTION('center_axis',(-3.85185988875507E-34,1.,0.));
#113994=DIRECTION('ref_axis',(0.,0.,-1.));
#113995=DIRECTION('center_axis',(-0.333333332905692,-1.28395329460448E-34,
0.942809041733257));
#113996=DIRECTION('ref_axis',(0.942809041733257,3.63156833060794E-34,0.333333332905692));
#113997=DIRECTION('',(3.85185988875507E-34,-1.,0.));
#113998=DIRECTION('',(0.942809041733257,3.63156833060794E-34,0.333333332905692));
#113999=DIRECTION('',(-0.942809041733257,-3.63156833060794E-34,-0.333333332905692));
#114000=DIRECTION('center_axis',(3.85185988875507E-34,-1.,0.));
#114001=DIRECTION('ref_axis',(-1.,-3.85185988875507E-34,0.));
#114002=DIRECTION('',(3.85185988875507E-34,-1.,0.));
#114003=DIRECTION('center_axis',(3.85185988875507E-34,-1.,0.));
#114004=DIRECTION('ref_axis',(0.,0.,-1.));
#114005=DIRECTION('center_axis',(-3.85185988875507E-34,1.,0.));
#114006=DIRECTION('ref_axis',(0.,0.,-1.));
#114007=DIRECTION('center_axis',(3.85185988875507E-34,-1.,0.));
#114008=DIRECTION('ref_axis',(-1.,-3.85185988875507E-34,0.));
#114009=DIRECTION('center_axis',(-3.85185988875507E-34,1.,0.));
#114010=DIRECTION('ref_axis',(0.,0.,-1.));
#114011=DIRECTION('center_axis',(3.85185988875507E-34,-1.,0.));
#114012=DIRECTION('ref_axis',(0.,0.,-1.));
#114013=DIRECTION('center_axis',(3.85185988875507E-34,-1.,0.));
#114014=DIRECTION('ref_axis',(-1.,-3.85185988875507E-34,0.));
#114015=DIRECTION('center_axis',(-3.85185988875507E-34,1.,0.));
#114016=DIRECTION('ref_axis',(-0.914659120976061,0.,0.404226041238437));
#114017=DIRECTION('center_axis',(0.388215488117679,1.49535166687396E-34,
-0.921568627279354));
#114018=DIRECTION('ref_axis',(-0.921568627279354,-3.54975323015241E-34,
-0.388215488117679));
#114019=DIRECTION('center_axis',(0.942809041733257,3.63156833060794E-34,
0.333333332905692));
#114020=DIRECTION('ref_axis',(-0.333333332905692,-1.28395329460448E-34,
0.942809041733257));
#114021=DIRECTION('center_axis',(-0.942809041733257,-3.63156833060794E-34,
-0.333333332905692));
#114022=DIRECTION('ref_axis',(0.235702261544926,-0.707106776831155,-0.666666670879881));
#114023=DIRECTION('center_axis',(0.942809041733257,3.63156833060794E-34,
0.333333332905692));
#114024=DIRECTION('ref_axis',(-0.333333332905692,-1.28395329460448E-34,
0.942809041733257));
#114025=DIRECTION('center_axis',(-3.85185988875507E-34,1.,0.));
#114026=DIRECTION('ref_axis',(1.,0.,0.));
#114027=DIRECTION('center_axis',(-3.85185988875507E-34,1.,0.));
#114028=DIRECTION('ref_axis',(1.,0.,0.));
#114029=DIRECTION('center_axis',(0.402255287051866,1.54943100523474E-34,
-0.915527544118046));
#114030=DIRECTION('ref_axis',(-0.915527544118046,-3.52648382423874E-34,
-0.402255287051866));
#114031=DIRECTION('center_axis',(-3.85185988875507E-34,1.,0.));
#114032=DIRECTION('ref_axis',(1.,0.,0.));
#114033=DIRECTION('center_axis',(0.402255287051866,1.54943100523474E-34,
0.915527544118046));
#114034=DIRECTION('ref_axis',(-0.915527544118046,-3.52648382423874E-34,
0.402255287051866));
#114035=DIRECTION('center_axis',(-0.942809041733257,-3.63156833060794E-34,
0.333333332905692));
#114036=DIRECTION('ref_axis',(0.333333332905692,1.28395329460448E-34,0.942809041733257));
#114037=DIRECTION('center_axis',(-0.942809041307877,-3.63156832896943E-34,
0.333333334108851));
#114038=DIRECTION('ref_axis',(0.333333334108851,1.28395329923887E-34,0.942809041307877));
#114039=DIRECTION('center_axis',(-3.85185988875507E-34,1.,0.));
#114040=DIRECTION('ref_axis',(1.,0.,0.));
#114041=DIRECTION('center_axis',(-3.85185988875507E-34,1.,0.));
#114042=DIRECTION('ref_axis',(1.,0.,0.));
#114043=DIRECTION('center_axis',(0.942809041733257,3.63156833060794E-34,
0.333333332905692));
#114044=DIRECTION('ref_axis',(0.333333332905692,1.28395329460448E-34,-0.942809041733257));
#114045=DIRECTION('center_axis',(-0.402255287051866,-1.54943100523474E-34,
0.915527544118046));
#114046=DIRECTION('ref_axis',(0.915527544118046,3.52648382423874E-34,0.402255287051866));
#114047=DIRECTION('center_axis',(-3.85185988875507E-34,1.,0.));
#114048=DIRECTION('ref_axis',(1.,0.,0.));
#114049=DIRECTION('center_axis',(-0.402255287051866,-1.54943100523474E-34,
-0.915527544118046));
#114050=DIRECTION('ref_axis',(0.915527544118046,3.52648382423874E-34,-0.402255287051866));
#114051=DIRECTION('center_axis',(0.942809041733257,3.63156833060794E-34,
0.333333332905692));
#114052=DIRECTION('ref_axis',(0.333333332905692,1.28395329460448E-34,-0.942809041733257));
#114053=DIRECTION('center_axis',(-3.85185988875507E-34,1.,0.));
#114054=DIRECTION('ref_axis',(1.,0.,0.));
#114055=DIRECTION('center_axis',(-0.942809041733257,-3.63156833060794E-34,
0.333333332905692));
#114056=DIRECTION('ref_axis',(-0.333333332905692,-1.28395329460448E-34,
-0.942809041733257));
#114057=DIRECTION('center_axis',(0.942809041733257,3.63156833060794E-34,
-0.333333332905692));
#114058=DIRECTION('ref_axis',(-0.333333332905692,-1.28395329460448E-34,
-0.942809041733257));
#114059=DIRECTION('center_axis',(-0.942809041733257,-3.63156833060794E-34,
0.333333332905692));
#114060=DIRECTION('ref_axis',(-0.333333332905692,-1.28395329460448E-34,
-0.942809041733257));
#114061=DIRECTION('center_axis',(-3.85185988875507E-34,1.,0.));
#114062=DIRECTION('ref_axis',(1.,0.,0.));
#114063=DIRECTION('center_axis',(-0.388215488966968,-1.4953516701453E-34,
-0.921568626921586));
#114064=DIRECTION('ref_axis',(-0.921568626921586,-3.54975322877434E-34,
0.388215488966968));
#114065=DIRECTION('center_axis',(-3.85185988875507E-34,1.,0.));
#114066=DIRECTION('ref_axis',(-0.914659121133649,0.,-0.404226040881857));
#114067=DIRECTION('center_axis',(-3.85185988875507E-34,1.,0.));
#114068=DIRECTION('ref_axis',(1.,3.85185988875507E-34,0.));
#114069=DIRECTION('center_axis',(-3.85185988875507E-34,1.,0.));
#114070=DIRECTION('ref_axis',(1.,3.85185988875507E-34,0.));
#145873=CARTESIAN_POINT('',(0.,0.,0.));
#145874=CARTESIAN_POINT('Origin',(1.11022302462516E-15,-1.77635683940025E-14,
2.22044604925031E-15));
#145875=CARTESIAN_POINT('',(8.993316745,-1.00000000000002,-0.346776472999999));
#145876=CARTESIAN_POINT('',(8.993316745,0.999999999999982,-0.346776472999999));
#145877=CARTESIAN_POINT('Ctrl Pts',(8.99331674501319,-0.999999999990532,
-0.346776473489777));
#145878=CARTESIAN_POINT('Ctrl Pts',(8.92005828617723,-0.888963444672732,
-0.346598504102869));
#145879=CARTESIAN_POINT('Ctrl Pts',(8.85904637943913,-0.76995646962542,
-0.346446577592176));
#145880=CARTESIAN_POINT('Ctrl Pts',(8.72757931577561,-0.424051722950309,
-0.34611575375876));
#145881=CARTESIAN_POINT('Ctrl Pts',(8.68754893604535,-0.18879105880841,
-0.346011201242058));
#145882=CARTESIAN_POINT('Ctrl Pts',(8.69992957774455,0.283921315910095,
-0.346043086203101));
#145883=CARTESIAN_POINT('Ctrl Pts',(8.75224857096735,0.516830885584916,
-0.346179200855117));
#145884=CARTESIAN_POINT('Ctrl Pts',(8.88881765021319,0.826237684539586,
-0.346520446328741));
#145885=CARTESIAN_POINT('Ctrl Pts',(8.93754891983208,0.915473689936097,
-0.346640994723032));
#145886=CARTESIAN_POINT('Ctrl Pts',(8.99331674501319,0.999999999990496,
-0.346776473489776));
#145887=CARTESIAN_POINT('',(8.988197099,-1.00000000000002,-0.460774244));
#145888=CARTESIAN_POINT('Origin',(1.11022302462516E-15,-1.00000000000002,
2.22044604925031E-15));
#145889=CARTESIAN_POINT('',(8.988197099,0.999999999999982,-0.460774244));
#145890=CARTESIAN_POINT('Ctrl Pts',(8.9881970991918,0.999999999893166,-0.460774243665515));
#145891=CARTESIAN_POINT('Ctrl Pts',(8.91521760434871,0.888963444601223,
-0.454384658959212));
#145892=CARTESIAN_POINT('Ctrl Pts',(8.85443769504401,0.76995646958464,-0.449066908687326));
#145893=CARTESIAN_POINT('Ctrl Pts',(8.72347022432541,0.424051722946438,
-0.43761178395344));
#145894=CARTESIAN_POINT('Ctrl Pts',(8.6835916231211,0.18879105880802,-0.434127619986626));
#145895=CARTESIAN_POINT('Ctrl Pts',(8.69592528214153,-0.28392131590547,
-0.435205655554323));
#145896=CARTESIAN_POINT('Ctrl Pts',(8.74804585570079,-0.516830885578334,
-0.439759927270131));
#145897=CARTESIAN_POINT('Ctrl Pts',(8.88409573697414,-0.826237684498686,
-0.451662013470527));
#145898=CARTESIAN_POINT('Ctrl Pts',(8.93264163468216,-0.915473689865194,
-0.455910187711914));
#145899=CARTESIAN_POINT('Ctrl Pts',(8.9881970991918,-0.999999999893202,
-0.460774243665515));
#145900=CARTESIAN_POINT('Origin',(1.11022302462516E-15,0.999999999999982,
2.22044604925031E-15));
#145901=CARTESIAN_POINT('Origin',(1.11022302462516E-15,-1.77635683940025E-14,
2.22044604925031E-15));
#145902=CARTESIAN_POINT('',(8.926027492,-1.00000000000002,-1.151535151));
#145903=CARTESIAN_POINT('',(8.926027492,0.999999999999982,-1.151535151));
#145904=CARTESIAN_POINT('Ctrl Pts',(8.92602749221155,-0.999999999831737,
-1.15153515148245));
#145905=CARTESIAN_POINT('Ctrl Pts',(8.85307990349065,-0.88896344455843,
-1.14479106093982));
#145906=CARTESIAN_POINT('Ctrl Pts',(8.79232723137321,-0.769956469564023,
-1.1391706808964));
#145907=CARTESIAN_POINT('Ctrl Pts',(8.66141907029811,-0.42405172294863,
-1.12705657215028));
#145908=CARTESIAN_POINT('Ctrl Pts',(8.6215592131229,-0.188791058808235,
-1.12336414496197));
#145909=CARTESIAN_POINT('Ctrl Pts',(8.63388715585244,0.283921315908099,
-1.1245056937277));
#145910=CARTESIAN_POINT('Ctrl Pts',(8.68598332696715,0.516830885582071,
-1.1293310988108));
#145911=CARTESIAN_POINT('Ctrl Pts',(8.82197203021842,0.826237684479057,
-1.14191292839256));
#145912=CARTESIAN_POINT('Ctrl Pts',(8.87049631616405,0.915473689823285,
-1.14640122881592));
#145913=CARTESIAN_POINT('Ctrl Pts',(8.92602749221155,0.999999999831702,
-1.15153515148245));
#145914=CARTESIAN_POINT('',(8.910709775,-1.00000000000002,-1.264615079));
#145915=CARTESIAN_POINT('Origin',(1.11022302462516E-15,-1.00000000000002,
2.22044604925031E-15));
#145916=CARTESIAN_POINT('',(8.910709775,0.999999999999982,-1.264615079));
#145917=CARTESIAN_POINT('Ctrl Pts',(8.9107097753288,0.999999999842809,-1.26461507851505));
#145918=CARTESIAN_POINT('Ctrl Pts',(8.83859683244853,0.888963444565197,
-1.25170938491645));
#145919=CARTESIAN_POINT('Ctrl Pts',(8.7785382846604,0.769956469565656,-1.24096477327833));
#145920=CARTESIAN_POINT('Ctrl Pts',(8.64912487994753,0.424051722946349,
-1.21781592994151));
#145921=CARTESIAN_POINT('Ctrl Pts',(8.6097191363179,0.188791058808013,-1.21077110194112));
#145922=CARTESIAN_POINT('Ctrl Pts',(8.6219065092898,-0.28392131590536,-1.21295037832583));
#145923=CARTESIAN_POINT('Ctrl Pts',(8.67340901897361,-0.516830885578179,
-1.22215836807797));
#145924=CARTESIAN_POINT('Ctrl Pts',(8.8078443086326,-0.82623768448008,-1.24620795731553));
#145925=CARTESIAN_POINT('Ctrl Pts',(8.85581397141433,-0.915473689829693,
-1.25479065037674));
#145926=CARTESIAN_POINT('Ctrl Pts',(8.9107097753288,-0.999999999842844,
-1.26461507851505));
#145927=CARTESIAN_POINT('Origin',(1.11022302462516E-15,0.999999999999982,
2.22044604925031E-15));
#145928=CARTESIAN_POINT('Origin',(1.11022302462516E-15,-1.77635683940025E-14,
2.22044604925031E-15));
#145929=CARTESIAN_POINT('',(8.786871115,-1.00000000000002,-1.947022345));
#145930=CARTESIAN_POINT('',(8.786871115,0.999999999999982,-1.947022345));
#145931=CARTESIAN_POINT('Ctrl Pts',(8.78687111484236,-1.00000000011924,
-1.9470223448582));
#145932=CARTESIAN_POINT('Ctrl Pts',(8.71482172720569,-0.888963444765539,
-1.93376643256629));
#145933=CARTESIAN_POINT('Ctrl Pts',(8.65481743440953,-0.769956469675546,
-1.92272285094909));
#145934=CARTESIAN_POINT('Ctrl Pts',(8.52552217140722,-0.424051722951982,
-1.89892299290974));
#145935=CARTESIAN_POINT('Ctrl Pts',(8.48615376492162,-0.188791058808556,
-1.89167242028617));
#145936=CARTESIAN_POINT('Ctrl Pts',(8.49832975133559,0.283921315912148,
-1.89391444178229));
#145937=CARTESIAN_POINT('Ctrl Pts',(8.54978365260218,0.516830885587828,
-1.90339028599331));
#145938=CARTESIAN_POINT('Ctrl Pts',(8.68409707884376,0.826237684589113,
-1.92811139825368));
#145939=CARTESIAN_POINT('Ctrl Pts',(8.73202369219063,0.915473690027751,
-1.9369313135815));
#145940=CARTESIAN_POINT('Ctrl Pts',(8.78687111484236,1.0000000001192,-1.9470223448582));
#145941=CARTESIAN_POINT('',(8.761478656,-1.00000000000002,-2.058273976));
#145942=CARTESIAN_POINT('Origin',(1.11022302462516E-15,-1.00000000000002,
2.22044604925031E-15));
#145943=CARTESIAN_POINT('',(8.761478656,0.999999999999982,-2.058273976));
#145944=CARTESIAN_POINT('Ctrl Pts',(8.76147865610178,1.00000000003545,-2.05827397542385));
#145945=CARTESIAN_POINT('Ctrl Pts',(8.69081287612847,0.888963444702555,
-2.03895608197732));
#145946=CARTESIAN_POINT('Ctrl Pts',(8.63195924591628,0.769956469637271,
-2.02287111825923));
#145947=CARTESIAN_POINT('Ctrl Pts',(8.50514186781519,0.424051722945794,
-1.9882149371944));
#145948=CARTESIAN_POINT('Ctrl Pts',(8.4665262536374,0.188791058807998,-1.97766616597551));
#145949=CARTESIAN_POINT('Ctrl Pts',(8.47846921499966,-0.283921315904603,
-1.98092913692443));
#145950=CARTESIAN_POINT('Ctrl Pts',(8.52893899288346,-0.516830885577122,
-1.9947167073906));
#145951=CARTESIAN_POINT('Ctrl Pts',(8.66067729706199,-0.826237684549968,
-2.03072016651486));
#145952=CARTESIAN_POINT('Ctrl Pts',(8.70768450145157,-0.915473689964895,
-2.04356827560745));
#145953=CARTESIAN_POINT('Ctrl Pts',(8.76147865610178,-1.00000000003548,
-2.05827397542385));
#145954=CARTESIAN_POINT('Origin',(1.11022302462516E-15,0.999999999999982,
2.22044604925031E-15));
#145955=CARTESIAN_POINT('Origin',(1.11022302462516E-15,-1.77635683940025E-14,
2.22044604925031E-15));
#145956=CARTESIAN_POINT('',(8.576968018,-1.00000000000002,-2.726833259));
#145957=CARTESIAN_POINT('',(8.576968018,0.999999999999982,-2.726833259));
#145958=CARTESIAN_POINT('Ctrl Pts',(8.57696801776425,-1.00000000013926,
-2.72683325905983));
#145959=CARTESIAN_POINT('Ctrl Pts',(8.50639693059222,-0.88896344478025,
-2.70717225385519));
#145960=CARTESIAN_POINT('Ctrl Pts',(8.44762413645845,-0.769956469683949,
-2.69079438711029));
#145961=CARTESIAN_POINT('Ctrl Pts',(8.32098278099789,-0.42405172295278,
-2.65550040227742));
#145962=CARTESIAN_POINT('Ctrl Pts',(8.28242279646211,-0.188791058808601,
-2.64475006157633));
#145963=CARTESIAN_POINT('Ctrl Pts',(8.29434879267705,0.283921315913182,
-2.64807450436084));
#145964=CARTESIAN_POINT('Ctrl Pts',(8.34474614753761,0.51683088558928,-2.66212449376052));
#145965=CARTESIAN_POINT('Ctrl Pts',(8.47630288399607,0.826237684597597,
-2.69878584880073));
#145966=CARTESIAN_POINT('Ctrl Pts',(8.52324594777668,0.915473690042371,
-2.71186636624358));
#145967=CARTESIAN_POINT('Ctrl Pts',(8.57696801776425,1.00000000013922,-2.72683325905983));
#145968=CARTESIAN_POINT('',(8.541705262,-1.00000000000002,-2.835360862));
#145969=CARTESIAN_POINT('Origin',(1.11022302462516E-15,-1.00000000000002,
2.22044604925031E-15));
#145970=CARTESIAN_POINT('',(8.541705262,0.999999999999982,-2.835360862));
#145971=CARTESIAN_POINT('Ctrl Pts',(8.54170526175661,1.00000000003763,-2.83536086248987));
#145972=CARTESIAN_POINT('Ctrl Pts',(8.47305560404579,0.888963444707527,
-2.80978630556046));
#145973=CARTESIAN_POINT('Ctrl Pts',(8.41588074626889,0.769956469645603,
-2.78849049646969));
#145974=CARTESIAN_POINT('Ctrl Pts',(8.29268045374403,0.424051722952562,
-2.74260600893571));
#145975=CARTESIAN_POINT('Ctrl Pts',(8.25516587923031,0.188791058808566,
-2.72863822702008));
#145976=CARTESIAN_POINT('Ctrl Pts',(8.26676827128391,-0.283921315912958,
-2.73295862100441));
#145977=CARTESIAN_POINT('Ctrl Pts',(8.31579896440192,-0.516830885588957,
-2.75121476275006));
#145978=CARTESIAN_POINT('Ctrl Pts',(8.44377960372841,-0.826237684560067,
-2.7988822130079));
#145979=CARTESIAN_POINT('Ctrl Pts',(8.48944587531942,-0.915473689970773,
-2.81589229268048));
#145980=CARTESIAN_POINT('Ctrl Pts',(8.54170526175661,-1.00000000003766,
-2.83536086248987));
#145981=CARTESIAN_POINT('Origin',(1.11022302462516E-15,0.999999999999982,
2.22044604925031E-15));
#145982=CARTESIAN_POINT('Origin',(1.11022302462516E-15,-1.77635683940025E-14,
2.22044604925031E-15));
#145983=CARTESIAN_POINT('',(8.298008217,-1.00000000000002,-3.484689316));
#145984=CARTESIAN_POINT('',(8.298008217,0.999999999999982,-3.484689317));
#145985=CARTESIAN_POINT('Ctrl Pts',(8.29800821680649,-0.999999999999693,
-3.48468931651321));
#145986=CARTESIAN_POINT('Ctrl Pts',(8.22948362702784,-0.888963444677954,
-3.4587815172934));
#145987=CARTESIAN_POINT('Ctrl Pts',(8.17241553555906,-0.769956469625942,
-3.43720123040944));
#145988=CARTESIAN_POINT('Ctrl Pts',(8.04944772937248,-0.424051722947685,
-3.39069728525703));
#145989=CARTESIAN_POINT('Ctrl Pts',(8.0120066291036,-0.188791058808186,
-3.37653373191683));
#145990=CARTESIAN_POINT('Ctrl Pts',(8.02358661401111,0.283921315906866,
-3.38091382952584));
#145991=CARTESIAN_POINT('Ctrl Pts',(8.07252165260454,0.516830885580342,
-3.39942484183956));
#145992=CARTESIAN_POINT('Ctrl Pts',(8.2002624818134,0.826237684599015,-3.4477312639312));
#145993=CARTESIAN_POINT('Ctrl Pts',(8.24584403809067,0.915473690055275,
-3.4649670668361));
#145994=CARTESIAN_POINT('Ctrl Pts',(8.29800821690682,1.00000000016222,-3.48468931655114));
#145995=CARTESIAN_POINT('',(8.253159079,-1.00000000000002,-3.58961909));
#145996=CARTESIAN_POINT('Origin',(1.11022302462516E-15,-1.00000000000002,
2.22044604925031E-15));
#145997=CARTESIAN_POINT('',(8.253159079,0.999999999999982,-3.58961909));
#145998=CARTESIAN_POINT('Ctrl Pts',(8.25315907930141,0.999999999897839,
-3.58961908972884));
#145999=CARTESIAN_POINT('Ctrl Pts',(8.18707827057777,0.888963444607218,
-3.55799378058502));
#146000=CARTESIAN_POINT('Ctrl Pts',(8.13204252360867,0.769956469592238,
-3.53165858743165));
#146001=CARTESIAN_POINT('Ctrl Pts',(8.01345125301593,0.424051722951706,
-3.47491522827454));
#146002=CARTESIAN_POINT('Ctrl Pts',(7.97733976346943,0.188791058808487,
-3.45764089600619));
#146003=CARTESIAN_POINT('Ctrl Pts',(7.98850817057213,-0.283921315911917,
-3.46298392776071));
#146004=CARTESIAN_POINT('Ctrl Pts',(8.03570501260313,-0.516830885587481,
-3.48556165309702));
#146005=CARTESIAN_POINT('Ctrl Pts',(8.15889756217779,-0.826237684507598,
-3.54450930427714));
#146006=CARTESIAN_POINT('Ctrl Pts',(8.20285522296936,-0.915473689871846,
-3.56554439938598));
#146007=CARTESIAN_POINT('Ctrl Pts',(8.25315907930141,-0.999999999897875,
-3.58961908972884));
#146008=CARTESIAN_POINT('Origin',(1.11022302462516E-15,0.999999999999982,
2.22044604925031E-15));
#146009=CARTESIAN_POINT('Origin',(1.11022302462516E-15,-1.77635683940025E-14,
2.22044604925031E-15));
#146010=CARTESIAN_POINT('',(7.952237733,-1.00000000000002,-4.214488703));
#146011=CARTESIAN_POINT('',(7.952237733,0.999999999999982,-4.214488703));
#146012=CARTESIAN_POINT('Ctrl Pts',(7.95223773319635,-0.999999999775502,
-4.21448870337516));
#146013=CARTESIAN_POINT('Ctrl Pts',(7.88631136054351,-0.888963444517432,
-4.18254270450202));
#146014=CARTESIAN_POINT('Ctrl Pts',(7.83140745047794,-0.769956469541136,
-4.15593374925552));
#146015=CARTESIAN_POINT('Ctrl Pts',(7.71310325805549,-0.424051722947019,
-4.0985942661749));
#146016=CARTESIAN_POINT('Ctrl Pts',(7.6770824957803,-0.188791058808112,
-4.08113153678696));
#146017=CARTESIAN_POINT('Ctrl Pts',(7.68822323415081,0.283921315906083,
-4.08653202325389));
#146018=CARTESIAN_POINT('Ctrl Pts',(7.73530196031659,0.516830885579221,
-4.10935501871067));
#146019=CARTESIAN_POINT('Ctrl Pts',(7.85819838815941,0.826237684456182,
-4.1689175729596));
#146020=CARTESIAN_POINT('Ctrl Pts',(7.90205144095589,0.915473689782661,
-4.19016988875141));
#146021=CARTESIAN_POINT('Ctrl Pts',(7.95223773319635,0.999999999775467,
-4.21448870337516));
#146022=CARTESIAN_POINT('',(7.898163313,-1.00000000000002,-4.314975815));
#146023=CARTESIAN_POINT('Origin',(1.11022302462516E-15,-1.00000000000002,
2.22044604925031E-15));
#146024=CARTESIAN_POINT('',(7.898163313,0.999999999999982,-4.314975815));
#146025=CARTESIAN_POINT('Ctrl Pts',(7.89816331271264,1.00000000009806,-4.31497581519262));
#146026=CARTESIAN_POINT('Ctrl Pts',(7.83518339669397,0.88896344475189,-4.277554382208));
#146027=CARTESIAN_POINT('Ctrl Pts',(7.78272987593037,0.769956469670873,
-4.24639184046861));
#146028=CARTESIAN_POINT('Ctrl Pts',(7.66970245438489,0.424051722954895,
-4.17924647387125));
#146029=CARTESIAN_POINT('Ctrl Pts',(7.63528479827936,0.188791058808738,
-4.15880467402876));
#146030=CARTESIAN_POINT('Ctrl Pts',(7.64592929898681,-0.283921315915892,
-4.16512732459995));
#146031=CARTESIAN_POINT('Ctrl Pts',(7.69091228871913,-0.516830885593102,
-4.19184485094197));
#146032=CARTESIAN_POINT('Ctrl Pts',(7.80832487464018,-0.826237684585495,
-4.26159809119923));
#146033=CARTESIAN_POINT('Ctrl Pts',(7.85022000346808,-0.915473690014823,
-4.28648883954431));
#146034=CARTESIAN_POINT('Ctrl Pts',(7.89816331271264,-1.00000000009809,
-4.31497581519262));
#146035=CARTESIAN_POINT('Origin',(1.11022302462516E-15,0.999999999999982,
2.22044604925031E-15));
#146036=CARTESIAN_POINT('Origin',(1.11022302462516E-15,-1.77635683940025E-14,
2.22044604925031E-15));
#146037=CARTESIAN_POINT('',(7.542440507,-1.00000000000002,-4.910355505));
#146038=CARTESIAN_POINT('',(7.542440507,0.999999999999982,-4.910355506));
#146039=CARTESIAN_POINT('Ctrl Pts',(7.54244050699415,-0.999999999713361,
-4.91035550585342));
#146040=CARTESIAN_POINT('Ctrl Pts',(7.47964315180284,-0.888963444471707,
-4.87262851771894));
#146041=CARTESIAN_POINT('Ctrl Pts',(7.42734547710069,-0.769956469514917,
-4.84120513376688));
#146042=CARTESIAN_POINT('Ctrl Pts',(7.31465741420511,-0.424051722944403,
-4.77349177656747));
#146043=CARTESIAN_POINT('Ctrl Pts',(7.2803470079185,-0.18879105880792,-4.75287047076504));
#146044=CARTESIAN_POINT('Ctrl Pts',(7.29095880107796,0.283921315902789,
-4.75924786454684));
#146045=CARTESIAN_POINT('Ctrl Pts',(7.33580216459886,0.516830885574571,
-4.78619908580148));
#146046=CARTESIAN_POINT('Ctrl Pts',(7.4528647013947,0.826237684516619,-4.85653820956603));
#146047=CARTESIAN_POINT('Ctrl Pts',(7.49463617183292,0.915473689903834,
-4.88163592714012));
#146048=CARTESIAN_POINT('Ctrl Pts',(7.54244050712803,0.99999999995005,-4.91035550593385));
#146049=CARTESIAN_POINT('',(7.47957618,-1.00000000000002,-5.005590891));
#146050=CARTESIAN_POINT('Origin',(1.11022302462516E-15,-1.00000000000002,
2.22044604925031E-15));
#146051=CARTESIAN_POINT('',(7.47957618,0.999999999999982,-5.005590891));
#146052=CARTESIAN_POINT('Ctrl Pts',(7.47957617982888,1.00000000003923,-5.00559089113518));
#146053=CARTESIAN_POINT('Ctrl Pts',(7.42020423385493,0.888963444707324,
-4.96267462967732));
#146054=CARTESIAN_POINT('Ctrl Pts',(7.37075526427221,0.769956469643232,
-4.92693564180633));
#146055=CARTESIAN_POINT('Ctrl Pts',(7.2642017221897,0.424051722949885,-4.84992888272495));
#146056=CARTESIAN_POINT('Ctrl Pts',(7.23175501026859,0.188791058808343,
-4.82648420063957));
#146057=CARTESIAN_POINT('Ctrl Pts',(7.24178990131453,-0.283921315909651,
-4.83373556376861));
#146058=CARTESIAN_POINT('Ctrl Pts',(7.28419686214625,-0.516830885584273,
-4.8643777773319));
#146059=CARTESIAN_POINT('Ctrl Pts',(7.39488414722774,-0.826237684556975,
-4.94437499464598));
#146060=CARTESIAN_POINT('Ctrl Pts',(7.43437942908497,-0.915473689970184,
-4.9729209905592));
#146061=CARTESIAN_POINT('Ctrl Pts',(7.47957617982888,-1.00000000003927,
-5.00559089113518));
#146062=CARTESIAN_POINT('Origin',(1.11022302462516E-15,0.999999999999982,
2.22044604925031E-15));
#146063=CARTESIAN_POINT('Origin',(1.11022302462516E-15,-1.77635683940025E-14,
2.22044604925031E-15));
#146064=CARTESIAN_POINT('',(7.071915986,-1.00000000000002,-5.566687012));
#146065=CARTESIAN_POINT('',(7.071915985,0.999999999999982,-5.566687013));
#146066=CARTESIAN_POINT('Ctrl Pts',(7.07191598537279,-1.00000000011093,
-5.56668701257384));
#146067=CARTESIAN_POINT('Ctrl Pts',(7.01275325493728,-0.888963444757714,
-5.52348279059387));
#146068=CARTESIAN_POINT('Ctrl Pts',(6.96348288566105,-0.769956469668278,
-5.48749798046137));
#146069=CARTESIAN_POINT('Ctrl Pts',(6.85731825030078,-0.424051722948234,
-5.4099559371812));
#146070=CARTESIAN_POINT('Ctrl Pts',(6.82499444723148,-0.188791058808213,
-5.38634208557447));
#146071=CARTESIAN_POINT('Ctrl Pts',(6.83499185525839,0.283921315907583,
-5.39364503965271));
#146072=CARTESIAN_POINT('Ctrl Pts',(6.87723880372388,0.516830885581344,
-5.4245074913437));
#146073=CARTESIAN_POINT('Ctrl Pts',(6.98752493069896,0.826237684544213,
-5.50505685541548));
#146074=CARTESIAN_POINT('Ctrl Pts',(7.02687849941884,0.915473689949043,
-5.53379790271953));
#146075=CARTESIAN_POINT('Ctrl Pts',(7.07191598531944,1.00000000001076,-5.56668701253488));
#146076=CARTESIAN_POINT('',(7.000767897,-1.00000000000002,-5.655903894));
#146077=CARTESIAN_POINT('Origin',(1.11022302462516E-15,-1.00000000000002,
2.22044604925031E-15));
#146078=CARTESIAN_POINT('',(7.000767897,0.999999999999982,-5.655903894));
#146079=CARTESIAN_POINT('Ctrl Pts',(7.00076789681102,1.00000000017972,-5.65590389380216));
#146080=CARTESIAN_POINT('Ctrl Pts',(6.94548194883083,0.888963444807022,
-5.60783834035334));
#146081=CARTESIAN_POINT('Ctrl Pts',(6.89943566441819,0.769956469694419,
-5.56781065565214));
#146082=CARTESIAN_POINT('Ctrl Pts',(6.8002139082344,0.424051722948536,-5.48156251723961));
#146083=CARTESIAN_POINT('Ctrl Pts',(6.76999938234043,0.188791058808216,
-5.4553037157138));
#146084=CARTESIAN_POINT('Ctrl Pts',(6.77934386868416,-0.283921315908016,
-5.46342540768646));
#146085=CARTESIAN_POINT('Ctrl Pts',(6.81883336470601,-0.516830885581949,
-5.49774559537489));
#146086=CARTESIAN_POINT('Ctrl Pts',(6.92190416004712,-0.826237684606703,
-5.58734269918266));
#146087=CARTESIAN_POINT('Ctrl Pts',(6.958681602184,-0.9154736900682,-5.61931410710659));
#146088=CARTESIAN_POINT('Ctrl Pts',(7.00076789681102,-1.00000000017975,
-5.65590389380216));
#146089=CARTESIAN_POINT('Origin',(1.11022302462516E-15,0.999999999999982,
2.22044604925031E-15));
#146090=CARTESIAN_POINT('Origin',(1.11022302462516E-15,-1.77635683940025E-14,
2.22044604925031E-15));
#146091=CARTESIAN_POINT('',(6.544452554,-1.00000000000002,-6.178198829));
#146092=CARTESIAN_POINT('',(6.544452554,0.999999999999982,-6.178198829));
#146093=CARTESIAN_POINT('Ctrl Pts',(6.54445255416351,-1.0000000000805,-6.17819882862886));
#146094=CARTESIAN_POINT('Ctrl Pts',(6.4894007921,-0.888963444736671,-6.12986522787583));
#146095=CARTESIAN_POINT('Ctrl Pts',(6.44355442436668,-0.769956469658398,
-6.08960872015794));
#146096=CARTESIAN_POINT('Ctrl Pts',(6.34476799180017,-0.424051722949613,
-6.00286231379505));
#146097=CARTESIAN_POINT('Ctrl Pts',(6.31469104420046,-0.188791058808339,
-5.97644604124083));
#146098=CARTESIAN_POINT('Ctrl Pts',(6.32399357384459,0.283921315909266,
-5.98461575652057));
#146099=CARTESIAN_POINT('Ctrl Pts',(6.36330395967154,0.516830885583735,
-6.01914095232269));
#146100=CARTESIAN_POINT('Ctrl Pts',(6.46592571779309,0.826237684571677,
-6.10925202055844));
#146101=CARTESIAN_POINT('Ctrl Pts',(6.50254453300505,0.915473689998984,
-6.14140499157264));
#146102=CARTESIAN_POINT('Ctrl Pts',(6.54445255416351,1.00000000008047,-6.17819882862886));
#146103=CARTESIAN_POINT('',(6.465593548,-1.00000000000002,-6.260678883));
#146104=CARTESIAN_POINT('Origin',(1.11022302462516E-15,-1.00000000000002,
2.22044604925031E-15));
#146105=CARTESIAN_POINT('',(6.465593547,0.999999999999982,-6.260678883));
#146106=CARTESIAN_POINT('Ctrl Pts',(6.46559354762128,0.99999999981135,-6.26067888279958));
#146107=CARTESIAN_POINT('Ctrl Pts',(6.41483872768217,0.888963444543264,
-6.20785103304572));
#146108=CARTESIAN_POINT('Ctrl Pts',(6.37256586612411,0.769956469555061,
-6.1638569309814));
#146109=CARTESIAN_POINT('Ctrl Pts',(6.28147477111903,0.424051722947445,
-6.06906183260181));
#146110=CARTESIAN_POINT('Ctrl Pts',(6.25373570084517,0.18879105880813,-6.04020033207072));
#146111=CARTESIAN_POINT('Ctrl Pts',(6.26231454617831,-0.283921315906656,
-6.04912696179709));
#146112=CARTESIAN_POINT('Ctrl Pts',(6.29856863119255,-0.516830885580026,
-6.08684879763255));
#146113=CARTESIAN_POINT('Ctrl Pts',(6.39319307134218,-0.826237684586883,
-6.18532440469951));
#146114=CARTESIAN_POINT('Ctrl Pts',(6.4269565633907,-0.915473690032379,
-6.22046380962379));
#146115=CARTESIAN_POINT('Ctrl Pts',(6.46559354776685,-1.00000000012986,
-6.26067888295109));
#146116=CARTESIAN_POINT('Origin',(1.11022302462516E-15,0.999999999999982,
2.22044604925031E-15));
#146117=CARTESIAN_POINT('Origin',(1.11022302462516E-15,-1.77635683940025E-14,
2.22044604925031E-15));
#146118=CARTESIAN_POINT('',(5.964297039,-1.00000000000002,-6.739967421));
#146119=CARTESIAN_POINT('',(5.964297039,0.999999999999982,-6.73996742));
#146120=CARTESIAN_POINT('Ctrl Pts',(5.96429703935934,-1.00000000016049,
-6.73996742032238));
#146121=CARTESIAN_POINT('Ctrl Pts',(5.91379949005691,-0.888963444794065,
-6.68689359451439));
#146122=CARTESIAN_POINT('Ctrl Pts',(5.87174625183969,-0.769956469688926,
-6.64268951092948));
#146123=CARTESIAN_POINT('Ctrl Pts',(5.78113339231567,-0.42405172295009,
-6.54743717254365));
#146124=CARTESIAN_POINT('Ctrl Pts',(5.75354546207986,-0.188791058808368,
-6.51843116733989));
#146125=CARTESIAN_POINT('Ctrl Pts',(5.76207821484305,0.283921315909877,
-6.52740186607613));
#146126=CARTESIAN_POINT('Ctrl Pts',(5.79813553392257,0.516830885584594,
-6.56531182940824));
#146127=CARTESIAN_POINT('Ctrl Pts',(5.89226667310739,0.826237684479476,
-6.66425908042156));
#146128=CARTESIAN_POINT('Ctrl Pts',(5.92585590159545,0.915473689821208,
-6.69956509827456));
#146129=CARTESIAN_POINT('Ctrl Pts',(5.96429703920789,0.999999999827432,
-6.7399674201632));
#146130=CARTESIAN_POINT('',(5.87836204,-1.00000000000002,-6.815046568));
#146131=CARTESIAN_POINT('Origin',(1.11022302462516E-15,-1.00000000000002,
2.22044604925031E-15));
#146132=CARTESIAN_POINT('',(5.87836204,0.999999999999982,-6.815046568));
#146133=CARTESIAN_POINT('Ctrl Pts',(5.87836203971057,0.999999999954793,
-6.81504656831974));
#146134=CARTESIAN_POINT('Ctrl Pts',(5.8325469956454,0.888963444648912,-6.75788176096771));
#146135=CARTESIAN_POINT('Ctrl Pts',(5.79438791306315,0.769956469615795,
-6.71027545612482));
#146136=CARTESIAN_POINT('Ctrl Pts',(5.7121608910693,0.424051722953685,-6.60769663216305));
#146137=CARTESIAN_POINT('Ctrl Pts',(5.68712061508326,0.188791058808652,
-6.57646480847093));
#146138=CARTESIAN_POINT('Ctrl Pts',(5.69486474759318,-0.283921315914366,
-6.58612450397438));
#146139=CARTESIAN_POINT('Ctrl Pts',(5.72759152504514,-0.516830885590948,
-6.62694427389891));
#146140=CARTESIAN_POINT('Ctrl Pts',(5.81300774969049,-0.826237684531224,
-6.73350551647852));
#146141=CARTESIAN_POINT('Ctrl Pts',(5.84348544786606,-0.915473689913203,
-6.77152999653492));
#146142=CARTESIAN_POINT('Ctrl Pts',(5.87836203971057,-0.999999999954828,
-6.81504656831974));
#146143=CARTESIAN_POINT('Origin',(1.11022302462516E-15,0.999999999999982,
2.22044604925031E-15));
#146144=CARTESIAN_POINT('Origin',(1.11022302462516E-15,-1.77635683940025E-14,
2.22044604925031E-15));
#146145=CARTESIAN_POINT('',(5.336120511,-1.00000000000002,-7.247469758));
#146146=CARTESIAN_POINT('',(5.33612051,0.999999999999982,-7.247469758));
#146147=CARTESIAN_POINT('Ctrl Pts',(5.3361205102212,-1.00000000007198,-7.24746975847874));
#146148=CARTESIAN_POINT('Ctrl Pts',(5.29058375025361,-0.888963444727195,
-7.19008302691189));
#146149=CARTESIAN_POINT('Ctrl Pts',(5.25266222949664,-0.769956469647748,
-7.14228727279495));
#146150=CARTESIAN_POINT('Ctrl Pts',(5.17095250443963,-0.42405172294289,
-7.03929591826978));
#146151=CARTESIAN_POINT('Ctrl Pts',(5.14607571334355,-0.18879105880775,
-7.00793371972911));
#146152=CARTESIAN_POINT('Ctrl Pts',(5.15376998852219,0.28392131590102,-7.01763317512497));
#146153=CARTESIAN_POINT('Ctrl Pts',(5.18628392854452,0.516830885572041,
-7.05862267723458));
#146154=CARTESIAN_POINT('Ctrl Pts',(5.27116656029511,0.826237684454488,
-7.16560944591632));
#146155=CARTESIAN_POINT('Ctrl Pts',(5.30145576140191,0.915473689787592,
-7.20378424732816));
#146156=CARTESIAN_POINT('Ctrl Pts',(5.33612051010402,0.999999999786219,
-7.24746975833107));
#146157=CARTESIAN_POINT('',(5.243801419,-1.00000000000002,-7.314543504));
#146158=CARTESIAN_POINT('Origin',(1.11022302462516E-15,-1.00000000000002,
2.22044604925031E-15));
#146159=CARTESIAN_POINT('',(5.243801419,0.999999999999982,-7.314543505));
#146160=CARTESIAN_POINT('Ctrl Pts',(5.24380141936078,1.00000000025759,-7.31454350429201));
#146161=CARTESIAN_POINT('Ctrl Pts',(5.20329502701867,0.888963444859878,
-7.25350199664624));
#146162=CARTESIAN_POINT('Ctrl Pts',(5.16955695795366,0.769956469717499,
-7.20266678690974));
#146163=CARTESIAN_POINT('Ctrl Pts',(5.09685605273472,0.424051722943023,
-7.09313014161181));
#146164=CARTESIAN_POINT('Ctrl Pts',(5.07471618065862,0.188791058807761,
-7.05977945500722));
#146165=CARTESIAN_POINT('Ctrl Pts',(5.08156324912866,-0.283921315901189,
-7.07009444210696));
#146166=CARTESIAN_POINT('Ctrl Pts',(5.11049922219244,-0.516830885572283,
-7.11368348937601));
#146167=CARTESIAN_POINT('Ctrl Pts',(5.18601950998405,-0.826237684487119,
-7.22747239912402));
#146168=CARTESIAN_POINT('Ctrl Pts',(5.21296602575133,-0.915473689849889,
-7.26807580361716));
#146169=CARTESIAN_POINT('Ctrl Pts',(5.24380141922105,-0.999999999874605,
-7.31454350408144));
#146170=CARTESIAN_POINT('Origin',(1.11022302462516E-15,0.999999999999982,
2.22044604925031E-15));
#146171=CARTESIAN_POINT('Origin',(1.11022302462516E-15,-1.77635683940025E-14,
2.22044604925031E-15));
#146172=CARTESIAN_POINT('',(4.664980679,-1.00000000000002,-7.69661973));
#146173=CARTESIAN_POINT('',(4.664980679,0.999999999999982,-7.69661973));
#146174=CARTESIAN_POINT('Ctrl Pts',(4.6649806790278,-1.00000000012153,-7.69661972976142));
#146175=CARTESIAN_POINT('Ctrl Pts',(4.62477134369037,-0.888963444769274,
-7.6353821365611));
#146176=CARTESIAN_POINT('Ctrl Pts',(4.59128686224838,-0.769956469681019,
-7.58437953514421));
#146177=CARTESIAN_POINT('Ctrl Pts',(4.51913815048226,-0.424051722956118,
-7.47447839016348));
#146178=CARTESIAN_POINT('Ctrl Pts',(4.49717279187256,-0.188791058808884,
-7.44101250822752));
#146179=CARTESIAN_POINT('Ctrl Pts',(4.50396663967298,0.283921315917304,
-7.45136262598658));
#146180=CARTESIAN_POINT('Ctrl Pts',(4.53267541744313,0.516830885595124,
-7.49510164355729));
#146181=CARTESIAN_POINT('Ctrl Pts',(4.60762611656944,0.826237684595681,
-7.60926653553599));
#146182=CARTESIAN_POINT('Ctrl Pts',(4.6343714194336,0.915473690032042,-7.65000275956128));
#146183=CARTESIAN_POINT('Ctrl Pts',(4.6649806790278,1.0000000001215,-7.69661972976142));
#146184=CARTESIAN_POINT('',(4.567020791,-1.00000000000002,-7.755148038));
#146185=CARTESIAN_POINT('Origin',(1.11022302462516E-15,-1.00000000000002,
2.22044604925031E-15));
#146186=CARTESIAN_POINT('',(4.56702079017615,1.00000000014985,-7.75514803858119));
#146187=CARTESIAN_POINT('Ctrl Pts',(4.56702079103465,1.0000000001046,-7.7551480381945));
#146188=CARTESIAN_POINT('Ctrl Pts',(4.53214918409692,0.888963444751377,
-7.69072130073945));
#146189=CARTESIAN_POINT('Ctrl Pts',(4.50310376766113,0.769956469661911,
-7.63706648144992));
#146190=CARTESIAN_POINT('Ctrl Pts',(4.44051432410008,0.424051722944636,
-7.5214539396054));
#146191=CARTESIAN_POINT('Ctrl Pts',(4.42145311313639,0.188791058807902,
-7.48625291022913));
#146192=CARTESIAN_POINT('Ctrl Pts',(4.42734798900763,-0.283921315903169,
-7.49714013870893));
#146193=CARTESIAN_POINT('Ctrl Pts',(4.45226018228089,-0.516830885575091,
-7.54314750991511));
#146194=CARTESIAN_POINT('Ctrl Pts',(4.5172764883787,-0.826237684515359,
-7.66324792537742));
#146195=CARTESIAN_POINT('Ctrl Pts',(4.54047486428761,-0.915473689900841,
-7.7061033395637));
#146196=CARTESIAN_POINT('Ctrl Pts',(4.56702079098469,-0.999999999945535,
-7.75514803810218));
#146197=CARTESIAN_POINT('Origin',(1.11022302462516E-15,0.999999999999982,
2.22044604925031E-15));
#146198=CARTESIAN_POINT('Origin',(1.11022302462516E-15,-1.77635683940025E-14,
2.22044604925031E-15));
#146199=CARTESIAN_POINT('',(3.956281164,-1.00000000000002,-8.083801046));
#146200=CARTESIAN_POINT('',(3.956281165,0.999999999999982,-8.083801046));
#146201=CARTESIAN_POINT('Ctrl Pts',(3.95628116468507,-1.00000000001549,
-8.08380104560689));
#146202=CARTESIAN_POINT('Ctrl Pts',(3.92172299585936,-0.888963444693514,
-8.01920563994906));
#146203=CARTESIAN_POINT('Ctrl Pts',(3.89294515105064,-0.769956469641267,
-7.96540683425602));
#146204=CARTESIAN_POINT('Ctrl Pts',(3.83093835147929,-0.424051722956149,
-7.84948075832601));
#146205=CARTESIAN_POINT('Ctrl Pts',(3.81206127747473,-0.188791058808902,
-7.81418064062605));
#146206=CARTESIAN_POINT('Ctrl Pts',(3.81789999783811,0.283921315917307,
-7.82509808767561));
#146207=CARTESIAN_POINT('Ctrl Pts',(3.8425724672014,0.516830885595135,-7.87123445981978));
#146208=CARTESIAN_POINT('Ctrl Pts',(3.90698777483689,0.826237684636356,
-7.99165828639557));
#146209=CARTESIAN_POINT('Ctrl Pts',(3.92997384201674,0.91547369011003,-8.0346279488464));
#146210=CARTESIAN_POINT('Ctrl Pts',(3.95628116475256,1.0000000002323,-8.08380104573303));
#146211=CARTESIAN_POINT('',(3.853469197,-1.00000000000002,-8.133312679));
#146212=CARTESIAN_POINT('Origin',(1.11022302462516E-15,-1.00000000000002,
2.22044604925031E-15));
#146213=CARTESIAN_POINT('',(3.853469197,0.999999999999982,-8.13331268));
#146214=CARTESIAN_POINT('Ctrl Pts',(3.85346919706807,1.0000000001062,-8.13331267979544));
#146215=CARTESIAN_POINT('Ctrl Pts',(3.82451314113869,0.888963444756582,
-8.06601943872399));
#146216=CARTESIAN_POINT('Ctrl Pts',(3.80039423388955,0.769956469671447,
-8.00997700692796));
#146217=CARTESIAN_POINT('Ctrl Pts',(3.74842018528737,0.424051722952665,
-7.88921941276124));
#146218=CARTESIAN_POINT('Ctrl Pts',(3.73259110507323,0.18879105880854,-7.85245145861414));
#146219=CARTESIAN_POINT('Ctrl Pts',(3.73748632627965,-0.283921315913163,
-7.86382327090975));
#146220=CARTESIAN_POINT('Ctrl Pts',(3.758174161464,-0.516830885589227,-7.91187854173883));
#146221=CARTESIAN_POINT('Ctrl Pts',(3.81216301286461,-0.82623768443046,
-8.0373234849023));
#146222=CARTESIAN_POINT('Ctrl Pts',(3.83142646923125,-0.91547368972195,
-8.08208586210271));
#146223=CARTESIAN_POINT('Ctrl Pts',(3.85346919695796,-0.999999999683993,
-8.13331267953954));
#146224=CARTESIAN_POINT('Origin',(1.11022302462516E-15,0.999999999999982,
2.22044604925031E-15));
#146225=CARTESIAN_POINT('Origin',(1.11022302462516E-15,-1.77635683940025E-14,
2.22044604925031E-15));
#146226=CARTESIAN_POINT('',(3.215728,-1.00000000000002,-8.405896349));
#146227=CARTESIAN_POINT('',(3.215728,0.999999999999982,-8.405896349));
#146228=CARTESIAN_POINT('Ctrl Pts',(3.21572799910164,-1.00000000004898,
-8.40589634930077));
#146229=CARTESIAN_POINT('Ctrl Pts',(3.18709923874645,-0.888963444711018,
-8.33846321539938));
#146230=CARTESIAN_POINT('Ctrl Pts',(3.16325973277762,-0.769956469639689,
-8.28230136177404));
#146231=CARTESIAN_POINT('Ctrl Pts',(3.11189408755156,-0.424051722943416,
-8.16128372353288));
#146232=CARTESIAN_POINT('Ctrl Pts',(3.09625728521347,-0.188791058807824,
-8.12443358587799));
#146233=CARTESIAN_POINT('Ctrl Pts',(3.10109386820783,0.283921315901602,
-8.13583046134637));
#146234=CARTESIAN_POINT('Ctrl Pts',(3.12153138099901,0.516830885572883,
-8.18399272510011));
#146235=CARTESIAN_POINT('Ctrl Pts',(3.17489266307679,0.826237684551582,
-8.30970590433157));
#146236=CARTESIAN_POINT('Ctrl Pts',(3.19393442429636,0.915473689972814,
-8.35456303867882));
#146237=CARTESIAN_POINT('Ctrl Pts',(3.21572799910164,1.00000000004895,-8.40589634930077));
#146238=CARTESIAN_POINT('',(3.108891736,-1.00000000000002,-8.445992669));
#146239=CARTESIAN_POINT('Origin',(1.11022302462516E-15,-1.00000000000002,
2.22044604925031E-15));
#146240=CARTESIAN_POINT('',(3.108891736,0.999999999999982,-8.44599267));
#146241=CARTESIAN_POINT('Ctrl Pts',(3.10889173624931,1.00000000023755,-8.44599266953941));
#146242=CARTESIAN_POINT('Ctrl Pts',(3.08608436854417,0.888963444846535,
-8.37637473037447));
#146243=CARTESIAN_POINT('Ctrl Pts',(3.06708616180808,0.76995646971212,-8.31839590671147));
#146244=CARTESIAN_POINT('Ctrl Pts',(3.0261459728075,0.424051722944944,-8.19346552927423));
#146245=CARTESIAN_POINT('Ctrl Pts',(3.01367646984111,0.188791058807912,
-8.15542668428225));
#146246=CARTESIAN_POINT('Ctrl Pts',(3.01753262292283,-0.283921315903587,
-8.16719152125182));
#146247=CARTESIAN_POINT('Ctrl Pts',(3.03382953366586,-0.516830885575674,
-8.21690777894712));
#146248=CARTESIAN_POINT('Ctrl Pts',(3.07635624373366,-0.826237684462671,
-8.34668724102495));
#146249=CARTESIAN_POINT('Ctrl Pts',(3.09152968251005,-0.915473689799155,
-8.39299618100886));
#146250=CARTESIAN_POINT('Ctrl Pts',(3.10889173615958,-0.999999999800758,
-8.44599266926553));
#146251=CARTESIAN_POINT('Origin',(1.11022302462516E-15,0.999999999999982,
2.22044604925031E-15));
#146252=CARTESIAN_POINT('Origin',(1.11022302462516E-15,-1.77635683940025E-14,
2.22044604925031E-15));
#146253=CARTESIAN_POINT('',(2.449283685,-1.00000000000002,-8.660312317));
#146254=CARTESIAN_POINT('',(2.449283685,0.999999999999982,-8.660312317));
#146255=CARTESIAN_POINT('Ctrl Pts',(2.44928368492003,-0.999999999970373,
-8.66031231707298));
#146256=CARTESIAN_POINT('Ctrl Pts',(2.42681483511176,-0.88896344465865,
-8.5905843868621));
#146257=CARTESIAN_POINT('Ctrl Pts',(2.40810560977552,-0.76995646961857,
-8.53251166751632));
#146258=CARTESIAN_POINT('Ctrl Pts',(2.36779468507835,-0.42405172295094,
-8.40737682975315));
#146259=CARTESIAN_POINT('Ctrl Pts',(2.35552405280636,-0.188791058808441,
-8.36927336775524));
#146260=CARTESIAN_POINT('Ctrl Pts',(2.35931955709161,0.283921315910929,
-8.38105791071449));
#146261=CARTESIAN_POINT('Ctrl Pts',(2.37535756239453,0.516830885586086,
-8.4308582918873));
#146262=CARTESIAN_POINT('Ctrl Pts',(2.41723518504276,0.826237684533091,
-8.56084865527989));
#146263=CARTESIAN_POINT('Ctrl Pts',(2.4321793271706,0.915473689922331,-8.6072320982976));
#146264=CARTESIAN_POINT('Ctrl Pts',(2.44928368492003,0.999999999970337,
-8.66031231707298));
#146265=CARTESIAN_POINT('',(2.339283306,-1.00000000000002,-8.690670493));
#146266=CARTESIAN_POINT('Origin',(1.11022302462516E-15,-1.00000000000002,
2.22044604925031E-15));
#146267=CARTESIAN_POINT('',(2.339283305,0.999999999999982,-8.690670493));
#146268=CARTESIAN_POINT('Ctrl Pts',(2.33928330561053,1.00000000001403,-8.69067049283723));
#146269=CARTESIAN_POINT('Ctrl Pts',(2.322808257611,0.888963444688627,-8.61928837841982));
#146270=CARTESIAN_POINT('Ctrl Pts',(2.30908371374843,0.769956469632264,
-8.5598399743875));
#146271=CARTESIAN_POINT('Ctrl Pts',(2.27950701057719,0.424051722948505,
-8.4317426797122));
#146272=CARTESIAN_POINT('Ctrl Pts',(2.27049748192907,0.188791058808199,
-8.39273921030103));
#146273=CARTESIAN_POINT('Ctrl Pts',(2.27328351942049,-0.283921315908009,
-8.40480234839289));
#146274=CARTESIAN_POINT('Ctrl Pts',(2.28505829262577,-0.516830885581933,
-8.45577930686427));
#146275=CARTESIAN_POINT('Ctrl Pts',(2.31578046142091,-0.826237684583821,
-8.58884837992317));
#146276=CARTESIAN_POINT('Ctrl Pts',(2.32674171504669,-0.91547369002434,
-8.63633103035858));
#146277=CARTESIAN_POINT('Ctrl Pts',(2.33928330562587,-1.00000000011744,
-8.69067049290369));
#146278=CARTESIAN_POINT('Origin',(1.11022302462516E-15,0.999999999999982,
2.22044604925031E-15));
#146279=CARTESIAN_POINT('Origin',(1.11022302462516E-15,-1.77635683940025E-14,
2.22044604925031E-15));
#146280=CARTESIAN_POINT('',(1.663119178,-1.00000000000002,-8.845000543));
#146281=CARTESIAN_POINT('',(1.663119178,0.999999999999982,-8.845000543));
#146282=CARTESIAN_POINT('Ctrl Pts',(1.66311917835389,-1.00000000017414,
-8.84500054264957));
#146283=CARTESIAN_POINT('Ctrl Pts',(1.64699114496605,-0.888963444802729,
-8.77353922436293));
#146284=CARTESIAN_POINT('Ctrl Pts',(1.6335628358678,-0.769956469691643,
-8.71402320664169));
#146285=CARTESIAN_POINT('Ctrl Pts',(1.60463119142803,-0.424051722947924,
-8.58577868149685));
#146286=CARTESIAN_POINT('Ctrl Pts',(1.5958255251009,-0.188791058808183,
-8.54672868184126));
#146287=CARTESIAN_POINT('Ctrl Pts',(1.59854939151922,0.28392131590721,-8.55880601007474));
#146288=CARTESIAN_POINT('Ctrl Pts',(1.61005876079406,0.516830885580814,
-8.60984354526128));
#146289=CARTESIAN_POINT('Ctrl Pts',(1.64011555016049,0.826237684603748,
-8.74306448684239));
#146290=CARTESIAN_POINT('Ctrl Pts',(1.65084175181585,0.915473690063816,
-8.79060078636947));
#146291=CARTESIAN_POINT('Ctrl Pts',(1.66311917835389,1.00000000017411,-8.84500054264957));
#146292=CARTESIAN_POINT('',(1.550840341,-1.00000000000002,-8.865376147));
#146293=CARTESIAN_POINT('Origin',(1.11022302462516E-15,-1.00000000000002,
2.22044604925031E-15));
#146294=CARTESIAN_POINT('',(1.550840341,0.999999999999982,-8.865376147));
#146295=CARTESIAN_POINT('Ctrl Pts',(1.55084034140624,0.999999999808245,
-8.86537614723733));
#146296=CARTESIAN_POINT('Ctrl Pts',(1.54083026051303,0.888963444542273,
-8.7928045843712));
#146297=CARTESIAN_POINT('Ctrl Pts',(1.53248988148326,0.769956469556595,
-8.73236524355606));
#146298=CARTESIAN_POINT('Ctrl Pts',(1.51451479838375,0.424051722949861,
-8.60213239572781));
#146299=CARTESIAN_POINT('Ctrl Pts',(1.50903778348876,0.188791058808314,
-8.56247833489648));
#146300=CARTESIAN_POINT('Ctrl Pts',(1.51073127385162,-0.283921315909679,
-8.5747426488163));
#146301=CARTESIAN_POINT('Ctrl Pts',(1.51788910595866,-0.516830885584297,
-8.62656987157201));
#146302=CARTESIAN_POINT('Ctrl Pts',(1.53655937659348,-0.826237684472212,
-8.76185716159183));
#146303=CARTESIAN_POINT('Ctrl Pts',(1.54322019145936,-0.915473689807618,
-8.81013121996665));
#146304=CARTESIAN_POINT('Ctrl Pts',(1.55084034140624,-0.99999999980828,
-8.86537614723733));
#146305=CARTESIAN_POINT('Origin',(1.11022302462516E-15,0.999999999999982,
2.22044604925031E-15));
#146306=CARTESIAN_POINT('Origin',(1.11022302462516E-15,-1.77635683940025E-14,
2.22044604925031E-15));
#146307=CARTESIAN_POINT('',(0.863564213,-1.00000000000002,-8.958474025));
#146308=CARTESIAN_POINT('',(0.863564213,0.999999999999982,-8.958474025));
#146309=CARTESIAN_POINT('Ctrl Pts',(0.863564213524502,-1.00000000018892,
-8.95847402464141));
#146310=CARTESIAN_POINT('Ctrl Pts',(0.853906850043781,-0.888963444813415,
-8.88585468284159));
#146311=CARTESIAN_POINT('Ctrl Pts',(0.845867574068788,-0.769956469697459,
-8.82537455475955));
#146312=CARTESIAN_POINT('Ctrl Pts',(0.828548150532186,-0.424051722948203,
-8.69505289175402));
#146313=CARTESIAN_POINT('Ctrl Pts',(0.823278348211899,-0.188791058808255,
-8.65537076207234));
#146314=CARTESIAN_POINT('Ctrl Pts',(0.824908645788199,0.283921315907445,
-8.6676436360364));
#146315=CARTESIAN_POINT('Ctrl Pts',(0.831796712342162,0.516830885581175,
-8.71950740101901));
#146316=CARTESIAN_POINT('Ctrl Pts',(0.849790668772453,0.826237684609472,
-8.8548863040852));
#146317=CARTESIAN_POINT('Ctrl Pts',(0.856212568854875,0.915473690074354,
-8.90319272575271));
#146318=CARTESIAN_POINT('Ctrl Pts',(0.863564213524502,1.00000000018889,
-8.95847402464141));
#146319=CARTESIAN_POINT('',(0.749910923000001,-1.00000000000002,-8.968703006));
#146320=CARTESIAN_POINT('Origin',(1.11022302462516E-15,-1.00000000000002,
2.22044604925031E-15));
#146321=CARTESIAN_POINT('',(0.749910923000001,0.999999999999982,-8.968703006));
#146322=CARTESIAN_POINT('Ctrl Pts',(0.749910923421742,1.0000000000954,-8.96870300583525));
#146323=CARTESIAN_POINT('Ctrl Pts',(0.746446404937194,0.888963444745312,
-8.89552629792414));
#146324=CARTESIAN_POINT('Ctrl Pts',(0.743557342583251,0.76995646965958,
-8.83458264224673));
#146325=CARTESIAN_POINT('Ctrl Pts',(0.737328604408766,0.424051722945632,
-8.70326279950605));
#146326=CARTESIAN_POINT('Ctrl Pts',(0.735428200989169,0.188791058807976,
-8.66327741843499));
#146327=CARTESIAN_POINT('Ctrl Pts',(0.736015509228912,-0.283921315904421,
-8.67564416313782));
#146328=CARTESIAN_POINT('Ctrl Pts',(0.738498769557774,-0.516830885576862,
-8.72790436785553));
#146329=CARTESIAN_POINT('Ctrl Pts',(0.744966819940245,-0.826237684571764,
-8.86432062122607));
#146330=CARTESIAN_POINT('Ctrl Pts',(0.747273567077169,-0.91547369000699,
-8.91299741334236));
#146331=CARTESIAN_POINT('Ctrl Pts',(0.749910923421742,-1.00000000009543,
-8.96870300583525));
#146332=CARTESIAN_POINT('Origin',(1.11022302462516E-15,0.999999999999982,
2.22044604925031E-15));
#146333=CARTESIAN_POINT('Origin',(1.11022302462516E-15,-1.77635683940025E-14,
2.22044604925031E-15));
#146334=CARTESIAN_POINT('',(0.057056338,-1.00000000000002,-8.999819141));
#146335=CARTESIAN_POINT('',(0.057056338,0.999999999999982,-8.999819141));
#146336=CARTESIAN_POINT('Ctrl Pts',(0.0570563383389186,-0.999999999933197,
-8.99981914108697));
#146337=CARTESIAN_POINT('Ctrl Pts',(0.0539474002202264,-0.888963444633974,
-8.92662646409639));
#146338=CARTESIAN_POINT('Ctrl Pts',(0.0513618849266559,-0.76995646960878,
-8.86566917614543));
#146339=CARTESIAN_POINT('Ctrl Pts',(0.0457941281782637,-0.424051722954681,
-8.73431964871831));
#146340=CARTESIAN_POINT('Ctrl Pts',(0.0441026192351812,-0.188791058808771,
-8.69432488618503));
#146341=CARTESIAN_POINT('Ctrl Pts',(0.0446262217656046,0.283921315915514,
-8.70669449191622));
#146342=CARTESIAN_POINT('Ctrl Pts',(0.0468375269099042,0.516830885592592,
-8.75896691015616));
#146343=CARTESIAN_POINT('Ctrl Pts',(0.0526237735737155,0.82623768452456,
-8.89541378333879));
#146344=CARTESIAN_POINT('Ctrl Pts',(0.054689666691092,0.915473689898555,
-8.94410139218079));
#146345=CARTESIAN_POINT('Ctrl Pts',(0.0570563383389185,0.999999999933161,
-8.99981914108697));
#146346=CARTESIAN_POINT('',(-0.0570563369999999,-1.00000000000002,-8.999819141));
#146347=CARTESIAN_POINT('Origin',(1.11022302462516E-15,-1.00000000000002,
2.22044604925031E-15));
#146348=CARTESIAN_POINT('',(-0.0570563369999999,0.999999999999982,-8.999819141));
#146349=CARTESIAN_POINT('Ctrl Pts',(-0.0570563367490442,0.999999999940042,
-8.99981914110159));
#146350=CARTESIAN_POINT('Ctrl Pts',(-0.0539473986136921,0.888963444636815,
-8.92662646410728));
#146351=CARTESIAN_POINT('Ctrl Pts',(-0.0513618833063578,0.769956469606837,
-8.86566917615349));
#146352=CARTESIAN_POINT('Ctrl Pts',(-0.0457941265286543,0.424051722950587,
-8.73431964872652));
#146353=CARTESIAN_POINT('Ctrl Pts',(-0.0441026175767645,0.188791058808359,
-8.69432488619385));
#146354=CARTESIAN_POINT('Ctrl Pts',(-0.0446262201098946,-0.283921315910611,
-8.70669449192419));
#146355=CARTESIAN_POINT('Ctrl Pts',(-0.0468375252657083,-0.51683088558561,
-8.75896691016323));
#146356=CARTESIAN_POINT('Ctrl Pts',(-0.0526237719600614,-0.826237684521612,
-8.89541378334643));
#146357=CARTESIAN_POINT('Ctrl Pts',(-0.0546896650884917,-0.91547368990086,
-8.94410139219154));
#146358=CARTESIAN_POINT('Ctrl Pts',(-0.0570563367490442,-0.999999999940079,
-8.99981914110159));
#146359=CARTESIAN_POINT('Origin',(1.11022302462516E-15,0.999999999999982,
2.22044604925031E-15));
#146360=CARTESIAN_POINT('Origin',(1.11022302462516E-15,-1.77635683940025E-14,
2.22044604925031E-15));
#146361=CARTESIAN_POINT('',(-0.749910922999999,-1.00000000000002,-8.968703006));
#146362=CARTESIAN_POINT('',(-0.749910922999999,0.999999999999982,-8.968703006));
#146363=CARTESIAN_POINT('Ctrl Pts',(-0.749910923031043,-1.00000000008893,
-8.96870300586362));
#146364=CARTESIAN_POINT('Ctrl Pts',(-0.746446404541414,-0.888963444741282,
-8.89552629795534));
#146365=CARTESIAN_POINT('Ctrl Pts',(-0.743557342183263,-0.769956469658455,
-8.83458264228013));
#146366=CARTESIAN_POINT('Ctrl Pts',(-0.737328603999571,-0.424051722946837,
-8.70326279954085));
#146367=CARTESIAN_POINT('Ctrl Pts',(-0.735428200577178,-0.188791058808127,
-8.66327741846985));
#146368=CARTESIAN_POINT('Ctrl Pts',(-0.736015508817798,0.28392131590579,
-8.67564416317284));
#146369=CARTESIAN_POINT('Ctrl Pts',(-0.738498769150314,0.516830885578821,
-8.72790436789049));
#146370=CARTESIAN_POINT('Ctrl Pts',(-0.744966819542354,0.826237684570914,
-8.86432062125932));
#146371=CARTESIAN_POINT('Ctrl Pts',(-0.747273566682627,0.915473690003112,
-8.91299741337342));
#146372=CARTESIAN_POINT('Ctrl Pts',(-0.749910923031043,1.00000000008889,
-8.96870300586362));
#146373=CARTESIAN_POINT('',(-0.863564211999999,-1.00000000000002,-8.958474025));
#146374=CARTESIAN_POINT('Origin',(1.11022302462516E-15,-1.00000000000002,
2.22044604925031E-15));
#146375=CARTESIAN_POINT('',(-0.863564212999999,0.999999999999982,-8.958474025));
#146376=CARTESIAN_POINT('Ctrl Pts',(-0.863564212376334,1.00000000020806,
-8.95847402476479));
#146377=CARTESIAN_POINT('Ctrl Pts',(-0.85390684889901,0.888963444826714,
-8.88585468295841));
#146378=CARTESIAN_POINT('Ctrl Pts',(-0.845867572926913,0.76995646970382,
-8.82537455487132));
#146379=CARTESIAN_POINT('Ctrl Pts',(-0.82854814939751,0.424051722947429,
-8.69505289186206));
#146380=CARTESIAN_POINT('Ctrl Pts',(-0.823278347079534,0.188791058808129,
-8.65537076218012));
#146381=CARTESIAN_POINT('Ctrl Pts',(-0.824908644655102,-0.283921315906636,
-8.66764363614415));
#146382=CARTESIAN_POINT('Ctrl Pts',(-0.831796711206042,-0.516830885579999,
-8.7195074011271));
#146383=CARTESIAN_POINT('Ctrl Pts',(-0.849790667627615,-0.826237684593336,
-8.8548863041878));
#146384=CARTESIAN_POINT('Ctrl Pts',(-0.856212567706076,-0.915473690044782,
-8.90319272584691));
#146385=CARTESIAN_POINT('Ctrl Pts',(-0.863564212371063,-1.00000000014749,
-8.95847402472516));
#146386=CARTESIAN_POINT('Origin',(1.11022302462516E-15,0.999999999999982,
2.22044604925031E-15));
#146387=CARTESIAN_POINT('Origin',(1.11022302462516E-15,-1.77635683940025E-14,
2.22044604925031E-15));
#146388=CARTESIAN_POINT('',(-1.550840341,-1.00000000000002,-8.865376147));
#146389=CARTESIAN_POINT('',(-1.550840341,0.999999999999982,-8.865376147));
#146390=CARTESIAN_POINT('Ctrl Pts',(-1.55084034103818,-0.999999999802089,
-8.86537614729757));
#146391=CARTESIAN_POINT('Ctrl Pts',(-1.54083026013964,-0.888963444538492,
-8.79280458443473));
#146392=CARTESIAN_POINT('Ctrl Pts',(-1.53248988110543,-0.769956469555648,
-8.73236524362217));
#146393=CARTESIAN_POINT('Ctrl Pts',(-1.51451479799595,-0.424051722951105,
-8.60213239579622));
#146394=CARTESIAN_POINT('Ctrl Pts',(-1.50903778309791,-0.188791058808463,
-8.56247833496524));
#146395=CARTESIAN_POINT('Ctrl Pts',(-1.51073127346174,0.283921315911108,
-8.57474264888515));
#146396=CARTESIAN_POINT('Ctrl Pts',(-1.51788910557278,0.516830885586346,
-8.62656987164042));
#146397=CARTESIAN_POINT('Ctrl Pts',(-1.53655937621794,0.826237684471543,
-8.76185716165758));
#146398=CARTESIAN_POINT('Ctrl Pts',(-1.54322019108732,0.915473689803992,
-8.81013122002992));
#146399=CARTESIAN_POINT('Ctrl Pts',(-1.55084034103818,0.999999999802054,
-8.86537614729757));
#146400=CARTESIAN_POINT('',(-1.663119178,-1.00000000000002,-8.845000543));
#146401=CARTESIAN_POINT('Origin',(1.11022302462516E-15,-1.00000000000002,
2.22044604925031E-15));
#146402=CARTESIAN_POINT('',(-1.663119178,0.999999999999982,-8.845000543));
#146403=CARTESIAN_POINT('Ctrl Pts',(-1.66311917779156,1.00000000018363,
-8.84500054276169));
#146404=CARTESIAN_POINT('Ctrl Pts',(-1.64699114441794,0.888963444810215,
-8.77353922446984));
#146405=CARTESIAN_POINT('Ctrl Pts',(-1.63356283533152,0.769956469696761,
-8.71402320674444));
#146406=CARTESIAN_POINT('Ctrl Pts',(-1.60463119091762,0.424051722949323,
-8.58577868159241));
#146407=CARTESIAN_POINT('Ctrl Pts',(-1.5958255245984,0.188791058808294,
-8.54672868193495));
#146408=CARTESIAN_POINT('Ctrl Pts',(-1.59854939101432,-0.283921315908962,
-8.55880601016923));
#146409=CARTESIAN_POINT('Ctrl Pts',(-1.61005876027881,-0.516830885583298,
-8.60984354535825));
#146410=CARTESIAN_POINT('Ctrl Pts',(-1.64011554961833,-0.826237684609204,
-8.74306448694674));
#146411=CARTESIAN_POINT('Ctrl Pts',(-1.65084175126428,-0.915473690071452,
-8.79060078647737));
#146412=CARTESIAN_POINT('Ctrl Pts',(-1.66311917779156,-1.00000000018366,
-8.84500054276169));
#146413=CARTESIAN_POINT('Origin',(1.11022302462516E-15,0.999999999999982,
2.22044604925031E-15));
#146414=CARTESIAN_POINT('Origin',(1.11022302462516E-15,-1.77635683940025E-14,
2.22044604925031E-15));
#146415=CARTESIAN_POINT('',(-2.339283305,-1.00000000000002,-8.690670493));
#146416=CARTESIAN_POINT('',(-2.339283305,0.999999999999982,-8.690670493));
#146417=CARTESIAN_POINT('Ctrl Pts',(-2.33928330447186,-0.999999999994548,
-8.6906704931304));
#146418=CARTESIAN_POINT('Ctrl Pts',(-2.32280825646114,-0.888963444676296,
-8.61928837872337));
#146419=CARTESIAN_POINT('Ctrl Pts',(-2.30908371258921,-0.769956469628456,
-8.55983997469919));
#146420=CARTESIAN_POINT('Ctrl Pts',(-2.27950700939569,-0.424051722951681,
-8.43174268003197));
#146421=CARTESIAN_POINT('Ctrl Pts',(-2.27049748074064,-0.188791058808523,
-8.39273921062221));
#146422=CARTESIAN_POINT('Ctrl Pts',(-2.27328351823432,0.2839213159118,-8.40480234871414));
#146423=CARTESIAN_POINT('Ctrl Pts',(-2.2850582914487,0.516830885587333,
-8.45577930718373));
#146424=CARTESIAN_POINT('Ctrl Pts',(-2.31578046026309,0.82623768454295,
-8.58884838021716));
#146425=CARTESIAN_POINT('Ctrl Pts',(-2.32674171389091,0.915473689939805,
-8.63633103062244));
#146426=CARTESIAN_POINT('Ctrl Pts',(-2.33928330447186,0.999999999994512,
-8.6906704931304));
#146427=CARTESIAN_POINT('',(-2.449283685,-1.00000000000002,-8.660312317));
#146428=CARTESIAN_POINT('Origin',(1.11022302462516E-15,-1.00000000000002,
2.22044604925031E-15));
#146429=CARTESIAN_POINT('',(-2.449283685,0.999999999999982,-8.660312317));
#146430=CARTESIAN_POINT('Ctrl Pts',(-2.44928368526842,0.999999999964309,
-8.66031231697031));
#146431=CARTESIAN_POINT('Ctrl Pts',(-2.42681483546961,0.88896344465514,
-8.59058438675928));
#146432=CARTESIAN_POINT('Ctrl Pts',(-2.40810561014116,0.769956469618107,
-8.53251166741322));
#146433=CARTESIAN_POINT('Ctrl Pts',(-2.36779468545961,0.424051722952562,
-8.40737682964596));
#146434=CARTESIAN_POINT('Ctrl Pts',(-2.35552405319222,0.188791058808562,
-8.36927336764646));
#146435=CARTESIAN_POINT('Ctrl Pts',(-2.35931955747613,-0.283921315912972,
-8.38105791060647));
#146436=CARTESIAN_POINT('Ctrl Pts',(-2.37535756277304,-0.516830885588973,
-8.43085829178138));
#146437=CARTESIAN_POINT('Ctrl Pts',(-2.41723518540491,-0.826237684533162,
-8.56084865517789));
#146438=CARTESIAN_POINT('Ctrl Pts',(-2.43217932752638,-0.915473689919173,
-8.60723209819538));
#146439=CARTESIAN_POINT('Ctrl Pts',(-2.44928368526842,-0.999999999964344,
-8.66031231697031));
#146440=CARTESIAN_POINT('Origin',(1.11022302462516E-15,0.999999999999982,
2.22044604925031E-15));
#146441=CARTESIAN_POINT('Origin',(1.11022302462516E-15,-1.77635683940025E-14,
2.22044604925031E-15));
#146442=CARTESIAN_POINT('',(-3.108891735,-1.00000000000002,-8.44599267));
#146443=CARTESIAN_POINT('',(-3.108891735,0.999999999999982,-8.44599267));
#146444=CARTESIAN_POINT('Ctrl Pts',(-3.10889173544937,-1.0000000000809,
-8.44599266972378));
#146445=CARTESIAN_POINT('Ctrl Pts',(-3.08608436775725,-0.888963444735185,
-8.37637473060366));
#146446=CARTESIAN_POINT('Ctrl Pts',(-3.06708616103101,-0.769956469654648,
-8.31839590697488));
#146447=CARTESIAN_POINT('Ctrl Pts',(-3.02614597203477,-0.424051722946105,
-8.19346552955976));
#146448=CARTESIAN_POINT('Ctrl Pts',(-3.01367646906759,-0.188791058808043,
-8.15542668456797));
#146449=CARTESIAN_POINT('Ctrl Pts',(-3.01753262214961,0.283921315904936,
-8.16719152153766));
#146450=CARTESIAN_POINT('Ctrl Pts',(-3.03382953289371,0.516830885577599,
-8.21690777923272));
#146451=CARTESIAN_POINT('Ctrl Pts',(-3.07635624297832,0.826237684567004,
-8.34668724135259));
#146452=CARTESIAN_POINT('Ctrl Pts',(-3.0915296817749,0.915473689997013,
-8.39299618139483));
#146453=CARTESIAN_POINT('Ctrl Pts',(-3.10889173544937,1.00000000008087,
-8.44599266972378));
#146454=CARTESIAN_POINT('',(-3.215728,-1.00000000000002,-8.405896349));
#146455=CARTESIAN_POINT('Origin',(1.11022302462516E-15,-1.00000000000002,
2.22044604925031E-15));
#146456=CARTESIAN_POINT('',(-3.215728,0.999999999999982,-8.405896349));
#146457=CARTESIAN_POINT('Ctrl Pts',(-3.21572799949971,1.00000000004184,
-8.40589634914347));
#146458=CARTESIAN_POINT('Ctrl Pts',(-3.1870992391518,0.888963444706609,
-8.33846321524215));
#146459=CARTESIAN_POINT('Ctrl Pts',(-3.16325973318893,0.769956469638536,
-8.28230136161672));
#146460=CARTESIAN_POINT('Ctrl Pts',(-3.11189408797419,0.424051722944788,
-8.1612837233719));
#146461=CARTESIAN_POINT('Ctrl Pts',(-3.09625728563935,0.188791058807923,
-8.12443358571553));
#146462=CARTESIAN_POINT('Ctrl Pts',(-3.10109386863279,-0.283921315903343,
-8.13583046118458));
#146463=CARTESIAN_POINT('Ctrl Pts',(-3.12153138141973,-0.516830885575342,
-8.18399272494027));
#146464=CARTESIAN_POINT('Ctrl Pts',(-3.17489266348559,-0.826237684550909,
-8.30970590417526));
#146465=CARTESIAN_POINT('Ctrl Pts',(-3.19393442470021,-0.915473689968737,
-8.35456303852214));
#146466=CARTESIAN_POINT('Ctrl Pts',(-3.21572799949971,-1.00000000004188,
-8.40589634914347));
#146467=CARTESIAN_POINT('Origin',(1.11022302462516E-15,0.999999999999982,
2.22044604925031E-15));
#146468=CARTESIAN_POINT('Origin',(1.11022302462516E-15,-1.77635683940025E-14,
2.22044604925031E-15));
#146469=CARTESIAN_POINT('',(-3.85346919675118,-0.999999999914645,-8.13331268017501));
#146470=CARTESIAN_POINT('',(-3.853469196,0.999999999999982,-8.13331268));
#146471=CARTESIAN_POINT('Ctrl Pts',(-3.85346919578197,-1.00000000005209,
-8.13331268036528));
#146472=CARTESIAN_POINT('Ctrl Pts',(-3.82451313984361,-0.888963444719943,
-8.06601943931758));
#146473=CARTESIAN_POINT('Ctrl Pts',(-3.8003942325866,-0.769956469655612,
-8.00997700754015));
#146474=CARTESIAN_POINT('Ctrl Pts',(-3.74842018395872,-0.424051722956698,
-7.889219413393));
#146475=CARTESIAN_POINT('Ctrl Pts',(-3.73259110373581,-0.188791058808942,
-7.85245145924943));
#146476=CARTESIAN_POINT('Ctrl Pts',(-3.73748632494522,0.283921315917998,
-7.86382327154454));
#146477=CARTESIAN_POINT('Ctrl Pts',(-3.75817416014108,0.516830885596111,
-7.9118785423691));
#146478=CARTESIAN_POINT('Ctrl Pts',(-3.81216301158527,0.826237684515586,
-8.03732348555132));
#146479=CARTESIAN_POINT('Ctrl Pts',(-3.83142646798091,0.915473689877324,
-8.08208586278962));
#146480=CARTESIAN_POINT('Ctrl Pts',(-3.85346919574261,0.999999999901152,
-8.13331268027382));
#146481=CARTESIAN_POINT('',(-3.956281164,-1.00000000000002,-8.083801046));
#146482=CARTESIAN_POINT('Origin',(1.11022302462516E-15,-1.00000000000002,
2.22044604925031E-15));
#146483=CARTESIAN_POINT('',(-3.956281164,0.999999999999982,-8.083801046));
#146484=CARTESIAN_POINT('Ctrl Pts',(-3.95628116427791,1.00000000002303,
-8.08380104581171));
#146485=CARTESIAN_POINT('Ctrl Pts',(-3.92172299544629,0.888963444698272,
-8.01920564015371));
#146486=CARTESIAN_POINT('Ctrl Pts',(-3.89294515063276,0.769956469642722,
-7.96540683446067));
#146487=CARTESIAN_POINT('Ctrl Pts',(-3.83093835105285,0.424051722954888,
-7.84948075853399));
#146488=CARTESIAN_POINT('Ctrl Pts',(-3.8120612770459,0.18879105880875,-7.81418064083539));
#146489=CARTESIAN_POINT('Ctrl Pts',(-3.81789999740993,-0.283921315915858,
-7.82509808788435));
#146490=CARTESIAN_POINT('Ctrl Pts',(-3.84257246677633,-0.516830885593061,
-7.87123446002671));
#146491=CARTESIAN_POINT('Ctrl Pts',(-3.9069877744043,-0.826237684557927,
-7.99165828656834));
#146492=CARTESIAN_POINT('Ctrl Pts',(-3.92997384156548,-0.915473689962003,
-8.03462794897708));
#146493=CARTESIAN_POINT('Ctrl Pts',(-3.95628116427791,-1.00000000002306,
-8.08380104581171));
#146494=CARTESIAN_POINT('Origin',(1.11022302462516E-15,0.999999999999982,
2.22044604925031E-15));
#146495=CARTESIAN_POINT('Origin',(1.11022302462516E-15,-1.77635683940025E-14,
2.22044604925031E-15));
#146496=CARTESIAN_POINT('',(-4.56702079,-1.00000000000002,-7.755148038));
#146497=CARTESIAN_POINT('',(-4.567020791,0.999999999999982,-7.755148038));
#146498=CARTESIAN_POINT('Ctrl Pts',(-4.5670207907231,-0.999999999723034,
-7.75514803808598));
#146499=CARTESIAN_POINT('Ctrl Pts',(-4.53214918384362,-0.888963444478476,
-7.69072130072636));
#146500=CARTESIAN_POINT('Ctrl Pts',(-4.5031037674526,-0.769956469518228,
-7.63706648150941));
#146501=CARTESIAN_POINT('Ctrl Pts',(-4.44051432392658,-0.424051722944118,
-7.52145393970776));
#146502=CARTESIAN_POINT('Ctrl Pts',(-4.42145311296568,-0.188791058807883,
-7.48625291033001));
#146503=CARTESIAN_POINT('Ctrl Pts',(-4.42734798883601,0.283921315902463,
-7.49714013881019));
#146504=CARTESIAN_POINT('Ctrl Pts',(-4.45226018210561,0.516830885574101,
-7.54314751001829));
#146505=CARTESIAN_POINT('Ctrl Pts',(-4.5172764881937,0.82623768451322,-7.66324792548531));
#146506=CARTESIAN_POINT('Ctrl Pts',(-4.54047486409895,0.915473689897858,
-7.70610333967294));
#146507=CARTESIAN_POINT('Ctrl Pts',(-4.56702079079182,0.999999999941809,
-7.75514803821294));
#146508=CARTESIAN_POINT('',(-4.664980679,-1.00000000000002,-7.69661973));
#146509=CARTESIAN_POINT('Origin',(1.11022302462516E-15,-1.00000000000002,
2.22044604925031E-15));
#146510=CARTESIAN_POINT('',(-4.664980678,0.999999999999982,-7.69661973));
#146511=CARTESIAN_POINT('Ctrl Pts',(-4.66498067874573,0.999999999872924,
-7.69661972974073));
#146512=CARTESIAN_POINT('Ctrl Pts',(-4.62477134343723,0.888963444590632,
-7.63538213660728));
#146513=CARTESIAN_POINT('Ctrl Pts',(-4.59128686201658,0.769956469585573,
-7.58437953524182));
#146514=CARTESIAN_POINT('Ctrl Pts',(-4.51913815025123,0.424051722954113,
-7.47447839030291));
#146515=CARTESIAN_POINT('Ctrl Pts',(-4.49717279163596,0.188791058808665,
-7.44101250837074));
#146516=CARTESIAN_POINT('Ctrl Pts',(-4.50396663943793,-0.283921315914944,
-7.45136262612836));
#146517=CARTESIAN_POINT('Ctrl Pts',(-4.53267541721535,-0.516830885591754,
-7.49510164369407));
#146518=CARTESIAN_POINT('Ctrl Pts',(-4.60762611636159,-0.826237684594402,
-7.60926653566084));
#146519=CARTESIAN_POINT('Ctrl Pts',(-4.63437141923369,-0.915473690033446,
-7.65000275968309));
#146520=CARTESIAN_POINT('Ctrl Pts',(-4.66498067883709,-1.00000000012526,
-7.69661972987988));
#146521=CARTESIAN_POINT('Origin',(1.11022302462516E-15,0.999999999999982,
2.22044604925031E-15));
#146522=CARTESIAN_POINT('Origin',(1.11022302462516E-15,-1.77635683940025E-14,
2.22044604925031E-15));
#146523=CARTESIAN_POINT('',(-5.243801418,-1.00000000000002,-7.314543505));
#146524=CARTESIAN_POINT('',(-5.243801418,0.999999999999982,-7.314543505));
#146525=CARTESIAN_POINT('Ctrl Pts',(-5.2438014182955,-0.999999999983744,
-7.31454350483351));
#146526=CARTESIAN_POINT('Ctrl Pts',(-5.20329502600418,-0.888963444664369,
-7.25350199725071));
#146527=CARTESIAN_POINT('Ctrl Pts',(-5.16955695697835,-0.769956469615146,
-7.20266678756193));
#146528=CARTESIAN_POINT('Ctrl Pts',(-5.09685605179224,-0.424051722943349,
-7.09313014228908));
#146529=CARTESIAN_POINT('Ctrl Pts',(-5.07471617971955,-0.188791058807812,
-7.0597794556822));
#146530=CARTESIAN_POINT('Ctrl Pts',(-5.08156324818856,0.283921315901536,
-7.0700944427827));
#146531=CARTESIAN_POINT('Ctrl Pts',(-5.11049922124789,0.516830885572785,
-7.11368349005474));
#146532=CARTESIAN_POINT('Ctrl Pts',(-5.18601950903758,0.826237684527553,
-7.22747239982518));
#146533=CARTESIAN_POINT('Ctrl Pts',(-5.21296602481403,0.91547368992686,
-7.26807580434118));
#146534=CARTESIAN_POINT('Ctrl Pts',(-5.2438014182955,0.999999999983708,
-7.31454350483351));
#146535=CARTESIAN_POINT('',(-5.336120511,-1.00000000000002,-7.247469758));
#146536=CARTESIAN_POINT('Origin',(1.11022302462516E-15,-1.00000000000002,
2.22044604925031E-15));
#146537=CARTESIAN_POINT('',(-5.336120511,0.999999999999982,-7.247469758));
#146538=CARTESIAN_POINT('Ctrl Pts',(-5.3361205105636,1.00000000006483,-7.24746975822081));
#146539=CARTESIAN_POINT('Ctrl Pts',(-5.29058375060566,0.888963444722998,
-7.19008302665036));
#146540=CARTESIAN_POINT('Ctrl Pts',(-5.25266222985656,0.769956469647075,
-7.1422872725303));
#146541=CARTESIAN_POINT('Ctrl Pts',(-5.17095250481387,0.424051722944707,
-7.03929591799513));
#146542=CARTESIAN_POINT('Ctrl Pts',(-5.14607571372182,0.1887910588079,-7.0079337194511));
#146543=CARTESIAN_POINT('Ctrl Pts',(-5.1537699888994,-0.283921315903279,
-7.01763317484824));
#146544=CARTESIAN_POINT('Ctrl Pts',(-5.18628392891646,-0.516830885575241,
-7.05862267696227));
#146545=CARTESIAN_POINT('Ctrl Pts',(-5.27116656068067,-0.826237684559263,
-7.16560944569037));
#146546=CARTESIAN_POINT('Ctrl Pts',(-5.30145576182033,-0.915473689984878,
-7.20378424715405));
#146547=CARTESIAN_POINT('Ctrl Pts',(-5.3361205105636,-1.00000000006487,
-7.24746975822081));
#146548=CARTESIAN_POINT('Origin',(1.11022302462516E-15,0.999999999999982,
2.22044604925031E-15));
#146549=CARTESIAN_POINT('Origin',(1.11022302462516E-15,-1.77635683940025E-14,
2.22044604925031E-15));
#146550=CARTESIAN_POINT('',(-5.87836204,-1.00000000000002,-6.815046568));
#146551=CARTESIAN_POINT('',(-5.878362039,0.999999999999982,-6.815046569));
#146552=CARTESIAN_POINT('Ctrl Pts',(-5.8783620393509,-0.999999999947016,
-6.81504656862317));
#146553=CARTESIAN_POINT('Ctrl Pts',(-5.83254699529058,-0.888963444643322,
-6.75788176127013));
#146554=CARTESIAN_POINT('Ctrl Pts',(-5.79438791271225,-0.769956469612807,
-6.71027545642628));
#146555=CARTESIAN_POINT('Ctrl Pts',(-5.71216089072527,-0.424051722953643,
-6.60769663246045));
#146556=CARTESIAN_POINT('Ctrl Pts',(-5.6871206147411,-0.188791058808675,
-6.57646480876682));
#146557=CARTESIAN_POINT('Ctrl Pts',(-5.69486474725043,0.283921315914249,
-6.58612450427073));
#146558=CARTESIAN_POINT('Ctrl Pts',(-5.72759152469995,0.516830885590793,
-6.62694427419722));
#146559=CARTESIAN_POINT('Ctrl Pts',(-5.81300774934533,0.826237684554357,
-6.73350551678999));
#146560=CARTESIAN_POINT('Ctrl Pts',(-5.84348544752745,0.915473689957745,
-6.77152999685925));
#146561=CARTESIAN_POINT('Ctrl Pts',(-5.87836203938029,1.0000000000182,-6.81504656865983));
#146562=CARTESIAN_POINT('',(-5.964297039,-1.00000000000002,-6.739967421));
#146563=CARTESIAN_POINT('Origin',(1.11022302462516E-15,-1.00000000000002,
2.22044604925031E-15));
#146564=CARTESIAN_POINT('',(-5.964297039,0.999999999999982,-6.739967421));
#146565=CARTESIAN_POINT('Ctrl Pts',(-5.96429703907415,1.00000000016684,
-6.73996742058037));
#146566=CARTESIAN_POINT('Ctrl Pts',(-5.91379948977288,0.888963444798608,
-6.68689359476871));
#146567=CARTESIAN_POINT('Ctrl Pts',(-5.87174625155671,0.769956469691324,
-6.64268951118085));
#146568=CARTESIAN_POINT('Ctrl Pts',(-5.78113339203643,0.424051722950086,
-6.54743717279022));
#146569=CARTESIAN_POINT('Ctrl Pts',(-5.75354546180194,0.18879105880834,
-6.51843116758519));
#146570=CARTESIAN_POINT('Ctrl Pts',(-5.76207821456473,-0.28392131590995,
-6.52740186632182));
#146571=CARTESIAN_POINT('Ctrl Pts',(-5.79813553364252,-0.516830885584689,
-6.56531182965558));
#146572=CARTESIAN_POINT('Ctrl Pts',(-5.8922666728607,-0.826237684604123,
-6.66425908071305));
#146573=CARTESIAN_POINT('Ctrl Pts',(-5.92585590139914,-0.91547369006014,
-6.69956509862226));
#146574=CARTESIAN_POINT('Ctrl Pts',(-5.96429703907415,-1.00000000016687,
-6.73996742058037));
#146575=CARTESIAN_POINT('Origin',(1.11022302462516E-15,0.999999999999982,
2.22044604925031E-15));
#146576=CARTESIAN_POINT('Origin',(1.11022302462516E-15,-1.77635683940025E-14,
2.22044604925031E-15));
#146577=CARTESIAN_POINT('',(-6.465593547,-1.00000000000002,-6.260678884));
#146578=CARTESIAN_POINT('',(-6.465593547,0.999999999999982,-6.260678883));
#146579=CARTESIAN_POINT('Ctrl Pts',(-6.465593547415,-1.00000000013442,-6.26067888331879));
#146580=CARTESIAN_POINT('Ctrl Pts',(-6.41483872740882,-0.888963444774572,
-6.20785103349866));
#146581=CARTESIAN_POINT('Ctrl Pts',(-6.37256586579951,-0.769956469677245,
-6.16385693138393));
#146582=CARTESIAN_POINT('Ctrl Pts',(-6.2814747707594,-0.424051722948395,
-6.06906183297416));
#146583=CARTESIAN_POINT('Ctrl Pts',(-6.25373570048456,-0.18879105880825,
-6.04020033244393));
#146584=CARTESIAN_POINT('Ctrl Pts',(-6.26231454581811,0.283921315907737,
-6.04912696217015));
#146585=CARTESIAN_POINT('Ctrl Pts',(-6.29856863083365,0.516830885581577,
-6.08684879800449));
#146586=CARTESIAN_POINT('Ctrl Pts',(-6.39319307094973,0.826237684468098,
-6.18532440503001));
#146587=CARTESIAN_POINT('Ctrl Pts',(-6.42695656294875,0.915473689802836,
-6.22046380990041));
#146588=CARTESIAN_POINT('Ctrl Pts',(-6.46559354726348,0.999999999802907,
-6.26067888316109));
#146589=CARTESIAN_POINT('',(-6.544452554,-1.00000000000002,-6.178198829));
#146590=CARTESIAN_POINT('Origin',(1.11022302462516E-15,-1.00000000000002,
2.22044604925031E-15));
#146591=CARTESIAN_POINT('',(-6.544452554,0.999999999999982,-6.178198829));
#146592=CARTESIAN_POINT('Ctrl Pts',(-6.54445255390455,1.0000000000868,-6.17819882890926));
#146593=CARTESIAN_POINT('Ctrl Pts',(-6.48940079184017,0.888963444741018,
-6.12986522815414));
#146594=CARTESIAN_POINT('Ctrl Pts',(-6.44355442410624,0.769956469660418,
-6.0896087204346));
#146595=CARTESIAN_POINT('Ctrl Pts',(-6.34476799154022,0.424051722949282,
-6.00286231406975));
#146596=CARTESIAN_POINT('Ctrl Pts',(-6.31469104394089,0.188791058808275,
-5.97644604151514));
#146597=CARTESIAN_POINT('Ctrl Pts',(-6.32399357358486,-0.283921315908946,
-5.98461575679496));
#146598=CARTESIAN_POINT('Ctrl Pts',(-6.36330395941132,-0.516830885583268,
-6.01914095259761));
#146599=CARTESIAN_POINT('Ctrl Pts',(-6.46592571753245,-0.82623768457364,
-6.10925202083548));
#146600=CARTESIAN_POINT('Ctrl Pts',(-6.50254453274514,-0.915473690003293,
-6.1414049918512));
#146601=CARTESIAN_POINT('Ctrl Pts',(-6.54445255390455,-1.00000000008684,
-6.17819882890926));
#146602=CARTESIAN_POINT('Origin',(1.11022302462516E-15,0.999999999999982,
2.22044604925031E-15));
#146603=CARTESIAN_POINT('Origin',(1.11022302462516E-15,-1.77635683940025E-14,
2.22044604925031E-15));
#146604=CARTESIAN_POINT('',(-7.000767897,-1.00000000000002,-5.655903894));
#146605=CARTESIAN_POINT('',(-7.000767897,0.999999999999982,-5.655903894));
#146606=CARTESIAN_POINT('Ctrl Pts',(-7.00076789655177,-1.00000000017299,
-5.65590389411597));
#146607=CARTESIAN_POINT('Ctrl Pts',(-6.94548194857316,-0.888963444802471,
-5.60783834066879));
#146608=CARTESIAN_POINT('Ctrl Pts',(-6.89943566416173,-0.769956469692456,
-5.56781065596884));
#146609=CARTESIAN_POINT('Ctrl Pts',(-6.80021390797847,-0.42405172294906,
-5.4815625175572));
#146610=CARTESIAN_POINT('Ctrl Pts',(-6.76999938208442,-0.1887910588083,
-5.45530371603143));
#146611=CARTESIAN_POINT('Ctrl Pts',(-6.77934386842823,0.283921315908572,
-5.46342540800412));
#146612=CARTESIAN_POINT('Ctrl Pts',(-6.81883336445019,0.516830885582756,
-5.49774559569251));
#146613=CARTESIAN_POINT('Ctrl Pts',(-6.92190415979063,0.826237684604844,
-5.58734269949925));
#146614=CARTESIAN_POINT('Ctrl Pts',(-6.95868160192628,0.915473690063716,
-5.61931410742192));
#146615=CARTESIAN_POINT('Ctrl Pts',(-7.00076789655177,1.00000000017296,
-5.65590389411597));
#146616=CARTESIAN_POINT('',(-7.071915985,-1.00000000000002,-5.566687013));
#146617=CARTESIAN_POINT('Origin',(1.11022302462516E-15,-1.00000000000002,
2.22044604925031E-15));
#146618=CARTESIAN_POINT('',(-7.07191598509133,1.00000000000236,-5.56668701279559));
#146619=CARTESIAN_POINT('Ctrl Pts',(-7.07191598491097,1.00000000000174,
-5.56668701304417));
#146620=CARTESIAN_POINT('Ctrl Pts',(-7.01275325449934,0.888963444679146,
-5.52348279108474));
#146621=CARTESIAN_POINT('Ctrl Pts',(-6.96348288524122,0.769956469626119,
-5.48749798096801));
#146622=CARTESIAN_POINT('Ctrl Pts',(-6.85731824989088,0.424051722947136,
-5.40995593770057));
#146623=CARTESIAN_POINT('Ctrl Pts',(-6.82499444682085,0.188791058808089,
-5.38634208609494));
#146624=CARTESIAN_POINT('Ctrl Pts',(-6.83499185484783,-0.283921315906313,
-5.39364504017274));
#146625=CARTESIAN_POINT('Ctrl Pts',(-6.87723880331428,-0.516830885579532,
-5.42450749186227));
#146626=CARTESIAN_POINT('Ctrl Pts',(-6.98752493029364,-0.826237684546756,
-5.50505685593148));
#146627=CARTESIAN_POINT('Ctrl Pts',(-7.02687849901688,-0.915473689956015,
-5.53379790323594));
#146628=CARTESIAN_POINT('Ctrl Pts',(-7.07191598492155,-1.00000000002162,
-5.5666870130519));
#146629=CARTESIAN_POINT('Origin',(1.11022302462516E-15,0.999999999999982,
2.22044604925031E-15));
#146630=CARTESIAN_POINT('Origin',(1.11022302462516E-15,-1.77635683940025E-14,
2.22044604925031E-15));
#146631=CARTESIAN_POINT('',(-7.47957618,-1.00000000000002,-5.005590892));
#146632=CARTESIAN_POINT('',(-7.47957618,0.999999999999982,-5.005590892));
#146633=CARTESIAN_POINT('Ctrl Pts',(-7.47957617967883,-1.00000000029992,
-5.00559089166839));
#146634=CARTESIAN_POINT('Ctrl Pts',(-7.4202042336451,-0.888963444893636,
-4.96267463016275));
#146635=CARTESIAN_POINT('Ctrl Pts',(-7.37075526401692,-0.769956469741096,
-4.92693564225511));
#146636=CARTESIAN_POINT('Ctrl Pts',(-7.26420172190818,-0.424051722949988,
-4.84992888314661));
#146637=CARTESIAN_POINT('Ctrl Pts',(-7.23175500998826,-0.188791058808376,
-4.82648420105959));
#146638=CARTESIAN_POINT('Ctrl Pts',(-7.24178990103384,0.283921315909722,
-4.83373556418914));
#146639=CARTESIAN_POINT('Ctrl Pts',(-7.28419686186403,0.516830885584386,
-4.86437777775459));
#146640=CARTESIAN_POINT('Ctrl Pts',(-7.3948841469757,0.82623768465271,-4.94437499509896));
#146641=CARTESIAN_POINT('Ctrl Pts',(-7.43437942887842,0.915473690153646,
-4.9729209910481));
#146642=CARTESIAN_POINT('Ctrl Pts',(-7.47957617967883,1.00000000029988,
-5.00559089166839));
#146643=CARTESIAN_POINT('',(-7.542440507,-1.00000000000002,-4.910355506));
#146644=CARTESIAN_POINT('Origin',(1.11022302462516E-15,-1.00000000000002,
2.22044604925031E-15));
#146645=CARTESIAN_POINT('',(-7.542440507,0.999999999999982,-4.910355506));
#146646=CARTESIAN_POINT('Ctrl Pts',(-7.54244050680655,0.999999999960002,
-4.91035550643967));
#146647=CARTESIAN_POINT('Ctrl Pts',(-7.47964315154329,0.888963444646453,
-4.87262851828103));
#146648=CARTESIAN_POINT('Ctrl Pts',(-7.42734547678568,0.769956469604148,
-4.84120513431145));
#146649=CARTESIAN_POINT('Ctrl Pts',(-7.31465741384491,0.424051722941438,
-4.77349177711883));
#146650=CARTESIAN_POINT('Ctrl Pts',(-7.28034700755391,0.188791058807605,
-4.75287047132402));
#146651=CARTESIAN_POINT('Ctrl Pts',(-7.29095880071433,-0.28392131589928,
-4.75924786510321));
#146652=CARTESIAN_POINT('Ctrl Pts',(-7.33580216424091,-0.516830885569566,
-4.78619908634786));
#146653=CARTESIAN_POINT('Ctrl Pts',(-7.45286470105418,-0.826237684516339,
-4.85653821008756));
#146654=CARTESIAN_POINT('Ctrl Pts',(-7.49463617150114,-0.915473689909019,
-4.88163592765425));
#146655=CARTESIAN_POINT('Ctrl Pts',(-7.54244050680655,-0.999999999960038,
-4.91035550643967));
#146656=CARTESIAN_POINT('Origin',(1.11022302462516E-15,0.999999999999982,
2.22044604925031E-15));
#146657=CARTESIAN_POINT('Origin',(1.11022302462516E-15,-1.77635683940025E-14,
2.22044604925031E-15));
#146658=CARTESIAN_POINT('',(-7.898163313,-1.00000000000002,-4.314975815));
#146659=CARTESIAN_POINT('',(-7.898163313,0.999999999999982,-4.314975815));
#146660=CARTESIAN_POINT('Ctrl Pts',(-7.89816331281296,-1.0000000001015,
-4.31497581501368));
#146661=CARTESIAN_POINT('Ctrl Pts',(-7.8351833967921,-0.888963444754436,
-4.27755438203096));
#146662=CARTESIAN_POINT('Ctrl Pts',(-7.78272987602674,-0.769956469672355,
-4.24639184029317));
#146663=CARTESIAN_POINT('Ctrl Pts',(-7.66970245447833,-0.424051722955077,
-4.1792464736998));
#146664=CARTESIAN_POINT('Ctrl Pts',(-7.63528479837203,-0.188791058808791,
-4.15880467385859));
#146665=CARTESIAN_POINT('Ctrl Pts',(-7.64592929907974,0.283921315916024,
-4.16512732442939));
#146666=CARTESIAN_POINT('Ctrl Pts',(-7.69091228881307,0.516830885593306,
-4.19184485076974));
#146667=CARTESIAN_POINT('Ctrl Pts',(-7.80832487473718,0.826237684586908,
-4.26159809102287));
#146668=CARTESIAN_POINT('Ctrl Pts',(-7.8502200035666,0.915473690017277,
-4.28648883936674));
#146669=CARTESIAN_POINT('Ctrl Pts',(-7.89816331281296,1.00000000010146,
-4.31497581501368));
#146670=CARTESIAN_POINT('',(-7.952237733,-1.00000000000002,-4.214488703));
#146671=CARTESIAN_POINT('Origin',(1.11022302462516E-15,-1.00000000000002,
2.22044604925031E-15));
#146672=CARTESIAN_POINT('',(-7.952237734,0.999999999999982,-4.214488703));
#146673=CARTESIAN_POINT('Ctrl Pts',(-7.9522377334233,1.00000000018981,-4.21448870353033));
#146674=CARTESIAN_POINT('Ctrl Pts',(-7.8863113606651,0.888963444813991,
-4.18254270459723));
#146675=CARTESIAN_POINT('Ctrl Pts',(-7.83140745051944,0.769956469697667,
-4.15593374930452));
#146676=CARTESIAN_POINT('Ctrl Pts',(-7.71310325805011,0.424051722948052,
-4.09859426618526));
#146677=CARTESIAN_POINT('Ctrl Pts',(-7.67708249577676,0.188791058808185,
-4.08113153679338));
#146678=CARTESIAN_POINT('Ctrl Pts',(-7.68822323414686,-0.283921315907398,
-4.08653202326161));
#146679=CARTESIAN_POINT('Ctrl Pts',(-7.73530196031026,-0.516830885581081,
-4.10935501872354));
#146680=CARTESIAN_POINT('Ctrl Pts',(-7.8581983881465,-0.8262376844579,-4.16891757298584));
#146681=CARTESIAN_POINT('Ctrl Pts',(-7.90205144094031,-0.915473689783842,
-4.19016988878227));
#146682=CARTESIAN_POINT('Ctrl Pts',(-7.95223773317769,-0.999999999776178,
-4.21448870341132));
#146683=CARTESIAN_POINT('Origin',(1.11022302462516E-15,0.999999999999982,
2.22044604925031E-15));
#146684=CARTESIAN_POINT('Origin',(1.11022302462516E-15,-1.77635683940025E-14,
2.22044604925031E-15));
#146685=CARTESIAN_POINT('',(-8.253159079,-1.00000000000002,-3.58961909));
#146686=CARTESIAN_POINT('',(-8.253159079,0.999999999999982,-3.58961909));
#146687=CARTESIAN_POINT('Ctrl Pts',(-8.25315907914881,-0.999999999891681,
-3.58961909006943));
#146688=CARTESIAN_POINT('Ctrl Pts',(-8.18707827043164,-0.888963444602147,
-3.55799378091446));
#146689=CARTESIAN_POINT('Ctrl Pts',(-8.13204252346783,-0.76995646958845,
-3.5316585877518));
#146690=CARTESIAN_POINT('Ctrl Pts',(-8.01345125288575,-0.424051722950383,
-3.47491522857435));
#146691=CARTESIAN_POINT('Ctrl Pts',(-7.97733976334233,-0.188791058808387,
-3.45764089629977));
#146692=CARTESIAN_POINT('Ctrl Pts',(-7.98850817044388,0.283921315910252,
-3.46298392805613));
#146693=CARTESIAN_POINT('Ctrl Pts',(-8.03570501247084,0.516830885585125,
-3.48556165340058));
#146694=CARTESIAN_POINT('Ctrl Pts',(-8.15889756203451,0.826237684503461,
-3.5445093046019));
#146695=CARTESIAN_POINT('Ctrl Pts',(-8.20285522282177,0.915473689866596,
-3.56554439971813));
#146696=CARTESIAN_POINT('Ctrl Pts',(-8.25315907914881,0.999999999891645,
-3.58961909006943));
#146697=CARTESIAN_POINT('',(-8.298008217,-1.00000000000002,-3.484689316));
#146698=CARTESIAN_POINT('Origin',(1.11022302462516E-15,-1.00000000000002,
2.22044604925031E-15));
#146699=CARTESIAN_POINT('',(-8.298008217,0.999999999999982,-3.484689316));
#146700=CARTESIAN_POINT('Ctrl Pts',(-8.29800821680407,0.999999999999763,
-3.48468931651914));
#146701=CARTESIAN_POINT('Ctrl Pts',(-8.22948362702398,0.888963444677762,
-3.4587815173023));
#146702=CARTESIAN_POINT('Ctrl Pts',(-8.17241553555401,0.769956469625439,
-3.43720123042082));
#146703=CARTESIAN_POINT('Ctrl Pts',(-8.04944772936533,0.424051722947192,
-3.39069728527389));
#146704=CARTESIAN_POINT('Ctrl Pts',(-8.01200662909584,0.188791058808111,
-3.37653373193536));
#146705=CARTESIAN_POINT('Ctrl Pts',(-8.02358661400347,-0.28392131590634,
-3.38091382954382));
#146706=CARTESIAN_POINT('Ctrl Pts',(-8.07252165259768,-0.51683088557958,
-3.39942484185536));
#146707=CARTESIAN_POINT('Ctrl Pts',(-8.20026248178415,-0.826237684538798,
-3.447731263932));
#146708=CARTESIAN_POINT('Ctrl Pts',(-8.24584403802863,-0.915473689940681,
-3.46496706682217));
#146709=CARTESIAN_POINT('Ctrl Pts',(-8.29800821680408,-0.999999999999801,
-3.48468931651914));
#146710=CARTESIAN_POINT('Origin',(1.11022302462516E-15,0.999999999999982,
2.22044604925031E-15));
#146711=CARTESIAN_POINT('Origin',(1.11022302462516E-15,-1.77635683940025E-14,
2.22044604925031E-15));
#146712=CARTESIAN_POINT('',(-8.541705262,-1.00000000000002,-2.835360862));
#146713=CARTESIAN_POINT('',(-8.541705262,0.999999999999982,-2.835360862));
#146714=CARTESIAN_POINT('Ctrl Pts',(-8.54170526179937,-1.00000000003984,
-2.83536086236564));
#146715=CARTESIAN_POINT('Ctrl Pts',(-8.47305560408872,-0.888963444708826,
-2.80978630543292));
#146716=CARTESIAN_POINT('Ctrl Pts',(-8.41588074631203,-0.76995646964581,
-2.78849049633943));
#146717=CARTESIAN_POINT('Ctrl Pts',(-8.29268045378883,-0.424051722952022,
-2.74260600880005));
#146718=CARTESIAN_POINT('Ctrl Pts',(-8.25516587927573,-0.188791058808552,
-2.72863822688283));
#146719=CARTESIAN_POINT('Ctrl Pts',(-8.26676827132905,0.283921315912211,
-2.73295862086762));
#146720=CARTESIAN_POINT('Ctrl Pts',(-8.31579896444622,0.51683088558791,
-2.75121476261534));
#146721=CARTESIAN_POINT('Ctrl Pts',(-8.4437796037711,0.826237684560039,
-2.79888221287883));
#146722=CARTESIAN_POINT('Ctrl Pts',(-8.48944587536211,0.915473689971902,
-2.81589229255365));
#146723=CARTESIAN_POINT('Ctrl Pts',(-8.54170526179937,1.00000000003981,
-2.83536086236564));
#146724=CARTESIAN_POINT('',(-8.576968018,-1.00000000000002,-2.726833259));
#146725=CARTESIAN_POINT('Origin',(1.11022302462516E-15,-1.00000000000002,
2.22044604925031E-15));
#146726=CARTESIAN_POINT('',(-8.576968018,0.999999999999982,-2.726833259));
#146727=CARTESIAN_POINT('Ctrl Pts',(-8.57696801766623,1.00000000014478,
-2.72683325938025));
#146728=CARTESIAN_POINT('Ctrl Pts',(-8.50639693048896,0.888963444783311,
-2.70717225418446));
#146729=CARTESIAN_POINT('Ctrl Pts',(-8.447624136351,0.769956469684066,-2.69079438744693));
#146730=CARTESIAN_POINT('Ctrl Pts',(-8.32098278088487,0.424051722950983,
-2.65550040263088));
#146731=CARTESIAN_POINT('Ctrl Pts',(-8.28242279634777,0.188791058808389,
-2.64475006193496));
#146732=CARTESIAN_POINT('Ctrl Pts',(-8.29434879256285,-0.283921315911112,
-2.64807450471779));
#146733=CARTESIAN_POINT('Ctrl Pts',(-8.34474614742513,-0.51683088558632,
-2.66212449411069));
#146734=CARTESIAN_POINT('Ctrl Pts',(-8.4763028838897,-0.826237684597308,
-2.6987858491335));
#146735=CARTESIAN_POINT('Ctrl Pts',(-8.52324594767412,-0.915473690045215,
-2.71186636657059));
#146736=CARTESIAN_POINT('Ctrl Pts',(-8.57696801766623,-1.00000000014482,
-2.72683325938025));
#146737=CARTESIAN_POINT('Origin',(1.11022302462516E-15,0.999999999999982,
2.22044604925031E-15));
#146738=CARTESIAN_POINT('Origin',(1.11022302462516E-15,-1.77635683940025E-14,
2.22044604925031E-15));
#146739=CARTESIAN_POINT('',(-8.761478656,-1.00000000000002,-2.058273977));
#146740=CARTESIAN_POINT('',(-8.761478656,0.999999999999982,-2.058273976));
#146741=CARTESIAN_POINT('Ctrl Pts',(-8.76147865594458,-1.00000000014044,
-2.0582739763956));
#146742=CARTESIAN_POINT('Ctrl Pts',(-8.69081287594316,-0.888963444777773,
-2.03895608293596));
#146743=CARTESIAN_POINT('Ctrl Pts',(-8.63195924570962,-0.76995646967708,
-2.02287111920752));
#146744=CARTESIAN_POINT('Ctrl Pts',(-8.50514186759658,-0.424051722946195,
-1.9882149381297));
#146745=CARTESIAN_POINT('Ctrl Pts',(-8.46652625341952,-0.188791058808052,
-1.97766616690805));
#146746=CARTESIAN_POINT('Ctrl Pts',(-8.47846921478163,0.283921315905045,
-1.98092913785784));
#146747=CARTESIAN_POINT('Ctrl Pts',(-8.52893899266448,0.516830885577757,
-1.99471670832764));
#146748=CARTESIAN_POINT('Ctrl Pts',(-8.66067729683783,0.82623768454449,
-2.03072016746058));
#146749=CARTESIAN_POINT('Ctrl Pts',(-8.70768450122283,0.915473689953664,
-2.04356827655552));
#146750=CARTESIAN_POINT('Ctrl Pts',(-8.76147865586744,1.00000000001919,
-2.05827397637451));
#146751=CARTESIAN_POINT('',(-8.786871115,-1.00000000000002,-1.947022346));
#146752=CARTESIAN_POINT('Origin',(1.11022302462516E-15,-1.00000000000002,
2.22044604925031E-15));
#146753=CARTESIAN_POINT('',(-8.786871115,0.999999999999982,-1.947022345));
#146754=CARTESIAN_POINT('Ctrl Pts',(-8.78687111468735,1.00000000013172,
-1.94702234559588));
#146755=CARTESIAN_POINT('Ctrl Pts',(-8.71482172704382,0.888963444773288,
-1.93376643331344));
#146756=CARTESIAN_POINT('Ctrl Pts',(-8.65481743424227,0.769956469677657,
-1.92272285170412));
#146757=CARTESIAN_POINT('Ctrl Pts',(-8.52552217123474,0.424051722949631,
-1.89892299368291));
#146758=CARTESIAN_POINT('Ctrl Pts',(-8.48615376474826,0.188791058808297,
-1.89167242106493));
#146759=CARTESIAN_POINT('Ctrl Pts',(-8.49832975116214,-0.283921315909391,
-1.89391444255924));
#146760=CARTESIAN_POINT('Ctrl Pts',(-8.54978365242985,-0.516830885583895,
-1.90339028676294));
#146761=CARTESIAN_POINT('Ctrl Pts',(-8.68409707869062,-0.826237684621147,
-1.92811139900698));
#146762=CARTESIAN_POINT('Ctrl Pts',(-8.73202369206082,-0.915473690093675,
-1.93693131433199));
#146763=CARTESIAN_POINT('Ctrl Pts',(-8.78687111474132,-1.00000000021493,
-1.94702234560581));
#146764=CARTESIAN_POINT('Origin',(1.11022302462516E-15,0.999999999999982,
2.22044604925031E-15));
#146765=CARTESIAN_POINT('Origin',(1.11022302462516E-15,-1.77635683940025E-14,
2.22044604925031E-15));
#146766=CARTESIAN_POINT('',(-8.910709775,-1.00000000000002,-1.264615079));
#146767=CARTESIAN_POINT('',(-8.910709775,0.999999999999982,-1.264615079));
#146768=CARTESIAN_POINT('Ctrl Pts',(-8.91070977524219,-0.999999999833344,
-1.26461507908072));
#146769=CARTESIAN_POINT('Ctrl Pts',(-8.83859683236404,-0.88896344455949,
-1.25170938549311));
#146770=CARTESIAN_POINT('Ctrl Pts',(-8.77853828457743,-0.769956469564433,
-1.24096477386405));
#146771=CARTESIAN_POINT('Ctrl Pts',(-8.64912487986267,-0.424051722948457,
-1.21781593054578));
#146772=CARTESIAN_POINT('Ctrl Pts',(-8.60971913623194,-0.188791058808239,
-1.21077110255088));
#146773=CARTESIAN_POINT('Ctrl Pts',(-8.62190650920452,0.283921315907843,
-1.21295037893394));
#146774=CARTESIAN_POINT('Ctrl Pts',(-8.67340901888981,0.516830885581718,
-1.2221583686789));
#146775=CARTESIAN_POINT('Ctrl Pts',(-8.80784430855032,0.826237684479383,
-1.24620795789709));
#146776=CARTESIAN_POINT('Ctrl Pts',(-8.85581397133016,0.915473689824291,
-1.25479065095093));
#146777=CARTESIAN_POINT('Ctrl Pts',(-8.91070977524219,0.999999999833308,
-1.26461507908072));
#146778=CARTESIAN_POINT('',(-8.926027492,-1.00000000000002,-1.151535151));
#146779=CARTESIAN_POINT('Origin',(1.11022302462516E-15,-1.00000000000002,
2.22044604925031E-15));
#146780=CARTESIAN_POINT('',(-8.926027492,0.999999999999982,-1.151535151));
#146781=CARTESIAN_POINT('Ctrl Pts',(-8.92602749223077,0.999999999828974,
-1.15153515131936));
#146782=CARTESIAN_POINT('Ctrl Pts',(-8.85307990351357,0.888963444557654,
-1.14479106076095));
#146783=CARTESIAN_POINT('Ctrl Pts',(-8.79232723139907,0.769956469565621,
-1.13917068070444));
#146784=CARTESIAN_POINT('Ctrl Pts',(-8.66141907032706,0.424051722951004,
-1.12705657192987));
#146785=CARTESIAN_POINT('Ctrl Pts',(-8.6215592131525,0.188791058808435,
-1.12336414473294));
#146786=CARTESIAN_POINT('Ctrl Pts',(-8.63388715588222,-0.28392131591104,
-1.12450569350138));
#146787=CARTESIAN_POINT('Ctrl Pts',(-8.68598332699613,-0.516830885586241,
-1.12933109859575));
#146788=CARTESIAN_POINT('Ctrl Pts',(-8.82197203024378,-0.826237684481343,
-1.14191292820707));
#146789=CARTESIAN_POINT('Ctrl Pts',(-8.87049631618663,-0.915473689822921,
-1.14640122864087));
#146790=CARTESIAN_POINT('Ctrl Pts',(-8.92602749223077,-0.999999999829011,
-1.15153515131936));
#146791=CARTESIAN_POINT('Origin',(1.11022302462516E-15,0.999999999999982,
2.22044604925031E-15));
#146792=CARTESIAN_POINT('Origin',(1.11022302462516E-15,-1.77635683940025E-14,
2.22044604925031E-15));
#146793=CARTESIAN_POINT('',(-8.988197099,-1.00000000000002,-0.460774244));
#146794=CARTESIAN_POINT('',(-8.988197099,0.999999999999982,-0.460774244));
#146795=CARTESIAN_POINT('Ctrl Pts',(-8.98819709915994,-0.999999999884686,
-0.4607742441774));
#146796=CARTESIAN_POINT('Ctrl Pts',(-8.91521760431959,-0.888963444596554,
-0.454384659487097));
#146797=CARTESIAN_POINT('Ctrl Pts',(-8.85443769501692,-0.769956469584521,
-0.449066909228443));
#146798=CARTESIAN_POINT('Ctrl Pts',(-8.72347022429716,-0.42405172294922,
-0.437611784522527));
#146799=CARTESIAN_POINT('Ctrl Pts',(-8.68359162309196,-0.188791058808321,
-0.434127620564106));
#146800=CARTESIAN_POINT('Ctrl Pts',(-8.69592528211311,0.283921315908748,
-0.435205656129234));
#146801=CARTESIAN_POINT('Ctrl Pts',(-8.74804585567359,0.51683088558301,
-0.439759927834076));
#146802=CARTESIAN_POINT('Ctrl Pts',(-8.88409573694761,0.82623768449924,
-0.451662014005326));
#146803=CARTESIAN_POINT('Ctrl Pts',(-8.93264163465328,0.915473689860902,
-0.455910188236057));
#146804=CARTESIAN_POINT('Ctrl Pts',(-8.98819709915994,0.999999999884654,
-0.460774244177401));
#146805=CARTESIAN_POINT('',(-8.993316745,-1.00000000000002,-0.346776472999999));
#146806=CARTESIAN_POINT('Origin',(1.11022302462516E-15,-1.00000000000002,
2.22044604925031E-15));
#146807=CARTESIAN_POINT('',(-8.993316745,0.999999999999982,-0.346776472999999));
#146808=CARTESIAN_POINT('Ctrl Pts',(-8.99331674501375,0.999999999990158,
-0.3467764734695));
#146809=CARTESIAN_POINT('Ctrl Pts',(-8.92005828617789,0.888963444672462,
-0.346598504082613));
#146810=CARTESIAN_POINT('Ctrl Pts',(-8.85904637943988,0.769956469625277,
-0.346446577571944));
#146811=CARTESIAN_POINT('Ctrl Pts',(-8.7275793157764,0.42405172295028,-0.346115753738565));
#146812=CARTESIAN_POINT('Ctrl Pts',(-8.68754893604615,0.188791058808367,
-0.34601120122187));
#146813=CARTESIAN_POINT('Ctrl Pts',(-8.69992957774535,-0.283921315910156,
-0.346043086182908));
#146814=CARTESIAN_POINT('Ctrl Pts',(-8.75224857096815,-0.516830885584984,
-0.346179200834906));
#146815=CARTESIAN_POINT('Ctrl Pts',(-8.88881765021394,-0.826237684539528,
-0.346520446308492));
#146816=CARTESIAN_POINT('Ctrl Pts',(-8.93754891983274,-0.915473689935909,
-0.346640994702772));
#146817=CARTESIAN_POINT('Ctrl Pts',(-8.99331674501375,-0.999999999990196,
-0.346776473469499));
#146818=CARTESIAN_POINT('Origin',(1.11022302462516E-15,0.999999999999982,
2.22044604925031E-15));
#146819=CARTESIAN_POINT('Origin',(1.11022302462516E-15,-1.77635683940025E-14,
2.22044604925031E-15));
#146820=CARTESIAN_POINT('',(-8.993316745,-1.00000000000002,0.346776472999999));
#146821=CARTESIAN_POINT('',(-8.993316745,0.999999999999982,0.346776472999999));
#146822=CARTESIAN_POINT('Ctrl Pts',(-8.99331674501319,-0.999999999990532,
0.346776473489777));
#146823=CARTESIAN_POINT('Ctrl Pts',(-8.92005828617723,-0.888963444672731,
0.34659850410287));
#146824=CARTESIAN_POINT('Ctrl Pts',(-8.85904637943913,-0.76995646962542,
0.346446577592178));
#146825=CARTESIAN_POINT('Ctrl Pts',(-8.72757931577561,-0.424051722950311,
0.346115753758762));
#146826=CARTESIAN_POINT('Ctrl Pts',(-8.68754893604535,-0.188791058808411,
0.346011201242062));
#146827=CARTESIAN_POINT('Ctrl Pts',(-8.69992957774455,0.283921315910098,
0.346043086203105));
#146828=CARTESIAN_POINT('Ctrl Pts',(-8.75224857096735,0.516830885584921,
0.346179200855117));
#146829=CARTESIAN_POINT('Ctrl Pts',(-8.88881765021319,0.826237684539586,
0.346520446328741));
#146830=CARTESIAN_POINT('Ctrl Pts',(-8.93754891983208,0.915473689936097,
0.346640994723034));
#146831=CARTESIAN_POINT('Ctrl Pts',(-8.99331674501319,0.999999999990497,
0.346776473489777));
#146832=CARTESIAN_POINT('',(-8.988197099,-1.00000000000002,0.460774244000002));
#146833=CARTESIAN_POINT('Origin',(1.11022302462516E-15,-1.00000000000002,
2.22044604925031E-15));
#146834=CARTESIAN_POINT('',(-8.988197099,0.999999999999982,0.460774244000002));
#146835=CARTESIAN_POINT('Ctrl Pts',(-8.9881970991918,0.999999999893167,
0.460774243665518));
#146836=CARTESIAN_POINT('Ctrl Pts',(-8.91521760434871,0.888963444601223,
0.454384658959215));
#146837=CARTESIAN_POINT('Ctrl Pts',(-8.85443769504401,0.76995646958464,
0.449066908687328));
#146838=CARTESIAN_POINT('Ctrl Pts',(-8.72347022432541,0.424051722946442,
0.437611783953442));
#146839=CARTESIAN_POINT('Ctrl Pts',(-8.6835916231211,0.188791058808023,
0.434127619986628));
#146840=CARTESIAN_POINT('Ctrl Pts',(-8.69592528214153,-0.283921315905468,
0.435205655554325));
#146841=CARTESIAN_POINT('Ctrl Pts',(-8.74804585570079,-0.516830885578331,
0.439759927270136));
#146842=CARTESIAN_POINT('Ctrl Pts',(-8.88409573697414,-0.826237684498686,
0.451662013470531));
#146843=CARTESIAN_POINT('Ctrl Pts',(-8.93264163468216,-0.915473689865192,
0.455910187711916));
#146844=CARTESIAN_POINT('Ctrl Pts',(-8.9881970991918,-0.9999999998932,0.460774243665518));
#146845=CARTESIAN_POINT('Origin',(1.11022302462516E-15,0.999999999999982,
2.22044604925031E-15));
#146846=CARTESIAN_POINT('Origin',(1.11022302462516E-15,-1.77635683940025E-14,
2.22044604925031E-15));
#146847=CARTESIAN_POINT('',(-8.926027492,-1.00000000000002,1.151535151));
#146848=CARTESIAN_POINT('',(-8.926027492,0.999999999999982,1.151535151));
#146849=CARTESIAN_POINT('Ctrl Pts',(-8.92602749221154,-0.999999999831735,
1.15153515148245));
#146850=CARTESIAN_POINT('Ctrl Pts',(-8.85307990349065,-0.888963444558428,
1.14479106093982));
#146851=CARTESIAN_POINT('Ctrl Pts',(-8.79232723137321,-0.769956469564023,
1.1391706808964));
#146852=CARTESIAN_POINT('Ctrl Pts',(-8.66141907029811,-0.424051722948626,
1.12705657215028));
#146853=CARTESIAN_POINT('Ctrl Pts',(-8.6215592131229,-0.188791058808234,
1.12336414496198));
#146854=CARTESIAN_POINT('Ctrl Pts',(-8.63388715585244,0.283921315908096,
1.1245056937277));
#146855=CARTESIAN_POINT('Ctrl Pts',(-8.68598332696715,0.516830885582066,
1.12933109881079));
#146856=CARTESIAN_POINT('Ctrl Pts',(-8.82197203021842,0.826237684479056,
1.14191292839256));
#146857=CARTESIAN_POINT('Ctrl Pts',(-8.87049631616405,0.915473689823283,
1.14640122881592));
#146858=CARTESIAN_POINT('Ctrl Pts',(-8.92602749221154,0.999999999831699,
1.15153515148245));
#146859=CARTESIAN_POINT('',(-8.910709775,-1.00000000000002,1.264615079));
#146860=CARTESIAN_POINT('Origin',(1.11022302462516E-15,-1.00000000000002,
2.22044604925031E-15));
#146861=CARTESIAN_POINT('',(-8.910709775,0.999999999999982,1.264615079));
#146862=CARTESIAN_POINT('Ctrl Pts',(-8.9107097753288,0.999999999842807,
1.26461507851505));
#146863=CARTESIAN_POINT('Ctrl Pts',(-8.83859683244852,0.888963444565195,
1.25170938491645));
#146864=CARTESIAN_POINT('Ctrl Pts',(-8.7785382846604,0.769956469565655,
1.24096477327833));
#146865=CARTESIAN_POINT('Ctrl Pts',(-8.64912487994753,0.424051722946345,
1.21781592994151));
#146866=CARTESIAN_POINT('Ctrl Pts',(-8.6097191363179,0.18879105880801,1.21077110194113));
#146867=CARTESIAN_POINT('Ctrl Pts',(-8.6219065092898,-0.28392131590536,
1.21295037832583));
#146868=CARTESIAN_POINT('Ctrl Pts',(-8.6734090189736,-0.516830885578178,
1.22215836807797));
#146869=CARTESIAN_POINT('Ctrl Pts',(-8.80784430863259,-0.82623768448008,
1.24620795731554));
#146870=CARTESIAN_POINT('Ctrl Pts',(-8.85581397141432,-0.915473689829693,
1.25479065037675));
#146871=CARTESIAN_POINT('Ctrl Pts',(-8.9107097753288,-0.999999999842844,
1.26461507851505));
#146872=CARTESIAN_POINT('Origin',(1.11022302462516E-15,0.999999999999982,
2.22044604925031E-15));
#146873=CARTESIAN_POINT('Origin',(1.11022302462516E-15,-1.77635683940025E-14,
2.22044604925031E-15));
#146874=CARTESIAN_POINT('',(-8.786871115,-1.00000000000002,1.947022345));
#146875=CARTESIAN_POINT('',(-8.786871115,0.999999999999982,1.947022345));
#146876=CARTESIAN_POINT('Ctrl Pts',(-8.78687111484236,-1.00000000011924,
1.9470223448582));
#146877=CARTESIAN_POINT('Ctrl Pts',(-8.71482172720569,-0.88896344476554,
1.93376643256629));
#146878=CARTESIAN_POINT('Ctrl Pts',(-8.65481743440953,-0.769956469675547,
1.92272285094909));
#146879=CARTESIAN_POINT('Ctrl Pts',(-8.52552217140722,-0.424051722951982,
1.89892299290974));
#146880=CARTESIAN_POINT('Ctrl Pts',(-8.48615376492161,-0.188791058808557,
1.89167242028618));
#146881=CARTESIAN_POINT('Ctrl Pts',(-8.49832975133559,0.283921315912148,
1.89391444178229));
#146882=CARTESIAN_POINT('Ctrl Pts',(-8.54978365260218,0.51683088558783,
1.90339028599331));
#146883=CARTESIAN_POINT('Ctrl Pts',(-8.68409707884375,0.826237684589113,
1.92811139825368));
#146884=CARTESIAN_POINT('Ctrl Pts',(-8.73202369219063,0.91547369002775,
1.9369313135815));
#146885=CARTESIAN_POINT('Ctrl Pts',(-8.78687111484236,1.0000000001192,1.9470223448582));
#146886=CARTESIAN_POINT('',(-8.761478656,-1.00000000000002,2.058273976));
#146887=CARTESIAN_POINT('Origin',(1.11022302462516E-15,-1.00000000000002,
2.22044604925031E-15));
#146888=CARTESIAN_POINT('',(-8.761478656,0.999999999999982,2.058273976));
#146889=CARTESIAN_POINT('Ctrl Pts',(-8.76147865610178,1.00000000003545,
2.05827397542386));
#146890=CARTESIAN_POINT('Ctrl Pts',(-8.69081287612847,0.888963444702555,
2.03895608197732));
#146891=CARTESIAN_POINT('Ctrl Pts',(-8.63195924591628,0.769956469637271,
2.02287111825923));
#146892=CARTESIAN_POINT('Ctrl Pts',(-8.50514186781518,0.424051722945794,
1.9882149371944));
#146893=CARTESIAN_POINT('Ctrl Pts',(-8.4665262536374,0.188791058807997,
1.97766616597551));
#146894=CARTESIAN_POINT('Ctrl Pts',(-8.47846921499966,-0.283921315904604,
1.98092913692443));
#146895=CARTESIAN_POINT('Ctrl Pts',(-8.52893899288346,-0.516830885577124,
1.9947167073906));
#146896=CARTESIAN_POINT('Ctrl Pts',(-8.66067729706199,-0.826237684549968,
2.03072016651486));
#146897=CARTESIAN_POINT('Ctrl Pts',(-8.70768450145157,-0.915473689964894,
2.04356827560746));
#146898=CARTESIAN_POINT('Ctrl Pts',(-8.76147865610178,-1.00000000003548,
2.05827397542386));
#146899=CARTESIAN_POINT('Origin',(1.11022302462516E-15,0.999999999999982,
2.22044604925031E-15));
#146900=CARTESIAN_POINT('Origin',(1.11022302462516E-15,-1.77635683940025E-14,
2.22044604925031E-15));
#146901=CARTESIAN_POINT('',(-8.576968018,-1.00000000000002,2.726833259));
#146902=CARTESIAN_POINT('',(-8.576968018,0.999999999999982,2.726833259));
#146903=CARTESIAN_POINT('Ctrl Pts',(-8.57696801776425,-1.00000000013926,
2.72683325905983));
#146904=CARTESIAN_POINT('Ctrl Pts',(-8.50639693059222,-0.888963444780249,
2.70717225385519));
#146905=CARTESIAN_POINT('Ctrl Pts',(-8.44762413645845,-0.769956469683948,
2.69079438711029));
#146906=CARTESIAN_POINT('Ctrl Pts',(-8.32098278099788,-0.424051722952772,
2.65550040227742));
#146907=CARTESIAN_POINT('Ctrl Pts',(-8.28242279646211,-0.188791058808596,
2.64475006157632));
#146908=CARTESIAN_POINT('Ctrl Pts',(-8.29434879267705,0.283921315913186,
2.64807450436084));
#146909=CARTESIAN_POINT('Ctrl Pts',(-8.34474614753761,0.516830885589286,
2.66212449376052));
#146910=CARTESIAN_POINT('Ctrl Pts',(-8.47630288399607,0.826237684597596,
2.69878584880073));
#146911=CARTESIAN_POINT('Ctrl Pts',(-8.52324594777668,0.91547369004237,
2.71186636624358));
#146912=CARTESIAN_POINT('Ctrl Pts',(-8.57696801776425,1.00000000013922,
2.72683325905983));
#146913=CARTESIAN_POINT('',(-8.541705262,-1.00000000000002,2.835360862));
#146914=CARTESIAN_POINT('Origin',(1.11022302462516E-15,-1.00000000000002,
2.22044604925031E-15));
#146915=CARTESIAN_POINT('',(-8.541705262,0.999999999999982,2.835360862));
#146916=CARTESIAN_POINT('Ctrl Pts',(-8.54170526175661,1.00000000003763,
2.83536086248987));
#146917=CARTESIAN_POINT('Ctrl Pts',(-8.47305560404579,0.888963444707527,
2.80978630556046));
#146918=CARTESIAN_POINT('Ctrl Pts',(-8.41588074626889,0.769956469645605,
2.78849049646969));
#146919=CARTESIAN_POINT('Ctrl Pts',(-8.29268045374403,0.424051722952567,
2.74260600893571));
#146920=CARTESIAN_POINT('Ctrl Pts',(-8.2551658792303,0.18879105880857,2.72863822702008));
#146921=CARTESIAN_POINT('Ctrl Pts',(-8.2667682712839,-0.28392131591296,
2.73295862100442));
#146922=CARTESIAN_POINT('Ctrl Pts',(-8.31579896440192,-0.516830885588963,
2.75121476275007));
#146923=CARTESIAN_POINT('Ctrl Pts',(-8.4437796037284,-0.826237684560064,
2.7988822130079));
#146924=CARTESIAN_POINT('Ctrl Pts',(-8.48944587531942,-0.915473689970771,
2.81589229268048));
#146925=CARTESIAN_POINT('Ctrl Pts',(-8.54170526175661,-1.00000000003766,
2.83536086248987));
#146926=CARTESIAN_POINT('Origin',(1.11022302462516E-15,0.999999999999982,
2.22044604925031E-15));
#146927=CARTESIAN_POINT('Origin',(1.11022302462516E-15,-1.77635683940025E-14,
2.22044604925031E-15));
#146928=CARTESIAN_POINT('',(-8.298008217,-1.00000000000002,3.484689316));
#146929=CARTESIAN_POINT('',(-8.298008217,0.999999999999982,3.484689317));
#146930=CARTESIAN_POINT('Ctrl Pts',(-8.29800821680649,-0.999999999999694,
3.48468931651321));
#146931=CARTESIAN_POINT('Ctrl Pts',(-8.22948362702784,-0.888963444677954,
3.4587815172934));
#146932=CARTESIAN_POINT('Ctrl Pts',(-8.17241553555906,-0.769956469625944,
3.43720123040945));
#146933=CARTESIAN_POINT('Ctrl Pts',(-8.04944772937249,-0.424051722947701,
3.39069728525703));
#146934=CARTESIAN_POINT('Ctrl Pts',(-8.0120066291036,-0.188791058808198,
3.37653373191682));
#146935=CARTESIAN_POINT('Ctrl Pts',(-8.02358661401112,0.28392131590686,
3.38091382952583));
#146936=CARTESIAN_POINT('Ctrl Pts',(-8.07252165260454,0.516830885580335,
3.39942484183956));
#146937=CARTESIAN_POINT('Ctrl Pts',(-8.2002624818134,0.826237684599012,
3.4477312639312));
#146938=CARTESIAN_POINT('Ctrl Pts',(-8.24584403809067,0.915473690055274,
3.4649670668361));
#146939=CARTESIAN_POINT('Ctrl Pts',(-8.29800821690682,1.00000000016222,
3.48468931655114));
#146940=CARTESIAN_POINT('',(-8.253159079,-1.00000000000002,3.58961909));
#146941=CARTESIAN_POINT('Origin',(1.11022302462516E-15,-1.00000000000002,
2.22044604925031E-15));
#146942=CARTESIAN_POINT('',(-8.253159079,0.999999999999982,3.58961909));
#146943=CARTESIAN_POINT('Ctrl Pts',(-8.2531590793014,0.999999999897838,
3.58961908972884));
#146944=CARTESIAN_POINT('Ctrl Pts',(-8.18707827057777,0.888963444607217,
3.55799378058502));
#146945=CARTESIAN_POINT('Ctrl Pts',(-8.13204252360867,0.769956469592236,
3.53165858743165));
#146946=CARTESIAN_POINT('Ctrl Pts',(-8.01345125301592,0.424051722951699,
3.47491522827454));
#146947=CARTESIAN_POINT('Ctrl Pts',(-7.97733976346943,0.188791058808483,
3.45764089600619));
#146948=CARTESIAN_POINT('Ctrl Pts',(-7.98850817057213,-0.283921315911911,
3.46298392776071));
#146949=CARTESIAN_POINT('Ctrl Pts',(-8.03570501260313,-0.51683088558747,
3.48556165309702));
#146950=CARTESIAN_POINT('Ctrl Pts',(-8.15889756217778,-0.826237684507599,
3.54450930427714));
#146951=CARTESIAN_POINT('Ctrl Pts',(-8.20285522296936,-0.915473689871845,
3.56554439938598));
#146952=CARTESIAN_POINT('Ctrl Pts',(-8.2531590793014,-0.999999999897872,
3.58961908972884));
#146953=CARTESIAN_POINT('Origin',(1.11022302462516E-15,0.999999999999982,
2.22044604925031E-15));
#146954=CARTESIAN_POINT('Origin',(1.11022302462516E-15,-1.77635683940025E-14,
2.22044604925031E-15));
#146955=CARTESIAN_POINT('',(-7.952237733,-1.00000000000002,4.214488703));
#146956=CARTESIAN_POINT('',(-7.952237733,0.999999999999982,4.214488703));
#146957=CARTESIAN_POINT('Ctrl Pts',(-7.95223773319635,-0.999999999775504,
4.21448870337516));
#146958=CARTESIAN_POINT('Ctrl Pts',(-7.88631136054351,-0.888963444517433,
4.18254270450202));
#146959=CARTESIAN_POINT('Ctrl Pts',(-7.83140745047794,-0.769956469541135,
4.15593374925552));
#146960=CARTESIAN_POINT('Ctrl Pts',(-7.71310325805549,-0.424051722947019,
4.0985942661749));
#146961=CARTESIAN_POINT('Ctrl Pts',(-7.6770824957803,-0.188791058808112,
4.08113153678696));
#146962=CARTESIAN_POINT('Ctrl Pts',(-7.68822323415081,0.283921315906088,
4.08653202325389));
#146963=CARTESIAN_POINT('Ctrl Pts',(-7.7353019603166,0.516830885579229,
4.10935501871067));
#146964=CARTESIAN_POINT('Ctrl Pts',(-7.85819838815941,0.826237684456182,
4.1689175729596));
#146965=CARTESIAN_POINT('Ctrl Pts',(-7.90205144095589,0.915473689782662,
4.19016988875141));
#146966=CARTESIAN_POINT('Ctrl Pts',(-7.95223773319635,0.999999999775469,
4.21448870337516));
#146967=CARTESIAN_POINT('',(-7.898163313,-1.00000000000002,4.314975815));
#146968=CARTESIAN_POINT('Origin',(1.11022302462516E-15,-1.00000000000002,
2.22044604925031E-15));
#146969=CARTESIAN_POINT('',(-7.898163313,0.999999999999982,4.314975815));
#146970=CARTESIAN_POINT('Ctrl Pts',(-7.89816331271264,1.00000000009806,
4.31497581519263));
#146971=CARTESIAN_POINT('Ctrl Pts',(-7.83518339669397,0.888963444751888,
4.277554382208));
#146972=CARTESIAN_POINT('Ctrl Pts',(-7.78272987593037,0.769956469670872,
4.24639184046861));
#146973=CARTESIAN_POINT('Ctrl Pts',(-7.66970245438489,0.424051722954907,
4.17924647387126));
#146974=CARTESIAN_POINT('Ctrl Pts',(-7.63528479827936,0.188791058808747,
4.15880467402877));
#146975=CARTESIAN_POINT('Ctrl Pts',(-7.64592929898681,-0.283921315915896,
4.16512732459995));
#146976=CARTESIAN_POINT('Ctrl Pts',(-7.69091228871914,-0.51683088559311,
4.19184485094197));
#146977=CARTESIAN_POINT('Ctrl Pts',(-7.80832487464018,-0.826237684585493,
4.26159809119923));
#146978=CARTESIAN_POINT('Ctrl Pts',(-7.85022000346807,-0.915473690014822,
4.28648883954432));
#146979=CARTESIAN_POINT('Ctrl Pts',(-7.89816331271264,-1.00000000009809,
4.31497581519263));
#146980=CARTESIAN_POINT('Origin',(1.11022302462516E-15,0.999999999999982,
2.22044604925031E-15));
#146981=CARTESIAN_POINT('Origin',(1.11022302462516E-15,-1.77635683940025E-14,
2.22044604925031E-15));
#146982=CARTESIAN_POINT('',(-7.542440507,-1.00000000000002,4.910355505));
#146983=CARTESIAN_POINT('',(-7.542440507,0.999999999999982,4.910355506));
#146984=CARTESIAN_POINT('Ctrl Pts',(-7.54244050699415,-0.999999999713363,
4.91035550585342));
#146985=CARTESIAN_POINT('Ctrl Pts',(-7.47964315180284,-0.888963444471708,
4.87262851771894));
#146986=CARTESIAN_POINT('Ctrl Pts',(-7.42734547710069,-0.769956469514917,
4.84120513376689));
#146987=CARTESIAN_POINT('Ctrl Pts',(-7.31465741420512,-0.424051722944422,
4.77349177656748));
#146988=CARTESIAN_POINT('Ctrl Pts',(-7.28034700791849,-0.18879105880793,
4.75287047076504));
#146989=CARTESIAN_POINT('Ctrl Pts',(-7.29095880107796,0.283921315902793,
4.75924786454684));
#146990=CARTESIAN_POINT('Ctrl Pts',(-7.33580216459887,0.516830885574576,
4.78619908580148));
#146991=CARTESIAN_POINT('Ctrl Pts',(-7.4528647013947,0.82623768451662,4.85653820956603));
#146992=CARTESIAN_POINT('Ctrl Pts',(-7.49463617183292,0.915473689903834,
4.88163592714012));
#146993=CARTESIAN_POINT('Ctrl Pts',(-7.54244050712803,0.999999999950053,
4.91035550593385));
#146994=CARTESIAN_POINT('',(-7.47957618,-1.00000000000002,5.005590891));
#146995=CARTESIAN_POINT('Origin',(1.11022302462516E-15,-1.00000000000002,
2.22044604925031E-15));
#146996=CARTESIAN_POINT('',(-7.47957618,0.999999999999982,5.005590891));
#146997=CARTESIAN_POINT('Ctrl Pts',(-7.47957617982888,1.00000000003923,
5.00559089113518));
#146998=CARTESIAN_POINT('Ctrl Pts',(-7.42020423385493,0.888963444707323,
4.96267462967732));
#146999=CARTESIAN_POINT('Ctrl Pts',(-7.37075526427221,0.769956469643229,
4.92693564180633));
#147000=CARTESIAN_POINT('Ctrl Pts',(-7.2642017221897,0.4240517229499,4.84992888272496));
#147001=CARTESIAN_POINT('Ctrl Pts',(-7.2317550102686,0.188791058808352,
4.82648420063956));
#147002=CARTESIAN_POINT('Ctrl Pts',(-7.24178990131453,-0.283921315909654,
4.83373556376861));
#147003=CARTESIAN_POINT('Ctrl Pts',(-7.28419686214626,-0.516830885584279,
4.8643777773319));
#147004=CARTESIAN_POINT('Ctrl Pts',(-7.39488414722774,-0.826237684556974,
4.94437499464598));
#147005=CARTESIAN_POINT('Ctrl Pts',(-7.43437942908497,-0.915473689970183,
4.9729209905592));
#147006=CARTESIAN_POINT('Ctrl Pts',(-7.47957617982888,-1.00000000003927,
5.00559089113518));
#147007=CARTESIAN_POINT('Origin',(1.11022302462516E-15,0.999999999999982,
2.22044604925031E-15));
#147008=CARTESIAN_POINT('Origin',(1.11022302462516E-15,-1.77635683940025E-14,
2.22044604925031E-15));
#147009=CARTESIAN_POINT('',(-7.071915986,-1.00000000000002,5.566687012));
#147010=CARTESIAN_POINT('',(-7.071915985,0.999999999999982,5.566687013));
#147011=CARTESIAN_POINT('Ctrl Pts',(-7.07191598537279,-1.00000000011093,
5.56668701257385));
#147012=CARTESIAN_POINT('Ctrl Pts',(-7.01275325493728,-0.888963444757717,
5.52348279059388));
#147013=CARTESIAN_POINT('Ctrl Pts',(-6.96348288566105,-0.76995646966828,
5.48749798046137));
#147014=CARTESIAN_POINT('Ctrl Pts',(-6.85731825030078,-0.424051722948235,
5.40995593718119));
#147015=CARTESIAN_POINT('Ctrl Pts',(-6.82499444723148,-0.188791058808213,
5.38634208557447));
#147016=CARTESIAN_POINT('Ctrl Pts',(-6.83499185525838,0.283921315907589,
5.39364503965271));
#147017=CARTESIAN_POINT('Ctrl Pts',(-6.87723880372388,0.516830885581356,
5.42450749134371));
#147018=CARTESIAN_POINT('Ctrl Pts',(-6.98752493069895,0.826237684544213,
5.50505685541549));
#147019=CARTESIAN_POINT('Ctrl Pts',(-7.02687849941884,0.915473689949042,
5.53379790271954));
#147020=CARTESIAN_POINT('Ctrl Pts',(-7.07191598531943,1.00000000001076,
5.56668701253488));
#147021=CARTESIAN_POINT('',(-7.000767897,-1.00000000000002,5.655903894));
#147022=CARTESIAN_POINT('Origin',(1.11022302462516E-15,-1.00000000000002,
2.22044604925031E-15));
#147023=CARTESIAN_POINT('',(-7.000767897,0.999999999999982,5.655903894));
#147024=CARTESIAN_POINT('Ctrl Pts',(-7.00076789681103,1.00000000017972,
5.65590389380216));
#147025=CARTESIAN_POINT('Ctrl Pts',(-6.94548194883083,0.888963444807022,
5.60783834035334));
#147026=CARTESIAN_POINT('Ctrl Pts',(-6.89943566441819,0.76995646969442,
5.56781065565214));
#147027=CARTESIAN_POINT('Ctrl Pts',(-6.8002139082344,0.42405172294853,5.48156251723961));
#147028=CARTESIAN_POINT('Ctrl Pts',(-6.76999938234043,0.188791058808214,
5.4553037157138));
#147029=CARTESIAN_POINT('Ctrl Pts',(-6.77934386868416,-0.283921315908009,
5.46342540768646));
#147030=CARTESIAN_POINT('Ctrl Pts',(-6.818833364706,-0.516830885581938,
5.49774559537489));
#147031=CARTESIAN_POINT('Ctrl Pts',(-6.92190416004712,-0.826237684606702,
5.58734269918266));
#147032=CARTESIAN_POINT('Ctrl Pts',(-6.958681602184,-0.915473690068199,
5.61931410710659));
#147033=CARTESIAN_POINT('Ctrl Pts',(-7.00076789681103,-1.00000000017975,
5.65590389380216));
#147034=CARTESIAN_POINT('Origin',(1.11022302462516E-15,0.999999999999982,
2.22044604925031E-15));
#147035=CARTESIAN_POINT('Origin',(1.11022302462516E-15,-1.77635683940025E-14,
2.22044604925031E-15));
#147036=CARTESIAN_POINT('',(-6.544452554,-1.00000000000002,6.178198829));
#147037=CARTESIAN_POINT('',(-6.544452554,0.999999999999982,6.178198829));
#147038=CARTESIAN_POINT('Ctrl Pts',(-6.54445255416351,-1.0000000000805,
6.17819882862887));
#147039=CARTESIAN_POINT('Ctrl Pts',(-6.4894007921,-0.88896344473667,6.12986522787584));
#147040=CARTESIAN_POINT('Ctrl Pts',(-6.44355442436669,-0.769956469658397,
6.08960872015794));
#147041=CARTESIAN_POINT('Ctrl Pts',(-6.34476799180017,-0.424051722949622,
6.00286231379506));
#147042=CARTESIAN_POINT('Ctrl Pts',(-6.31469104420046,-0.188791058808342,
5.97644604124084));
#147043=CARTESIAN_POINT('Ctrl Pts',(-6.32399357384458,0.283921315909262,
5.98461575652057));
#147044=CARTESIAN_POINT('Ctrl Pts',(-6.36330395967153,0.516830885583727,
6.01914095232269));
#147045=CARTESIAN_POINT('Ctrl Pts',(-6.46592571779309,0.826237684571677,
6.10925202055845));
#147046=CARTESIAN_POINT('Ctrl Pts',(-6.50254453300505,0.915473689998982,
6.14140499157264));
#147047=CARTESIAN_POINT('Ctrl Pts',(-6.54445255416351,1.00000000008046,
6.17819882862886));
#147048=CARTESIAN_POINT('',(-6.465593548,-1.00000000000002,6.260678883));
#147049=CARTESIAN_POINT('Origin',(1.11022302462516E-15,-1.00000000000002,
2.22044604925031E-15));
#147050=CARTESIAN_POINT('',(-6.465593547,0.999999999999982,6.260678883));
#147051=CARTESIAN_POINT('Ctrl Pts',(-6.46559354762128,0.999999999811353,
6.26067888279958));
#147052=CARTESIAN_POINT('Ctrl Pts',(-6.41483872768217,0.888963444543266,
6.20785103304572));
#147053=CARTESIAN_POINT('Ctrl Pts',(-6.37256586612412,0.769956469555061,
6.1638569309814));
#147054=CARTESIAN_POINT('Ctrl Pts',(-6.28147477111903,0.424051722947448,
6.06906183260181));
#147055=CARTESIAN_POINT('Ctrl Pts',(-6.25373570084517,0.188791058808131,
6.04020033207072));
#147056=CARTESIAN_POINT('Ctrl Pts',(-6.26231454617831,-0.283921315906657,
6.04912696179709));
#147057=CARTESIAN_POINT('Ctrl Pts',(-6.29856863119255,-0.516830885580028,
6.08684879763255));
#147058=CARTESIAN_POINT('Ctrl Pts',(-6.39319307134218,-0.826237684586883,
6.18532440469952));
#147059=CARTESIAN_POINT('Ctrl Pts',(-6.42695656339071,-0.91547369003238,
6.22046380962379));
#147060=CARTESIAN_POINT('Ctrl Pts',(-6.46559354776686,-1.00000000012986,
6.26067888295109));
#147061=CARTESIAN_POINT('Origin',(1.11022302462516E-15,0.999999999999982,
2.22044604925031E-15));
#147062=CARTESIAN_POINT('Origin',(1.11022302462516E-15,-1.77635683940025E-14,
2.22044604925031E-15));
#147063=CARTESIAN_POINT('',(-5.964297039,-1.00000000000002,6.739967421));
#147064=CARTESIAN_POINT('',(-5.964297039,0.999999999999982,6.73996742));
#147065=CARTESIAN_POINT('Ctrl Pts',(-5.96429703935934,-1.00000000016049,
6.73996742032238));
#147066=CARTESIAN_POINT('Ctrl Pts',(-5.91379949005691,-0.888963444794064,
6.68689359451439));
#147067=CARTESIAN_POINT('Ctrl Pts',(-5.87174625183969,-0.769956469688926,
6.64268951092948));
#147068=CARTESIAN_POINT('Ctrl Pts',(-5.78113339231567,-0.424051722950078,
6.54743717254365));
#147069=CARTESIAN_POINT('Ctrl Pts',(-5.75354546207987,-0.188791058808362,
6.51843116733989));
#147070=CARTESIAN_POINT('Ctrl Pts',(-5.76207821484306,0.283921315909882,
6.52740186607612));
#147071=CARTESIAN_POINT('Ctrl Pts',(-5.79813553392257,0.516830885584602,
6.56531182940825));
#147072=CARTESIAN_POINT('Ctrl Pts',(-5.89226667310739,0.826237684479476,
6.66425908042156));
#147073=CARTESIAN_POINT('Ctrl Pts',(-5.92585590159545,0.915473689821207,
6.69956509827457));
#147074=CARTESIAN_POINT('Ctrl Pts',(-5.96429703920789,0.999999999827432,
6.7399674201632));
#147075=CARTESIAN_POINT('',(-5.87836204,-1.00000000000002,6.815046568));
#147076=CARTESIAN_POINT('Origin',(1.11022302462516E-15,-1.00000000000002,
2.22044604925031E-15));
#147077=CARTESIAN_POINT('',(-5.87836204,0.999999999999982,6.815046568));
#147078=CARTESIAN_POINT('Ctrl Pts',(-5.87836203971057,0.999999999954792,
6.81504656831974));
#147079=CARTESIAN_POINT('Ctrl Pts',(-5.8325469956454,0.888963444648911,
6.75788176096771));
#147080=CARTESIAN_POINT('Ctrl Pts',(-5.79438791306314,0.769956469615795,
6.71027545612482));
#147081=CARTESIAN_POINT('Ctrl Pts',(-5.7121608910693,0.424051722953674,
6.60769663216305));
#147082=CARTESIAN_POINT('Ctrl Pts',(-5.68712061508326,0.188791058808645,
6.57646480847093));
#147083=CARTESIAN_POINT('Ctrl Pts',(-5.69486474759318,-0.28392131591436,
6.58612450397438));
#147084=CARTESIAN_POINT('Ctrl Pts',(-5.72759152504513,-0.516830885590938,
6.62694427389891));
#147085=CARTESIAN_POINT('Ctrl Pts',(-5.81300774969049,-0.826237684531225,
6.73350551647852));
#147086=CARTESIAN_POINT('Ctrl Pts',(-5.84348544786606,-0.915473689913203,
6.77152999653492));
#147087=CARTESIAN_POINT('Ctrl Pts',(-5.87836203971057,-0.999999999954829,
6.81504656831974));
#147088=CARTESIAN_POINT('Origin',(1.11022302462516E-15,0.999999999999982,
2.22044604925031E-15));
#147089=CARTESIAN_POINT('Origin',(1.11022302462516E-15,-1.77635683940025E-14,
2.22044604925031E-15));
#147090=CARTESIAN_POINT('',(-5.336120511,-1.00000000000002,7.247469758));
#147091=CARTESIAN_POINT('',(-5.33612051,0.999999999999982,7.247469758));
#147092=CARTESIAN_POINT('Ctrl Pts',(-5.3361205102212,-1.00000000007198,
7.24746975847874));
#147093=CARTESIAN_POINT('Ctrl Pts',(-5.29058375025361,-0.888963444727199,
7.1900830269119));
#147094=CARTESIAN_POINT('Ctrl Pts',(-5.25266222949664,-0.769956469647752,
7.14228727279496));
#147095=CARTESIAN_POINT('Ctrl Pts',(-5.17095250443963,-0.424051722942908,
7.03929591826979));
#147096=CARTESIAN_POINT('Ctrl Pts',(-5.14607571334354,-0.18879105880776,
7.00793371972911));
#147097=CARTESIAN_POINT('Ctrl Pts',(-5.15376998852218,0.283921315901019,
7.01763317512498));
#147098=CARTESIAN_POINT('Ctrl Pts',(-5.18628392854453,0.516830885572041,
7.05862267723458));
#147099=CARTESIAN_POINT('Ctrl Pts',(-5.27116656029511,0.826237684454485,
7.16560944591632));
#147100=CARTESIAN_POINT('Ctrl Pts',(-5.30145576140191,0.915473689787588,
7.20378424732816));
#147101=CARTESIAN_POINT('Ctrl Pts',(-5.33612051010402,0.999999999786214,
7.24746975833107));
#147102=CARTESIAN_POINT('',(-5.243801419,-1.00000000000002,7.314543504));
#147103=CARTESIAN_POINT('Origin',(1.11022302462516E-15,-1.00000000000002,
2.22044604925031E-15));
#147104=CARTESIAN_POINT('',(-5.243801419,0.999999999999982,7.314543505));
#147105=CARTESIAN_POINT('Ctrl Pts',(-5.24380141936077,1.00000000025758,
7.31454350429201));
#147106=CARTESIAN_POINT('Ctrl Pts',(-5.20329502701867,0.888963444859877,
7.25350199664625));
#147107=CARTESIAN_POINT('Ctrl Pts',(-5.16955695795366,0.769956469717498,
7.20266678690975));
#147108=CARTESIAN_POINT('Ctrl Pts',(-5.09685605273471,0.424051722943015,
7.09313014161181));
#147109=CARTESIAN_POINT('Ctrl Pts',(-5.07471618065861,0.188791058807757,
7.05977945500723));
#147110=CARTESIAN_POINT('Ctrl Pts',(-5.08156324912865,-0.283921315901173,
7.07009444210697));
#147111=CARTESIAN_POINT('Ctrl Pts',(-5.11049922219243,-0.516830885572257,
7.113683489376));
#147112=CARTESIAN_POINT('Ctrl Pts',(-5.18601950998405,-0.826237684487118,
7.22747239912401));
#147113=CARTESIAN_POINT('Ctrl Pts',(-5.21296602575132,-0.915473689849885,
7.26807580361716));
#147114=CARTESIAN_POINT('Ctrl Pts',(-5.24380141922105,-0.999999999874601,
7.31454350408145));
#147115=CARTESIAN_POINT('Origin',(1.11022302462516E-15,0.999999999999982,
2.22044604925031E-15));
#147116=CARTESIAN_POINT('Origin',(1.11022302462516E-15,-1.77635683940025E-14,
2.22044604925031E-15));
#147117=CARTESIAN_POINT('',(-4.664980679,-1.00000000000002,7.69661973));
#147118=CARTESIAN_POINT('',(-4.664980679,0.999999999999982,7.69661973));
#147119=CARTESIAN_POINT('Ctrl Pts',(-4.6649806790278,-1.00000000012154,
7.69661972976142));
#147120=CARTESIAN_POINT('Ctrl Pts',(-4.62477134369037,-0.888963444769277,
7.6353821365611));
#147121=CARTESIAN_POINT('Ctrl Pts',(-4.59128686224838,-0.769956469681022,
7.58437953514422));
#147122=CARTESIAN_POINT('Ctrl Pts',(-4.51913815048226,-0.424051722956112,
7.47447839016348));
#147123=CARTESIAN_POINT('Ctrl Pts',(-4.49717279187257,-0.188791058808881,
7.44101250822753));
#147124=CARTESIAN_POINT('Ctrl Pts',(-4.50396663967298,0.283921315917288,
7.45136262598659));
#147125=CARTESIAN_POINT('Ctrl Pts',(-4.53267541744312,0.516830885595098,
7.49510164355728));
#147126=CARTESIAN_POINT('Ctrl Pts',(-4.60762611656943,0.826237684595678,
7.609266535536));
#147127=CARTESIAN_POINT('Ctrl Pts',(-4.6343714194336,0.915473690032038,
7.65000275956128));
#147128=CARTESIAN_POINT('Ctrl Pts',(-4.6649806790278,1.00000000012149,7.69661972976142));
#147129=CARTESIAN_POINT('',(-4.567020791,-1.00000000000002,7.755148038));
#147130=CARTESIAN_POINT('Origin',(1.11022302462516E-15,-1.00000000000002,
2.22044604925031E-15));
#147131=CARTESIAN_POINT('',(-4.56702079017615,1.00000000014985,7.75514803858119));
#147132=CARTESIAN_POINT('Ctrl Pts',(-4.56702079103465,1.0000000001046,7.7551480381945));
#147133=CARTESIAN_POINT('Ctrl Pts',(-4.53214918409692,0.888963444751377,
7.69072130073945));
#147134=CARTESIAN_POINT('Ctrl Pts',(-4.50310376766113,0.769956469661912,
7.63706648144992));
#147135=CARTESIAN_POINT('Ctrl Pts',(-4.44051432410009,0.42405172294464,
7.5214539396054));
#147136=CARTESIAN_POINT('Ctrl Pts',(-4.42145311313639,0.188791058807904,
7.48625291022913));
#147137=CARTESIAN_POINT('Ctrl Pts',(-4.42734798900763,-0.283921315903176,
7.49714013870893));
#147138=CARTESIAN_POINT('Ctrl Pts',(-4.45226018228089,-0.516830885575103,
7.54314750991512));
#147139=CARTESIAN_POINT('Ctrl Pts',(-4.5172764883787,-0.826237684515357,
7.66324792537743));
#147140=CARTESIAN_POINT('Ctrl Pts',(-4.5404748642876,-0.915473689900839,
7.7061033395637));
#147141=CARTESIAN_POINT('Ctrl Pts',(-4.56702079098469,-0.999999999945533,
7.75514803810219));
#147142=CARTESIAN_POINT('Origin',(1.11022302462516E-15,0.999999999999982,
2.22044604925031E-15));
#147143=CARTESIAN_POINT('Origin',(1.11022302462516E-15,-1.77635683940025E-14,
2.22044604925031E-15));
#147144=CARTESIAN_POINT('',(-3.956281164,-1.00000000000002,8.083801046));
#147145=CARTESIAN_POINT('',(-3.956281165,0.999999999999982,8.083801046));
#147146=CARTESIAN_POINT('Ctrl Pts',(-3.95628116468507,-1.00000000001549,
8.08380104560689));
#147147=CARTESIAN_POINT('Ctrl Pts',(-3.92172299585936,-0.888963444693512,
8.01920563994907));
#147148=CARTESIAN_POINT('Ctrl Pts',(-3.89294515105064,-0.769956469641267,
7.96540683425602));
#147149=CARTESIAN_POINT('Ctrl Pts',(-3.83093835147929,-0.424051722956145,
7.84948075832601));
#147150=CARTESIAN_POINT('Ctrl Pts',(-3.81206127747473,-0.188791058808899,
7.81418064062606));
#147151=CARTESIAN_POINT('Ctrl Pts',(-3.81789999783811,0.28392131591731,
7.82509808767561));
#147152=CARTESIAN_POINT('Ctrl Pts',(-3.84257246720139,0.516830885595139,
7.87123445981979));
#147153=CARTESIAN_POINT('Ctrl Pts',(-3.90698777483688,0.826237684636356,
7.99165828639558));
#147154=CARTESIAN_POINT('Ctrl Pts',(-3.92997384201674,0.915473690110029,
8.03462794884641));
#147155=CARTESIAN_POINT('Ctrl Pts',(-3.95628116475256,1.0000000002323,8.08380104573304));
#147156=CARTESIAN_POINT('',(-3.853469197,-1.00000000000002,8.133312679));
#147157=CARTESIAN_POINT('Origin',(1.11022302462516E-15,-1.00000000000002,
2.22044604925031E-15));
#147158=CARTESIAN_POINT('',(-3.853469197,0.999999999999982,8.13331268));
#147159=CARTESIAN_POINT('Ctrl Pts',(-3.85346919706807,1.0000000001062,8.13331267979544));
#147160=CARTESIAN_POINT('Ctrl Pts',(-3.82451314113869,0.888963444756583,
8.06601943872399));
#147161=CARTESIAN_POINT('Ctrl Pts',(-3.80039423388956,0.769956469671448,
8.00997700692796));
#147162=CARTESIAN_POINT('Ctrl Pts',(-3.74842018528738,0.424051722952648,
7.88921941276123));
#147163=CARTESIAN_POINT('Ctrl Pts',(-3.73259110507324,0.188791058808531,
7.85245145861415));
#147164=CARTESIAN_POINT('Ctrl Pts',(-3.73748632627966,-0.283921315913158,
7.86382327090975));
#147165=CARTESIAN_POINT('Ctrl Pts',(-3.758174161464,-0.51683088558922,7.91187854173883));
#147166=CARTESIAN_POINT('Ctrl Pts',(-3.81216301286461,-0.826237684430458,
8.0373234849023));
#147167=CARTESIAN_POINT('Ctrl Pts',(-3.83142646923125,-0.915473689721949,
8.08208586210271));
#147168=CARTESIAN_POINT('Ctrl Pts',(-3.85346919695796,-0.999999999683992,
8.13331267953955));
#147169=CARTESIAN_POINT('Origin',(1.11022302462516E-15,0.999999999999982,
2.22044604925031E-15));
#147170=CARTESIAN_POINT('Origin',(1.11022302462516E-15,-1.77635683940025E-14,
2.22044604925031E-15));
#147171=CARTESIAN_POINT('',(-3.215728,-1.00000000000002,8.405896349));
#147172=CARTESIAN_POINT('',(-3.215728,0.999999999999982,8.405896349));
#147173=CARTESIAN_POINT('Ctrl Pts',(-3.21572799910164,-1.00000000004898,
8.40589634930078));
#147174=CARTESIAN_POINT('Ctrl Pts',(-3.18709923874645,-0.888963444711017,
8.33846321539938));
#147175=CARTESIAN_POINT('Ctrl Pts',(-3.16325973277762,-0.769956469639689,
8.28230136177404));
#147176=CARTESIAN_POINT('Ctrl Pts',(-3.11189408755156,-0.424051722943413,
8.16128372353288));
#147177=CARTESIAN_POINT('Ctrl Pts',(-3.09625728521347,-0.188791058807823,
8.12443358587799));
#147178=CARTESIAN_POINT('Ctrl Pts',(-3.10109386820782,0.283921315901608,
8.13583046134637));
#147179=CARTESIAN_POINT('Ctrl Pts',(-3.12153138099901,0.516830885572894,
8.18399272510012));
#147180=CARTESIAN_POINT('Ctrl Pts',(-3.17489266307678,0.82623768455158,
8.30970590433158));
#147181=CARTESIAN_POINT('Ctrl Pts',(-3.19393442429636,0.915473689972812,
8.35456303867883));
#147182=CARTESIAN_POINT('Ctrl Pts',(-3.21572799910164,1.00000000004894,
8.40589634930078));
#147183=CARTESIAN_POINT('',(-3.108891736,-1.00000000000002,8.445992669));
#147184=CARTESIAN_POINT('Origin',(1.11022302462516E-15,-1.00000000000002,
2.22044604925031E-15));
#147185=CARTESIAN_POINT('',(-3.108891736,0.999999999999982,8.44599267));
#147186=CARTESIAN_POINT('Ctrl Pts',(-3.10889173624931,1.00000000023756,
8.44599266953942));
#147187=CARTESIAN_POINT('Ctrl Pts',(-3.08608436854417,0.888963444846536,
8.37637473037447));
#147188=CARTESIAN_POINT('Ctrl Pts',(-3.06708616180808,0.769956469712122,
8.31839590671147));
#147189=CARTESIAN_POINT('Ctrl Pts',(-3.0261459728075,0.424051722944941,
8.19346552927423));
#147190=CARTESIAN_POINT('Ctrl Pts',(-3.01367646984111,0.188791058807912,
8.15542668428226));
#147191=CARTESIAN_POINT('Ctrl Pts',(-3.01753262292282,-0.283921315903578,
8.16719152125183));
#147192=CARTESIAN_POINT('Ctrl Pts',(-3.03382953366587,-0.51683088557566,
8.21690777894712));
#147193=CARTESIAN_POINT('Ctrl Pts',(-3.07635624373367,-0.826237684462668,
8.34668724102495));
#147194=CARTESIAN_POINT('Ctrl Pts',(-3.09152968251005,-0.915473689799155,
8.39299618100886));
#147195=CARTESIAN_POINT('Ctrl Pts',(-3.10889173615958,-0.999999999800759,
8.44599266926553));
#147196=CARTESIAN_POINT('Origin',(1.11022302462516E-15,0.999999999999982,
2.22044604925031E-15));
#147197=CARTESIAN_POINT('Origin',(1.11022302462516E-15,-1.77635683940025E-14,
2.22044604925031E-15));
#147198=CARTESIAN_POINT('',(-2.449283685,-1.00000000000002,8.660312317));
#147199=CARTESIAN_POINT('',(-2.449283685,0.999999999999982,8.660312317));
#147200=CARTESIAN_POINT('Ctrl Pts',(-2.44928368492003,-0.999999999970374,
8.66031231707298));
#147201=CARTESIAN_POINT('Ctrl Pts',(-2.42681483511176,-0.888963444658655,
8.5905843868621));
#147202=CARTESIAN_POINT('Ctrl Pts',(-2.40810560977551,-0.769956469618574,
8.53251166751632));
#147203=CARTESIAN_POINT('Ctrl Pts',(-2.36779468507834,-0.424051722950929,
8.40737682975315));
#147204=CARTESIAN_POINT('Ctrl Pts',(-2.35552405280636,-0.188791058808435,
8.36927336775524));
#147205=CARTESIAN_POINT('Ctrl Pts',(-2.35931955709161,0.283921315910924,
8.3810579107145));
#147206=CARTESIAN_POINT('Ctrl Pts',(-2.37535756239453,0.516830885586079,
8.4308582918873));
#147207=CARTESIAN_POINT('Ctrl Pts',(-2.41723518504276,0.826237684533093,
8.56084865527989));
#147208=CARTESIAN_POINT('Ctrl Pts',(-2.4321793271706,0.915473689922331,
8.6072320982976));
#147209=CARTESIAN_POINT('Ctrl Pts',(-2.44928368492003,0.999999999970338,
8.66031231707298));
#147210=CARTESIAN_POINT('',(-2.339283306,-1.00000000000002,8.690670493));
#147211=CARTESIAN_POINT('Origin',(1.11022302462516E-15,-1.00000000000002,
2.22044604925031E-15));
#147212=CARTESIAN_POINT('',(-2.339283305,0.999999999999982,8.690670493));
#147213=CARTESIAN_POINT('Ctrl Pts',(-2.33928330561053,1.00000000001403,
8.69067049283724));
#147214=CARTESIAN_POINT('Ctrl Pts',(-2.322808257611,0.888963444688627,8.61928837841982));
#147215=CARTESIAN_POINT('Ctrl Pts',(-2.30908371374843,0.769956469632263,
8.55983997438751));
#147216=CARTESIAN_POINT('Ctrl Pts',(-2.27950701057719,0.424051722948508,
8.4317426797122));
#147217=CARTESIAN_POINT('Ctrl Pts',(-2.27049748192908,0.188791058808201,
8.39273921030103));
#147218=CARTESIAN_POINT('Ctrl Pts',(-2.27328351942049,-0.283921315908011,
8.40480234839289));
#147219=CARTESIAN_POINT('Ctrl Pts',(-2.28505829262577,-0.516830885581936,
8.45577930686427));
#147220=CARTESIAN_POINT('Ctrl Pts',(-2.31578046142091,-0.826237684583821,
8.58884837992318));
#147221=CARTESIAN_POINT('Ctrl Pts',(-2.32674171504669,-0.91547369002434,
8.63633103035859));
#147222=CARTESIAN_POINT('Ctrl Pts',(-2.33928330562587,-1.00000000011744,
8.6906704929037));
#147223=CARTESIAN_POINT('Origin',(1.11022302462516E-15,0.999999999999982,
2.22044604925031E-15));
#147224=CARTESIAN_POINT('Origin',(1.11022302462516E-15,-1.77635683940025E-14,
2.22044604925031E-15));
#147225=CARTESIAN_POINT('',(-1.663119178,-1.00000000000002,8.845000543));
#147226=CARTESIAN_POINT('',(-1.663119178,0.999999999999982,8.845000543));
#147227=CARTESIAN_POINT('Ctrl Pts',(-1.66311917835389,-1.00000000017415,
8.84500054264958));
#147228=CARTESIAN_POINT('Ctrl Pts',(-1.64699114496605,-0.888963444802729,
8.77353922436293));
#147229=CARTESIAN_POINT('Ctrl Pts',(-1.6335628358678,-0.769956469691642,
8.7140232066417));
#147230=CARTESIAN_POINT('Ctrl Pts',(-1.60463119142804,-0.424051722947916,
8.58577868149686));
#147231=CARTESIAN_POINT('Ctrl Pts',(-1.5958255251009,-0.188791058808179,
8.54672868184127));
#147232=CARTESIAN_POINT('Ctrl Pts',(-1.59854939151922,0.283921315907216,
8.55880601007475));
#147233=CARTESIAN_POINT('Ctrl Pts',(-1.61005876079405,0.516830885580825,
8.6098435452613));
#147234=CARTESIAN_POINT('Ctrl Pts',(-1.64011555016048,0.826237684603746,
8.7430644868424));
#147235=CARTESIAN_POINT('Ctrl Pts',(-1.65084175181584,0.915473690063816,
8.79060078636947));
#147236=CARTESIAN_POINT('Ctrl Pts',(-1.66311917835389,1.00000000017411,
8.84500054264958));
#147237=CARTESIAN_POINT('',(-1.550840341,-1.00000000000002,8.865376147));
#147238=CARTESIAN_POINT('Origin',(1.11022302462516E-15,-1.00000000000002,
2.22044604925031E-15));
#147239=CARTESIAN_POINT('',(-1.550840341,0.999999999999982,8.865376147));
#147240=CARTESIAN_POINT('Ctrl Pts',(-1.55084034140624,0.999999999808246,
8.86537614723733));
#147241=CARTESIAN_POINT('Ctrl Pts',(-1.54083026051303,0.88896344454227,
8.7928045843712));
#147242=CARTESIAN_POINT('Ctrl Pts',(-1.53248988148326,0.769956469556594,
8.73236524355607));
#147243=CARTESIAN_POINT('Ctrl Pts',(-1.51451479838375,0.424051722949868,
8.60213239572782));
#147244=CARTESIAN_POINT('Ctrl Pts',(-1.50903778348876,0.188791058808319,
8.56247833489648));
#147245=CARTESIAN_POINT('Ctrl Pts',(-1.51073127385161,-0.283921315909671,
8.57474264881631));
#147246=CARTESIAN_POINT('Ctrl Pts',(-1.51788910595866,-0.516830885584286,
8.62656987157201));
#147247=CARTESIAN_POINT('Ctrl Pts',(-1.53655937659347,-0.82623768447221,
8.76185716159184));
#147248=CARTESIAN_POINT('Ctrl Pts',(-1.54322019145936,-0.915473689807616,
8.81013121996666));
#147249=CARTESIAN_POINT('Ctrl Pts',(-1.55084034140624,-0.999999999808279,
8.86537614723733));
#147250=CARTESIAN_POINT('Origin',(1.11022302462516E-15,0.999999999999982,
2.22044604925031E-15));
#147251=CARTESIAN_POINT('Origin',(1.11022302462516E-15,-1.77635683940025E-14,
2.22044604925031E-15));
#147252=CARTESIAN_POINT('',(-0.863564212999999,-1.00000000000002,8.958474025));
#147253=CARTESIAN_POINT('',(-0.863564212999999,0.999999999999982,8.958474025));
#147254=CARTESIAN_POINT('Ctrl Pts',(-0.863564213524501,-1.00000000018892,
8.95847402464142));
#147255=CARTESIAN_POINT('Ctrl Pts',(-0.853906850043781,-0.888963444813406,
8.88585468284159));
#147256=CARTESIAN_POINT('Ctrl Pts',(-0.845867574068782,-0.769956469697448,
8.82537455475955));
#147257=CARTESIAN_POINT('Ctrl Pts',(-0.828548150532178,-0.42405172294816,
8.69505289175401));
#147258=CARTESIAN_POINT('Ctrl Pts',(-0.823278348211893,-0.188791058808215,
8.65537076207235));
#147259=CARTESIAN_POINT('Ctrl Pts',(-0.824908645788194,0.283921315907471,
8.66764363603641));
#147260=CARTESIAN_POINT('Ctrl Pts',(-0.83179671234216,0.516830885581191,
8.71950740101902));
#147261=CARTESIAN_POINT('Ctrl Pts',(-0.84979066877245,0.82623768460948,
8.8548863040852));
#147262=CARTESIAN_POINT('Ctrl Pts',(-0.856212568854875,0.915473690074359,
8.90319272575272));
#147263=CARTESIAN_POINT('Ctrl Pts',(-0.863564213524501,1.00000000018888,
8.95847402464141));
#147264=CARTESIAN_POINT('',(-0.749910922999999,-1.00000000000002,8.968703006));
#147265=CARTESIAN_POINT('Origin',(1.11022302462516E-15,-1.00000000000002,
2.22044604925031E-15));
#147266=CARTESIAN_POINT('',(-0.749910922999999,0.999999999999982,8.968703006));
#147267=CARTESIAN_POINT('Ctrl Pts',(-0.749910923421741,1.0000000000954,
8.96870300583526));
#147268=CARTESIAN_POINT('Ctrl Pts',(-0.746446404937193,0.888963444745311,
8.89552629792414));
#147269=CARTESIAN_POINT('Ctrl Pts',(-0.743557342583254,0.769956469659581,
8.83458264224674));
#147270=CARTESIAN_POINT('Ctrl Pts',(-0.737328604408769,0.424051722945646,
8.70326279950606));
#147271=CARTESIAN_POINT('Ctrl Pts',(-0.73542820098917,0.188791058807986,
8.66327741843499));
#147272=CARTESIAN_POINT('Ctrl Pts',(-0.736015509228913,-0.283921315904419,
8.67564416313782));
#147273=CARTESIAN_POINT('Ctrl Pts',(-0.738498769557774,-0.516830885576862,
8.72790436785554));
#147274=CARTESIAN_POINT('Ctrl Pts',(-0.744966819940244,-0.826237684571763,
8.86432062122608));
#147275=CARTESIAN_POINT('Ctrl Pts',(-0.747273567077168,-0.91547369000699,
8.91299741334237));
#147276=CARTESIAN_POINT('Ctrl Pts',(-0.749910923421741,-1.00000000009543,
8.96870300583526));
#147277=CARTESIAN_POINT('Origin',(1.11022302462516E-15,0.999999999999982,
2.22044604925031E-15));
#147278=CARTESIAN_POINT('Origin',(1.11022302462516E-15,-1.77635683940025E-14,
2.22044604925031E-15));
#147279=CARTESIAN_POINT('',(-0.057056338,-1.00000000000002,8.999819141));
#147280=CARTESIAN_POINT('',(-0.057056338,0.999999999999982,8.999819141));
#147281=CARTESIAN_POINT('Ctrl Pts',(-0.0570563383389178,-0.999999999933198,
8.99981914108698));
#147282=CARTESIAN_POINT('Ctrl Pts',(-0.0539474002202254,-0.88896344463397,
8.92662646409639));
#147283=CARTESIAN_POINT('Ctrl Pts',(-0.0513618849266572,-0.769956469608777,
8.86566917614544));
#147284=CARTESIAN_POINT('Ctrl Pts',(-0.0457941281782648,-0.424051722954678,
8.73431964871832));
#147285=CARTESIAN_POINT('Ctrl Pts',(-0.0441026192351823,-0.188791058808769,
8.69432488618504));
#147286=CARTESIAN_POINT('Ctrl Pts',(-0.0446262217656057,0.283921315915507,
8.70669449191623));
#147287=CARTESIAN_POINT('Ctrl Pts',(-0.0468375269099042,0.516830885592579,
8.75896691015616));
#147288=CARTESIAN_POINT('Ctrl Pts',(-0.0526237735737156,0.82623768452456,
8.89541378333879));
#147289=CARTESIAN_POINT('Ctrl Pts',(-0.0546896666910911,0.915473689898557,
8.9441013921808));
#147290=CARTESIAN_POINT('Ctrl Pts',(-0.0570563383389176,0.999999999933163,
8.99981914108698));
#147291=CARTESIAN_POINT('',(0.0570563369999999,-1.00000000000002,8.999819141));
#147292=CARTESIAN_POINT('Origin',(1.11022302462516E-15,-1.00000000000002,
2.22044604925031E-15));
#147293=CARTESIAN_POINT('',(0.0570563369999999,0.999999999999982,8.999819141));
#147294=CARTESIAN_POINT('Ctrl Pts',(0.0570563367490446,0.999999999940043,
8.99981914110159));
#147295=CARTESIAN_POINT('Ctrl Pts',(0.0539473986136925,0.888963444636815,
8.92662646410728));
#147296=CARTESIAN_POINT('Ctrl Pts',(0.0513618833063579,0.769956469606838,
8.86566917615349));
#147297=CARTESIAN_POINT('Ctrl Pts',(0.0457941265286543,0.424051722950573,
8.73431964872651));
#147298=CARTESIAN_POINT('Ctrl Pts',(0.0441026175767656,0.188791058808352,
8.69432488619386));
#147299=CARTESIAN_POINT('Ctrl Pts',(0.0446262201098957,-0.2839213159106,
8.70669449192419));
#147300=CARTESIAN_POINT('Ctrl Pts',(0.0468375252657094,-0.516830885585594,
8.75896691016323));
#147301=CARTESIAN_POINT('Ctrl Pts',(0.0526237719600633,-0.826237684521612,
8.89541378334644));
#147302=CARTESIAN_POINT('Ctrl Pts',(0.0546896650884921,-0.91547368990086,
8.94410139219155));
#147303=CARTESIAN_POINT('Ctrl Pts',(0.0570563367490447,-0.999999999940079,
8.9998191411016));
#147304=CARTESIAN_POINT('Origin',(1.11022302462516E-15,0.999999999999982,
2.22044604925031E-15));
#147305=CARTESIAN_POINT('Origin',(1.11022302462516E-15,-1.77635683940025E-14,
2.22044604925031E-15));
#147306=CARTESIAN_POINT('',(0.749910923000001,-1.00000000000002,8.968703006));
#147307=CARTESIAN_POINT('',(0.749910923000001,0.999999999999982,8.968703006));
#147308=CARTESIAN_POINT('Ctrl Pts',(0.749910923031046,-1.00000000008893,
8.96870300586362));
#147309=CARTESIAN_POINT('Ctrl Pts',(0.746446404541417,-0.888963444741279,
8.89552629795535));
#147310=CARTESIAN_POINT('Ctrl Pts',(0.743557342183267,-0.769956469658455,
8.83458264228014));
#147311=CARTESIAN_POINT('Ctrl Pts',(0.737328603999575,-0.424051722946827,
8.70326279954085));
#147312=CARTESIAN_POINT('Ctrl Pts',(0.735428200577185,-0.188791058808123,
8.66327741846986));
#147313=CARTESIAN_POINT('Ctrl Pts',(0.736015508817804,0.283921315905779,
8.67564416317285));
#147314=CARTESIAN_POINT('Ctrl Pts',(0.73849876915032,0.516830885578806,
8.72790436789049));
#147315=CARTESIAN_POINT('Ctrl Pts',(0.74496681954236,0.826237684570912,
8.86432062125932));
#147316=CARTESIAN_POINT('Ctrl Pts',(0.747273566682631,0.91547369000311,
8.91299741337342));
#147317=CARTESIAN_POINT('Ctrl Pts',(0.749910923031046,1.00000000008889,
8.96870300586362));
#147318=CARTESIAN_POINT('',(0.863564212000001,-1.00000000000002,8.958474025));
#147319=CARTESIAN_POINT('Origin',(1.11022302462516E-15,-1.00000000000002,
2.22044604925031E-15));
#147320=CARTESIAN_POINT('',(0.863564213,0.999999999999982,8.958474025));
#147321=CARTESIAN_POINT('Ctrl Pts',(0.863564212376334,1.00000000020806,
8.95847402476479));
#147322=CARTESIAN_POINT('Ctrl Pts',(0.85390684889901,0.888963444826714,
8.88585468295841));
#147323=CARTESIAN_POINT('Ctrl Pts',(0.845867572926911,0.769956469703821,
8.82537455487133));
#147324=CARTESIAN_POINT('Ctrl Pts',(0.828548149397508,0.424051722947431,
8.69505289186206));
#147325=CARTESIAN_POINT('Ctrl Pts',(0.823278347079537,0.188791058808132,
8.65537076218013));
#147326=CARTESIAN_POINT('Ctrl Pts',(0.824908644655106,-0.283921315906622,
8.66764363614415));
#147327=CARTESIAN_POINT('Ctrl Pts',(0.83179671120604,-0.516830885579978,
8.71950740112709));
#147328=CARTESIAN_POINT('Ctrl Pts',(0.849790667627614,-0.826237684593335,
8.8548863041878));
#147329=CARTESIAN_POINT('Ctrl Pts',(0.856212567706076,-0.915473690044782,
8.90319272584691));
#147330=CARTESIAN_POINT('Ctrl Pts',(0.863564212371063,-1.00000000014749,
8.95847402472516));
#147331=CARTESIAN_POINT('Origin',(1.11022302462516E-15,0.999999999999982,
2.22044604925031E-15));
#147332=CARTESIAN_POINT('Origin',(1.11022302462516E-15,-1.77635683940025E-14,
2.22044604925031E-15));
#147333=CARTESIAN_POINT('',(1.550840341,-1.00000000000002,8.865376147));
#147334=CARTESIAN_POINT('',(1.550840341,0.999999999999982,8.865376147));
#147335=CARTESIAN_POINT('Ctrl Pts',(1.55084034103818,-0.999999999802086,
8.86537614729757));
#147336=CARTESIAN_POINT('Ctrl Pts',(1.54083026013964,-0.888963444538492,
8.79280458443474));
#147337=CARTESIAN_POINT('Ctrl Pts',(1.53248988110544,-0.769956469555649,
8.73236524362217));
#147338=CARTESIAN_POINT('Ctrl Pts',(1.51451479799596,-0.424051722951098,
8.60213239579622));
#147339=CARTESIAN_POINT('Ctrl Pts',(1.50903778309792,-0.188791058808459,
8.56247833496524));
#147340=CARTESIAN_POINT('Ctrl Pts',(1.51073127346174,0.283921315911105,
8.57474264888516));
#147341=CARTESIAN_POINT('Ctrl Pts',(1.51788910557278,0.516830885586341,
8.62656987164042));
#147342=CARTESIAN_POINT('Ctrl Pts',(1.53655937621794,0.826237684471544,
8.76185716165758));
#147343=CARTESIAN_POINT('Ctrl Pts',(1.54322019108732,0.91547368980399,8.81013122002992));
#147344=CARTESIAN_POINT('Ctrl Pts',(1.55084034103818,0.99999999980205,8.86537614729757));
#147345=CARTESIAN_POINT('',(1.663119178,-1.00000000000002,8.845000543));
#147346=CARTESIAN_POINT('Origin',(1.11022302462516E-15,-1.00000000000002,
2.22044604925031E-15));
#147347=CARTESIAN_POINT('',(1.663119178,0.999999999999982,8.845000543));
#147348=CARTESIAN_POINT('Ctrl Pts',(1.66311917779156,1.00000000018363,8.84500054276169));
#147349=CARTESIAN_POINT('Ctrl Pts',(1.64699114441794,0.888963444810215,
8.77353922446985));
#147350=CARTESIAN_POINT('Ctrl Pts',(1.63356283533152,0.769956469696762,
8.71402320674444));
#147351=CARTESIAN_POINT('Ctrl Pts',(1.60463119091762,0.424051722949316,
8.58577868159241));
#147352=CARTESIAN_POINT('Ctrl Pts',(1.5958255245984,0.188791058808291,8.54672868193495));
#147353=CARTESIAN_POINT('Ctrl Pts',(1.59854939101432,-0.28392131590896,
8.55880601016923));
#147354=CARTESIAN_POINT('Ctrl Pts',(1.61005876027881,-0.516830885583296,
8.60984354535825));
#147355=CARTESIAN_POINT('Ctrl Pts',(1.64011554961833,-0.826237684609203,
8.74306448694674));
#147356=CARTESIAN_POINT('Ctrl Pts',(1.65084175126428,-0.915473690071451,
8.79060078647738));
#147357=CARTESIAN_POINT('Ctrl Pts',(1.66311917779156,-1.00000000018366,
8.84500054276169));
#147358=CARTESIAN_POINT('Origin',(1.11022302462516E-15,0.999999999999982,
2.22044604925031E-15));
#147359=CARTESIAN_POINT('Origin',(1.11022302462516E-15,-1.77635683940025E-14,
2.22044604925031E-15));
#147360=CARTESIAN_POINT('',(2.339283305,-1.00000000000002,8.690670493));
#147361=CARTESIAN_POINT('',(2.339283305,0.999999999999982,8.690670493));
#147362=CARTESIAN_POINT('Ctrl Pts',(2.33928330447186,-0.999999999994545,
8.6906704931304));
#147363=CARTESIAN_POINT('Ctrl Pts',(2.32280825646114,-0.888963444676295,
8.61928837872337));
#147364=CARTESIAN_POINT('Ctrl Pts',(2.30908371258922,-0.769956469628457,
8.55983997469919));
#147365=CARTESIAN_POINT('Ctrl Pts',(2.2795070093957,-0.424051722951687,
8.43174268003198));
#147366=CARTESIAN_POINT('Ctrl Pts',(2.27049748074064,-0.188791058808529,
8.39273921062222));
#147367=CARTESIAN_POINT('Ctrl Pts',(2.27328351823432,0.283921315911797,
8.40480234871414));
#147368=CARTESIAN_POINT('Ctrl Pts',(2.2850582914487,0.51683088558733,8.45577930718374));
#147369=CARTESIAN_POINT('Ctrl Pts',(2.31578046026309,0.826237684542946,
8.58884838021717));
#147370=CARTESIAN_POINT('Ctrl Pts',(2.32674171389092,0.915473689939803,
8.63633103062244));
#147371=CARTESIAN_POINT('Ctrl Pts',(2.33928330447186,0.99999999999451,8.6906704931304));
#147372=CARTESIAN_POINT('',(2.449283685,-1.00000000000002,8.660312317));
#147373=CARTESIAN_POINT('Origin',(1.11022302462516E-15,-1.00000000000002,
2.22044604925031E-15));
#147374=CARTESIAN_POINT('',(2.449283685,0.999999999999982,8.660312317));
#147375=CARTESIAN_POINT('Ctrl Pts',(2.44928368526842,0.999999999964307,
8.66031231697032));
#147376=CARTESIAN_POINT('Ctrl Pts',(2.42681483546961,0.888963444655136,
8.59058438675928));
#147377=CARTESIAN_POINT('Ctrl Pts',(2.40810561014116,0.769956469618104,
8.53251166741322));
#147378=CARTESIAN_POINT('Ctrl Pts',(2.36779468545961,0.424051722952564,
8.40737682964597));
#147379=CARTESIAN_POINT('Ctrl Pts',(2.35552405319223,0.188791058808564,
8.36927336764647));
#147380=CARTESIAN_POINT('Ctrl Pts',(2.35931955747614,-0.283921315912966,
8.38105791060647));
#147381=CARTESIAN_POINT('Ctrl Pts',(2.37535756277304,-0.516830885588967,
8.43085829178138));
#147382=CARTESIAN_POINT('Ctrl Pts',(2.41723518540491,-0.826237684533161,
8.5608486551779));
#147383=CARTESIAN_POINT('Ctrl Pts',(2.43217932752638,-0.915473689919173,
8.60723209819538));
#147384=CARTESIAN_POINT('Ctrl Pts',(2.44928368526842,-0.999999999964343,
8.66031231697032));
#147385=CARTESIAN_POINT('Origin',(1.11022302462516E-15,0.999999999999982,
2.22044604925031E-15));
#147386=CARTESIAN_POINT('Origin',(1.11022302462516E-15,-1.77635683940025E-14,
2.22044604925031E-15));
#147387=CARTESIAN_POINT('',(3.108891735,-1.00000000000002,8.44599267));
#147388=CARTESIAN_POINT('',(3.108891735,0.999999999999982,8.44599267));
#147389=CARTESIAN_POINT('Ctrl Pts',(3.10889173544937,-1.0000000000809,8.44599266972378));
#147390=CARTESIAN_POINT('Ctrl Pts',(3.08608436775726,-0.888963444735186,
8.37637473060366));
#147391=CARTESIAN_POINT('Ctrl Pts',(3.06708616103102,-0.769956469654649,
8.31839590697489));
#147392=CARTESIAN_POINT('Ctrl Pts',(3.02614597203478,-0.424051722946102,
8.19346552955976));
#147393=CARTESIAN_POINT('Ctrl Pts',(3.0136764690676,-0.188791058808042,
8.15542668456797));
#147394=CARTESIAN_POINT('Ctrl Pts',(3.01753262214962,0.283921315904921,
8.16719152153767));
#147395=CARTESIAN_POINT('Ctrl Pts',(3.03382953289371,0.516830885577575,
8.21690777923271));
#147396=CARTESIAN_POINT('Ctrl Pts',(3.07635624297832,0.826237684567004,
8.34668724135259));
#147397=CARTESIAN_POINT('Ctrl Pts',(3.0915296817749,0.915473689997012,8.39299618139483));
#147398=CARTESIAN_POINT('Ctrl Pts',(3.10889173544937,1.00000000008087,8.44599266972378));
#147399=CARTESIAN_POINT('',(3.215728,-1.00000000000002,8.405896349));
#147400=CARTESIAN_POINT('Origin',(1.11022302462516E-15,-1.00000000000002,
2.22044604925031E-15));
#147401=CARTESIAN_POINT('',(3.215728,0.999999999999982,8.405896349));
#147402=CARTESIAN_POINT('Ctrl Pts',(3.21572799949971,1.00000000004184,8.40589634914348));
#147403=CARTESIAN_POINT('Ctrl Pts',(3.1870992391518,0.888963444706611,8.33846321524216));
#147404=CARTESIAN_POINT('Ctrl Pts',(3.16325973318893,0.769956469638538,
8.28230136161672));
#147405=CARTESIAN_POINT('Ctrl Pts',(3.11189408797419,0.424051722944791,
8.16128372337191));
#147406=CARTESIAN_POINT('Ctrl Pts',(3.09625728563936,0.188791058807925,
8.12443358571553));
#147407=CARTESIAN_POINT('Ctrl Pts',(3.10109386863279,-0.283921315903338,
8.13583046118458));
#147408=CARTESIAN_POINT('Ctrl Pts',(3.12153138141972,-0.516830885575335,
8.18399272494027));
#147409=CARTESIAN_POINT('Ctrl Pts',(3.17489266348559,-0.826237684550909,
8.30970590417526));
#147410=CARTESIAN_POINT('Ctrl Pts',(3.19393442470021,-0.915473689968736,
8.35456303852214));
#147411=CARTESIAN_POINT('Ctrl Pts',(3.21572799949971,-1.00000000004187,
8.40589634914348));
#147412=CARTESIAN_POINT('Origin',(1.11022302462516E-15,0.999999999999982,
2.22044604925031E-15));
#147413=CARTESIAN_POINT('Origin',(1.11022302462516E-15,-1.77635683940025E-14,
2.22044604925031E-15));
#147414=CARTESIAN_POINT('',(3.85346919675118,-0.999999999914645,8.13331268017501));
#147415=CARTESIAN_POINT('',(3.853469196,0.999999999999982,8.13331268));
#147416=CARTESIAN_POINT('Ctrl Pts',(3.85346919578197,-1.00000000005208,
8.13331268036528));
#147417=CARTESIAN_POINT('Ctrl Pts',(3.82451313984361,-0.888963444719939,
8.06601943931758));
#147418=CARTESIAN_POINT('Ctrl Pts',(3.8003942325866,-0.76995646965561,8.00997700754015));
#147419=CARTESIAN_POINT('Ctrl Pts',(3.74842018395873,-0.424051722956707,
7.88921941339301));
#147420=CARTESIAN_POINT('Ctrl Pts',(3.73259110373581,-0.188791058808946,
7.85245145924944));
#147421=CARTESIAN_POINT('Ctrl Pts',(3.73748632494522,0.283921315918004,
7.86382327154455));
#147422=CARTESIAN_POINT('Ctrl Pts',(3.75817416014108,0.51683088559612,7.91187854236911));
#147423=CARTESIAN_POINT('Ctrl Pts',(3.81216301158527,0.826237684515584,
8.03732348555132));
#147424=CARTESIAN_POINT('Ctrl Pts',(3.83142646798092,0.91547368987732,8.08208586278962));
#147425=CARTESIAN_POINT('Ctrl Pts',(3.85346919574262,0.999999999901147,
8.13331268027382));
#147426=CARTESIAN_POINT('',(3.956281164,-1.00000000000002,8.083801046));
#147427=CARTESIAN_POINT('Origin',(1.11022302462516E-15,-1.00000000000002,
2.22044604925031E-15));
#147428=CARTESIAN_POINT('',(3.956281164,0.999999999999982,8.083801046));
#147429=CARTESIAN_POINT('Ctrl Pts',(3.95628116427791,1.00000000002302,8.08380104581171));
#147430=CARTESIAN_POINT('Ctrl Pts',(3.92172299544629,0.88896344469827,8.01920564015371));
#147431=CARTESIAN_POINT('Ctrl Pts',(3.89294515063276,0.76995646964272,7.96540683446068));
#147432=CARTESIAN_POINT('Ctrl Pts',(3.83093835105285,0.424051722954895,
7.849480758534));
#147433=CARTESIAN_POINT('Ctrl Pts',(3.8120612770459,0.188791058808754,7.8141806408354));
#147434=CARTESIAN_POINT('Ctrl Pts',(3.81789999740993,-0.28392131591586,
7.82509808788435));
#147435=CARTESIAN_POINT('Ctrl Pts',(3.84257246677632,-0.516830885593063,
7.87123446002672));
#147436=CARTESIAN_POINT('Ctrl Pts',(3.9069877744043,-0.826237684557924,
7.99165828656834));
#147437=CARTESIAN_POINT('Ctrl Pts',(3.92997384156548,-0.915473689961999,
8.03462794897708));
#147438=CARTESIAN_POINT('Ctrl Pts',(3.95628116427791,-1.00000000002306,
8.08380104581171));
#147439=CARTESIAN_POINT('Origin',(1.11022302462516E-15,0.999999999999982,
2.22044604925031E-15));
#147440=CARTESIAN_POINT('Origin',(1.11022302462516E-15,-1.77635683940025E-14,
2.22044604925031E-15));
#147441=CARTESIAN_POINT('',(4.56702079,-1.00000000000002,7.755148038));
#147442=CARTESIAN_POINT('',(4.567020791,0.999999999999982,7.755148038));
#147443=CARTESIAN_POINT('Ctrl Pts',(4.56702079072311,-0.999999999723031,
7.75514803808598));
#147444=CARTESIAN_POINT('Ctrl Pts',(4.53214918384362,-0.888963444478469,
7.69072130072636));
#147445=CARTESIAN_POINT('Ctrl Pts',(4.50310376745261,-0.769956469518223,
7.63706648150941));
#147446=CARTESIAN_POINT('Ctrl Pts',(4.44051432392658,-0.424051722944125,
7.52145393970777));
#147447=CARTESIAN_POINT('Ctrl Pts',(4.42145311296569,-0.188791058807886,
7.48625291033002));
#147448=CARTESIAN_POINT('Ctrl Pts',(4.42734798883602,0.283921315902461,
7.49714013881019));
#147449=CARTESIAN_POINT('Ctrl Pts',(4.45226018210562,0.516830885574096,
7.54314751001828));
#147450=CARTESIAN_POINT('Ctrl Pts',(4.51727648819371,0.82623768451322,7.66324792548531));
#147451=CARTESIAN_POINT('Ctrl Pts',(4.54047486409896,0.915473689897855,
7.70610333967294));
#147452=CARTESIAN_POINT('Ctrl Pts',(4.56702079079182,0.999999999941805,
7.75514803821294));
#147453=CARTESIAN_POINT('',(4.664980679,-1.00000000000002,7.69661973));
#147454=CARTESIAN_POINT('Origin',(1.11022302462516E-15,-1.00000000000002,
2.22044604925031E-15));
#147455=CARTESIAN_POINT('',(4.664980678,0.999999999999982,7.69661973));
#147456=CARTESIAN_POINT('Ctrl Pts',(4.66498067874573,0.999999999872922,
7.69661972974073));
#147457=CARTESIAN_POINT('Ctrl Pts',(4.62477134343723,0.888963444590633,
7.63538213660728));
#147458=CARTESIAN_POINT('Ctrl Pts',(4.59128686201659,0.769956469585573,
7.58437953524182));
#147459=CARTESIAN_POINT('Ctrl Pts',(4.51913815025123,0.424051722954107,
7.47447839030291));
#147460=CARTESIAN_POINT('Ctrl Pts',(4.49717279163596,0.188791058808661,
7.44101250837075));
#147461=CARTESIAN_POINT('Ctrl Pts',(4.50396663943793,-0.28392131591495,
7.45136262612837));
#147462=CARTESIAN_POINT('Ctrl Pts',(4.53267541721536,-0.516830885591761,
7.49510164369408));
#147463=CARTESIAN_POINT('Ctrl Pts',(4.6076261163616,-0.826237684594402,
7.60926653566084));
#147464=CARTESIAN_POINT('Ctrl Pts',(4.63437141923369,-0.915473690033447,
7.6500027596831));
#147465=CARTESIAN_POINT('Ctrl Pts',(4.66498067883709,-1.00000000012526,
7.69661972987988));
#147466=CARTESIAN_POINT('Origin',(1.11022302462516E-15,0.999999999999982,
2.22044604925031E-15));
#147467=CARTESIAN_POINT('Origin',(1.11022302462516E-15,-1.77635683940025E-14,
2.22044604925031E-15));
#147468=CARTESIAN_POINT('',(5.243801418,-1.00000000000002,7.314543505));
#147469=CARTESIAN_POINT('',(5.243801418,0.999999999999982,7.314543505));
#147470=CARTESIAN_POINT('Ctrl Pts',(5.24380141829551,-0.999999999983744,
7.31454350483351));
#147471=CARTESIAN_POINT('Ctrl Pts',(5.20329502600419,-0.888963444664367,
7.25350199725071));
#147472=CARTESIAN_POINT('Ctrl Pts',(5.16955695697835,-0.769956469615145,
7.20266678756194));
#147473=CARTESIAN_POINT('Ctrl Pts',(5.09685605179224,-0.424051722943348,
7.09313014228908));
#147474=CARTESIAN_POINT('Ctrl Pts',(5.07471617971955,-0.188791058807811,
7.05977945568221));
#147475=CARTESIAN_POINT('Ctrl Pts',(5.08156324818856,0.283921315901524,
7.0700944427827));
#147476=CARTESIAN_POINT('Ctrl Pts',(5.11049922124789,0.516830885572765,
7.11368349005473));
#147477=CARTESIAN_POINT('Ctrl Pts',(5.18601950903758,0.826237684527554,
7.22747239982517));
#147478=CARTESIAN_POINT('Ctrl Pts',(5.21296602481403,0.915473689926858,
7.26807580434118));
#147479=CARTESIAN_POINT('Ctrl Pts',(5.24380141829551,0.999999999983706,
7.31454350483351));
#147480=CARTESIAN_POINT('',(5.336120511,-1.00000000000002,7.247469758));
#147481=CARTESIAN_POINT('Origin',(1.11022302462516E-15,-1.00000000000002,
2.22044604925031E-15));
#147482=CARTESIAN_POINT('',(5.336120511,0.999999999999982,7.247469758));
#147483=CARTESIAN_POINT('Ctrl Pts',(5.3361205105636,1.00000000006483,7.24746975822081));
#147484=CARTESIAN_POINT('Ctrl Pts',(5.29058375060566,0.888963444722995,
7.19008302665037));
#147485=CARTESIAN_POINT('Ctrl Pts',(5.25266222985656,0.769956469647073,
7.1422872725303));
#147486=CARTESIAN_POINT('Ctrl Pts',(5.17095250481386,0.424051722944686,
7.03929591799513));
#147487=CARTESIAN_POINT('Ctrl Pts',(5.14607571372183,0.188791058807888,
7.0079337194511));
#147488=CARTESIAN_POINT('Ctrl Pts',(5.1537699888994,-0.283921315903273,
7.01763317484824));
#147489=CARTESIAN_POINT('Ctrl Pts',(5.18628392891646,-0.51683088557523,
7.05862267696227));
#147490=CARTESIAN_POINT('Ctrl Pts',(5.27116656068068,-0.826237684559263,
7.16560944569038));
#147491=CARTESIAN_POINT('Ctrl Pts',(5.30145576182033,-0.915473689984878,
7.20378424715405));
#147492=CARTESIAN_POINT('Ctrl Pts',(5.3361205105636,-1.00000000006487,7.24746975822082));
#147493=CARTESIAN_POINT('Origin',(1.11022302462516E-15,0.999999999999982,
2.22044604925031E-15));
#147494=CARTESIAN_POINT('Origin',(1.11022302462516E-15,-1.77635683940025E-14,
2.22044604925031E-15));
#147495=CARTESIAN_POINT('',(5.87836204,-1.00000000000002,6.815046568));
#147496=CARTESIAN_POINT('',(5.878362039,0.999999999999982,6.815046569));
#147497=CARTESIAN_POINT('Ctrl Pts',(5.8783620393509,-0.999999999947016,
6.81504656862317));
#147498=CARTESIAN_POINT('Ctrl Pts',(5.83254699529058,-0.888963444643323,
6.75788176127013));
#147499=CARTESIAN_POINT('Ctrl Pts',(5.79438791271225,-0.769956469612809,
6.71027545642629));
#147500=CARTESIAN_POINT('Ctrl Pts',(5.71216089072527,-0.424051722953641,
6.60769663246045));
#147501=CARTESIAN_POINT('Ctrl Pts',(5.68712061474111,-0.188791058808674,
6.57646480876682));
#147502=CARTESIAN_POINT('Ctrl Pts',(5.69486474725044,0.283921315914245,
6.58612450427073));
#147503=CARTESIAN_POINT('Ctrl Pts',(5.72759152469994,0.516830885590786,
6.62694427419722));
#147504=CARTESIAN_POINT('Ctrl Pts',(5.81300774934532,0.826237684554357,
6.73350551678999));
#147505=CARTESIAN_POINT('Ctrl Pts',(5.84348544752745,0.915473689957744,
6.77152999685925));
#147506=CARTESIAN_POINT('Ctrl Pts',(5.87836203938029,1.0000000000182,6.81504656865984));
#147507=CARTESIAN_POINT('',(5.964297039,-1.00000000000002,6.739967421));
#147508=CARTESIAN_POINT('Origin',(1.11022302462516E-15,-1.00000000000002,
2.22044604925031E-15));
#147509=CARTESIAN_POINT('',(5.964297039,0.999999999999982,6.739967421));
#147510=CARTESIAN_POINT('Ctrl Pts',(5.96429703907415,1.00000000016684,6.73996742058037));
#147511=CARTESIAN_POINT('Ctrl Pts',(5.91379948977288,0.888963444798607,
6.68689359476872));
#147512=CARTESIAN_POINT('Ctrl Pts',(5.87174625155671,0.769956469691321,
6.64268951118086));
#147513=CARTESIAN_POINT('Ctrl Pts',(5.78113339203642,0.424051722950071,
6.54743717279022));
#147514=CARTESIAN_POINT('Ctrl Pts',(5.75354546180195,0.188791058808329,
6.5184311675852));
#147515=CARTESIAN_POINT('Ctrl Pts',(5.76207821456473,-0.283921315909946,
6.52740186632183));
#147516=CARTESIAN_POINT('Ctrl Pts',(5.79813553364251,-0.516830885584677,
6.56531182965559));
#147517=CARTESIAN_POINT('Ctrl Pts',(5.89226667286069,-0.826237684604124,
6.66425908071306));
#147518=CARTESIAN_POINT('Ctrl Pts',(5.92585590139914,-0.91547369006014,
6.69956509862226));
#147519=CARTESIAN_POINT('Ctrl Pts',(5.96429703907415,-1.00000000016687,
6.73996742058037));
#147520=CARTESIAN_POINT('Origin',(1.11022302462516E-15,0.999999999999982,
2.22044604925031E-15));
#147521=CARTESIAN_POINT('Origin',(1.11022302462516E-15,-1.77635683940025E-14,
2.22044604925031E-15));
#147522=CARTESIAN_POINT('',(6.465593547,-1.00000000000002,6.260678884));
#147523=CARTESIAN_POINT('',(6.465593547,0.999999999999982,6.260678883));
#147524=CARTESIAN_POINT('Ctrl Pts',(6.465593547415,-1.00000000013442,6.26067888331879));
#147525=CARTESIAN_POINT('Ctrl Pts',(6.41483872740882,-0.888963444774573,
6.20785103349867));
#147526=CARTESIAN_POINT('Ctrl Pts',(6.37256586579951,-0.769956469677246,
6.16385693138393));
#147527=CARTESIAN_POINT('Ctrl Pts',(6.28147477075941,-0.424051722948395,
6.06906183297416));
#147528=CARTESIAN_POINT('Ctrl Pts',(6.25373570048457,-0.188791058808251,
6.04020033244393));
#147529=CARTESIAN_POINT('Ctrl Pts',(6.26231454581812,0.283921315907732,
6.04912696217015));
#147530=CARTESIAN_POINT('Ctrl Pts',(6.29856863083365,0.516830885581569,
6.08684879800449));
#147531=CARTESIAN_POINT('Ctrl Pts',(6.39319307094974,0.826237684468099,
6.18532440503001));
#147532=CARTESIAN_POINT('Ctrl Pts',(6.42695656294875,0.915473689802837,
6.22046380990041));
#147533=CARTESIAN_POINT('Ctrl Pts',(6.46559354726348,0.999999999802907,
6.26067888316109));
#147534=CARTESIAN_POINT('',(6.544452554,-1.00000000000002,6.178198829));
#147535=CARTESIAN_POINT('Origin',(1.11022302462516E-15,-1.00000000000002,
2.22044604925031E-15));
#147536=CARTESIAN_POINT('',(6.544452554,0.999999999999982,6.178198829));
#147537=CARTESIAN_POINT('Ctrl Pts',(6.54445255390455,1.0000000000868,6.17819882890926));
#147538=CARTESIAN_POINT('Ctrl Pts',(6.48940079184017,0.888963444741015,
6.12986522815415));
#147539=CARTESIAN_POINT('Ctrl Pts',(6.44355442410623,0.769956469660416,
6.0896087204346));
#147540=CARTESIAN_POINT('Ctrl Pts',(6.34476799154022,0.424051722949287,
6.00286231406977));
#147541=CARTESIAN_POINT('Ctrl Pts',(6.3146910439409,0.188791058808277,5.97644604151514));
#147542=CARTESIAN_POINT('Ctrl Pts',(6.32399357358487,-0.28392131590895,
5.98461575679496));
#147543=CARTESIAN_POINT('Ctrl Pts',(6.36330395941132,-0.516830885583272,
6.01914095259762));
#147544=CARTESIAN_POINT('Ctrl Pts',(6.46592571753245,-0.82623768457364,
6.10925202083549));
#147545=CARTESIAN_POINT('Ctrl Pts',(6.50254453274514,-0.915473690003291,
6.1414049918512));
#147546=CARTESIAN_POINT('Ctrl Pts',(6.54445255390455,-1.00000000008684,
6.17819882890926));
#147547=CARTESIAN_POINT('Origin',(1.11022302462516E-15,0.999999999999982,
2.22044604925031E-15));
#147548=CARTESIAN_POINT('Origin',(1.11022302462516E-15,-1.77635683940025E-14,
2.22044604925031E-15));
#147549=CARTESIAN_POINT('',(7.000767897,-1.00000000000002,5.655903894));
#147550=CARTESIAN_POINT('',(7.000767897,0.999999999999982,5.655903894));
#147551=CARTESIAN_POINT('Ctrl Pts',(7.00076789655178,-1.00000000017299,
5.65590389411597));
#147552=CARTESIAN_POINT('Ctrl Pts',(6.94548194857317,-0.888963444802474,
5.60783834066879));
#147553=CARTESIAN_POINT('Ctrl Pts',(6.89943566416173,-0.769956469692457,
5.56781065596884));
#147554=CARTESIAN_POINT('Ctrl Pts',(6.80021390797847,-0.424051722949051,
5.4815625175572));
#147555=CARTESIAN_POINT('Ctrl Pts',(6.76999938208442,-0.188791058808294,
5.45530371603143));
#147556=CARTESIAN_POINT('Ctrl Pts',(6.77934386842824,0.283921315908569,
5.46342540800412));
#147557=CARTESIAN_POINT('Ctrl Pts',(6.8188333644502,0.516830885582751,5.4977455956925));
#147558=CARTESIAN_POINT('Ctrl Pts',(6.92190415979063,0.826237684604844,
5.58734269949924));
#147559=CARTESIAN_POINT('Ctrl Pts',(6.95868160192628,0.915473690063715,
5.61931410742192));
#147560=CARTESIAN_POINT('Ctrl Pts',(7.00076789655177,1.00000000017296,5.65590389411597));
#147561=CARTESIAN_POINT('',(7.071915985,-1.00000000000002,5.566687013));
#147562=CARTESIAN_POINT('Origin',(1.11022302462516E-15,-1.00000000000002,
2.22044604925031E-15));
#147563=CARTESIAN_POINT('',(7.07191598509134,1.00000000000236,5.5666870127956));
#147564=CARTESIAN_POINT('Ctrl Pts',(7.07191598491098,1.00000000000174,5.56668701304418));
#147565=CARTESIAN_POINT('Ctrl Pts',(7.01275325449934,0.888963444679149,
5.52348279108474));
#147566=CARTESIAN_POINT('Ctrl Pts',(6.96348288524122,0.769956469626121,
5.48749798096801));
#147567=CARTESIAN_POINT('Ctrl Pts',(6.85731824989088,0.424051722947126,
5.40995593770058));
#147568=CARTESIAN_POINT('Ctrl Pts',(6.82499444682085,0.188791058808083,
5.38634208609495));
#147569=CARTESIAN_POINT('Ctrl Pts',(6.83499185484784,-0.283921315906306,
5.39364504017274));
#147570=CARTESIAN_POINT('Ctrl Pts',(6.87723880331427,-0.516830885579519,
5.42450749186227));
#147571=CARTESIAN_POINT('Ctrl Pts',(6.98752493029364,-0.826237684546757,
5.50505685593149));
#147572=CARTESIAN_POINT('Ctrl Pts',(7.02687849901688,-0.915473689956015,
5.53379790323594));
#147573=CARTESIAN_POINT('Ctrl Pts',(7.07191598492155,-1.00000000002162,
5.5666870130519));
#147574=CARTESIAN_POINT('Origin',(1.11022302462516E-15,0.999999999999982,
2.22044604925031E-15));
#147575=CARTESIAN_POINT('Origin',(1.11022302462516E-15,-1.77635683940025E-14,
2.22044604925031E-15));
#147576=CARTESIAN_POINT('',(7.47957618,-1.00000000000002,5.005590892));
#147577=CARTESIAN_POINT('',(7.47957618,0.999999999999982,5.005590892));
#147578=CARTESIAN_POINT('Ctrl Pts',(7.47957617967883,-1.00000000029992,
5.00559089166839));
#147579=CARTESIAN_POINT('Ctrl Pts',(7.4202042336451,-0.888963444893634,
4.96267463016275));
#147580=CARTESIAN_POINT('Ctrl Pts',(7.37075526401692,-0.769956469741095,
4.92693564225512));
#147581=CARTESIAN_POINT('Ctrl Pts',(7.26420172190819,-0.424051722949997,
4.84992888314662));
#147582=CARTESIAN_POINT('Ctrl Pts',(7.23175500998827,-0.188791058808381,
4.82648420105958));
#147583=CARTESIAN_POINT('Ctrl Pts',(7.24178990103385,0.283921315909722,
4.83373556418914));
#147584=CARTESIAN_POINT('Ctrl Pts',(7.28419686186404,0.516830885584386,
4.86437777775458));
#147585=CARTESIAN_POINT('Ctrl Pts',(7.39488414697571,0.82623768465271,4.94437499509896));
#147586=CARTESIAN_POINT('Ctrl Pts',(7.43437942887843,0.915473690153646,
4.9729209910481));
#147587=CARTESIAN_POINT('Ctrl Pts',(7.47957617967883,1.00000000029988,5.00559089166839));
#147588=CARTESIAN_POINT('',(7.542440507,-1.00000000000002,4.910355506));
#147589=CARTESIAN_POINT('Origin',(1.11022302462516E-15,-1.00000000000002,
2.22044604925031E-15));
#147590=CARTESIAN_POINT('',(7.542440507,0.999999999999982,4.910355506));
#147591=CARTESIAN_POINT('Ctrl Pts',(7.54244050680655,0.99999999996,4.91035550643967));
#147592=CARTESIAN_POINT('Ctrl Pts',(7.47964315154329,0.888963444646452,
4.87262851828103));
#147593=CARTESIAN_POINT('Ctrl Pts',(7.42734547678568,0.769956469604149,
4.84120513431145));
#147594=CARTESIAN_POINT('Ctrl Pts',(7.31465741384491,0.42405172294144,4.77349177711884));
#147595=CARTESIAN_POINT('Ctrl Pts',(7.28034700755391,0.188791058807607,
4.75287047132403));
#147596=CARTESIAN_POINT('Ctrl Pts',(7.29095880071433,-0.283921315899282,
4.75924786510322));
#147597=CARTESIAN_POINT('Ctrl Pts',(7.33580216424092,-0.51683088556957,
4.78619908634786));
#147598=CARTESIAN_POINT('Ctrl Pts',(7.45286470105419,-0.826237684516338,
4.85653821008756));
#147599=CARTESIAN_POINT('Ctrl Pts',(7.49463617150114,-0.915473689909017,
4.88163592765426));
#147600=CARTESIAN_POINT('Ctrl Pts',(7.54244050680656,-0.999999999960036,
4.91035550643967));
#147601=CARTESIAN_POINT('Origin',(1.11022302462516E-15,0.999999999999982,
2.22044604925031E-15));
#147602=CARTESIAN_POINT('Origin',(1.11022302462516E-15,-1.77635683940025E-14,
2.22044604925031E-15));
#147603=CARTESIAN_POINT('',(7.898163313,-1.00000000000002,4.314975815));
#147604=CARTESIAN_POINT('',(7.898163313,0.999999999999982,4.314975815));
#147605=CARTESIAN_POINT('Ctrl Pts',(7.89816331281297,-1.0000000001015,4.31497581501367));
#147606=CARTESIAN_POINT('Ctrl Pts',(7.83518339679211,-0.888963444754433,
4.27755438203095));
#147607=CARTESIAN_POINT('Ctrl Pts',(7.78272987602675,-0.769956469672351,
4.24639184029318));
#147608=CARTESIAN_POINT('Ctrl Pts',(7.66970245447833,-0.424051722955082,
4.1792464736998));
#147609=CARTESIAN_POINT('Ctrl Pts',(7.63528479837203,-0.188791058808791,
4.1588046738586));
#147610=CARTESIAN_POINT('Ctrl Pts',(7.64592929907975,0.283921315916036,
4.16512732442939));
#147611=CARTESIAN_POINT('Ctrl Pts',(7.69091228881308,0.516830885593324,
4.19184485076974));
#147612=CARTESIAN_POINT('Ctrl Pts',(7.80832487473718,0.826237684586909,
4.26159809102288));
#147613=CARTESIAN_POINT('Ctrl Pts',(7.8502200035666,0.915473690017278,4.28648883936673));
#147614=CARTESIAN_POINT('Ctrl Pts',(7.89816331281297,1.00000000010146,4.31497581501367));
#147615=CARTESIAN_POINT('',(7.952237733,-1.00000000000002,4.214488703));
#147616=CARTESIAN_POINT('Origin',(1.11022302462516E-15,-1.00000000000002,
2.22044604925031E-15));
#147617=CARTESIAN_POINT('',(7.952237734,0.999999999999982,4.214488703));
#147618=CARTESIAN_POINT('Ctrl Pts',(7.9522377334233,1.00000000018981,4.21448870353033));
#147619=CARTESIAN_POINT('Ctrl Pts',(7.8863113606651,0.888963444813986,4.18254270459723));
#147620=CARTESIAN_POINT('Ctrl Pts',(7.83140745051944,0.769956469697662,
4.15593374930452));
#147621=CARTESIAN_POINT('Ctrl Pts',(7.71310325805012,0.424051722948053,
4.09859426618527));
#147622=CARTESIAN_POINT('Ctrl Pts',(7.67708249577676,0.188791058808183,
4.08113153679339));
#147623=CARTESIAN_POINT('Ctrl Pts',(7.68822323414686,-0.283921315907404,
4.08653202326162));
#147624=CARTESIAN_POINT('Ctrl Pts',(7.73530196031026,-0.516830885581086,
4.10935501872354));
#147625=CARTESIAN_POINT('Ctrl Pts',(7.8581983881465,-0.826237684457902,
4.16891757298585));
#147626=CARTESIAN_POINT('Ctrl Pts',(7.90205144094032,-0.915473689783842,
4.19016988878228));
#147627=CARTESIAN_POINT('Ctrl Pts',(7.95223773317769,-0.999999999776177,
4.21448870341132));
#147628=CARTESIAN_POINT('Origin',(1.11022302462516E-15,0.999999999999982,
2.22044604925031E-15));
#147629=CARTESIAN_POINT('Origin',(1.11022302462516E-15,-1.77635683940025E-14,
2.22044604925031E-15));
#147630=CARTESIAN_POINT('',(8.253159079,-1.00000000000002,3.58961909));
#147631=CARTESIAN_POINT('',(8.253159079,0.999999999999982,3.58961909));
#147632=CARTESIAN_POINT('Ctrl Pts',(8.25315907914881,-0.999999999891678,
3.58961909006944));
#147633=CARTESIAN_POINT('Ctrl Pts',(8.18707827043164,-0.888963444602143,
3.55799378091446));
#147634=CARTESIAN_POINT('Ctrl Pts',(8.13204252346783,-0.769956469588448,
3.5316585877518));
#147635=CARTESIAN_POINT('Ctrl Pts',(8.01345125288576,-0.424051722950382,
3.47491522857436));
#147636=CARTESIAN_POINT('Ctrl Pts',(7.97733976334233,-0.188791058808387,
3.45764089629978));
#147637=CARTESIAN_POINT('Ctrl Pts',(7.98850817044388,0.283921315910249,
3.46298392805613));
#147638=CARTESIAN_POINT('Ctrl Pts',(8.03570501247084,0.516830885585118,
3.48556165340058));
#147639=CARTESIAN_POINT('Ctrl Pts',(8.15889756203452,0.826237684503458,
3.5445093046019));
#147640=CARTESIAN_POINT('Ctrl Pts',(8.20285522282177,0.915473689866593,
3.56554439971813));
#147641=CARTESIAN_POINT('Ctrl Pts',(8.25315907914881,0.999999999891641,
3.58961909006944));
#147642=CARTESIAN_POINT('',(8.298008217,-1.00000000000002,3.484689316));
#147643=CARTESIAN_POINT('Origin',(1.11022302462516E-15,-1.00000000000002,
2.22044604925031E-15));
#147644=CARTESIAN_POINT('',(8.298008217,0.999999999999982,3.484689316));
#147645=CARTESIAN_POINT('Ctrl Pts',(8.29800821680408,0.999999999999766,
3.48468931651914));
#147646=CARTESIAN_POINT('Ctrl Pts',(8.22948362702398,0.888963444677765,
3.45878151730231));
#147647=CARTESIAN_POINT('Ctrl Pts',(8.17241553555401,0.769956469625439,
3.43720123042083));
#147648=CARTESIAN_POINT('Ctrl Pts',(8.04944772936533,0.424051722947189,
3.39069728527389));
#147649=CARTESIAN_POINT('Ctrl Pts',(8.01200662909584,0.188791058808109,
3.37653373193536));
#147650=CARTESIAN_POINT('Ctrl Pts',(8.02358661400347,-0.28392131590634,
3.38091382954382));
#147651=CARTESIAN_POINT('Ctrl Pts',(8.07252165259768,-0.51683088557958,
3.39942484185536));
#147652=CARTESIAN_POINT('Ctrl Pts',(8.20026248178416,-0.826237684538796,
3.447731263932));
#147653=CARTESIAN_POINT('Ctrl Pts',(8.24584403802863,-0.915473689940678,
3.46496706682217));
#147654=CARTESIAN_POINT('Ctrl Pts',(8.29800821680408,-0.999999999999798,
3.48468931651914));
#147655=CARTESIAN_POINT('Origin',(1.11022302462516E-15,0.999999999999982,
2.22044604925031E-15));
#147656=CARTESIAN_POINT('Origin',(1.11022302462516E-15,-1.77635683940025E-14,
2.22044604925031E-15));
#147657=CARTESIAN_POINT('',(8.541705262,-1.00000000000002,2.835360862));
#147658=CARTESIAN_POINT('',(8.541705262,0.999999999999982,2.835360862));
#147659=CARTESIAN_POINT('Ctrl Pts',(8.54170526179937,-1.00000000003984,
2.83536086236564));
#147660=CARTESIAN_POINT('Ctrl Pts',(8.47305560408873,-0.888963444708827,
2.80978630543292));
#147661=CARTESIAN_POINT('Ctrl Pts',(8.41588074631203,-0.769956469645811,
2.78849049633942));
#147662=CARTESIAN_POINT('Ctrl Pts',(8.29268045378883,-0.424051722952013,
2.74260600880004));
#147663=CARTESIAN_POINT('Ctrl Pts',(8.25516587927574,-0.188791058808545,
2.72863822688282));
#147664=CARTESIAN_POINT('Ctrl Pts',(8.26676827132905,0.283921315912221,
2.73295862086762));
#147665=CARTESIAN_POINT('Ctrl Pts',(8.31579896444623,0.516830885587926,
2.75121476261534));
#147666=CARTESIAN_POINT('Ctrl Pts',(8.44377960377111,0.826237684560039,
2.79888221287883));
#147667=CARTESIAN_POINT('Ctrl Pts',(8.48944587536212,0.915473689971902,
2.81589229255365));
#147668=CARTESIAN_POINT('Ctrl Pts',(8.54170526179937,1.00000000003981,2.83536086236564));
#147669=CARTESIAN_POINT('',(8.576968018,-1.00000000000002,2.726833259));
#147670=CARTESIAN_POINT('Origin',(1.11022302462516E-15,-1.00000000000002,
2.22044604925031E-15));
#147671=CARTESIAN_POINT('',(8.576968018,0.999999999999982,2.726833259));
#147672=CARTESIAN_POINT('Ctrl Pts',(8.57696801766623,1.00000000014478,2.72683325938026));
#147673=CARTESIAN_POINT('Ctrl Pts',(8.50639693048896,0.888963444783309,
2.70717225418446));
#147674=CARTESIAN_POINT('Ctrl Pts',(8.44762413635101,0.769956469684064,
2.69079438744694));
#147675=CARTESIAN_POINT('Ctrl Pts',(8.32098278088488,0.424051722950995,
2.65550040263089));
#147676=CARTESIAN_POINT('Ctrl Pts',(8.28242279634777,0.188791058808397,
2.64475006193496));
#147677=CARTESIAN_POINT('Ctrl Pts',(8.29434879256285,-0.283921315911108,
2.6480745047178));
#147678=CARTESIAN_POINT('Ctrl Pts',(8.34474614742513,-0.516830885586315,
2.6621244941107));
#147679=CARTESIAN_POINT('Ctrl Pts',(8.4763028838897,-0.826237684597308,
2.69878584913351));
#147680=CARTESIAN_POINT('Ctrl Pts',(8.52324594767412,-0.915473690045216,
2.71186636657059));
#147681=CARTESIAN_POINT('Ctrl Pts',(8.57696801766623,-1.00000000014482,
2.72683325938026));
#147682=CARTESIAN_POINT('Origin',(1.11022302462516E-15,0.999999999999982,
2.22044604925031E-15));
#147683=CARTESIAN_POINT('Origin',(1.11022302462516E-15,-1.77635683940025E-14,
2.22044604925031E-15));
#147684=CARTESIAN_POINT('',(8.761478656,-1.00000000000002,2.058273977));
#147685=CARTESIAN_POINT('',(8.761478656,0.999999999999982,2.058273976));
#147686=CARTESIAN_POINT('Ctrl Pts',(8.76147865594458,-1.00000000014044,
2.0582739763956));
#147687=CARTESIAN_POINT('Ctrl Pts',(8.69081287594316,-0.888963444777774,
2.03895608293596));
#147688=CARTESIAN_POINT('Ctrl Pts',(8.63195924570963,-0.769956469677081,
2.02287111920753));
#147689=CARTESIAN_POINT('Ctrl Pts',(8.50514186759659,-0.424051722946206,
1.98821493812971));
#147690=CARTESIAN_POINT('Ctrl Pts',(8.46652625341953,-0.188791058808058,
1.97766616690805));
#147691=CARTESIAN_POINT('Ctrl Pts',(8.47846921478163,0.283921315905046,
1.98092913785784));
#147692=CARTESIAN_POINT('Ctrl Pts',(8.52893899266448,0.516830885577759,
1.99471670832763));
#147693=CARTESIAN_POINT('Ctrl Pts',(8.66067729683783,0.82623768454449,2.03072016746057));
#147694=CARTESIAN_POINT('Ctrl Pts',(8.70768450122283,0.915473689953662,
2.04356827655552));
#147695=CARTESIAN_POINT('Ctrl Pts',(8.76147865586744,1.00000000001919,2.05827397637451));
#147696=CARTESIAN_POINT('',(8.786871115,-1.00000000000002,1.947022346));
#147697=CARTESIAN_POINT('Origin',(1.11022302462516E-15,-1.00000000000002,
2.22044604925031E-15));
#147698=CARTESIAN_POINT('',(8.786871115,0.999999999999982,1.947022345));
#147699=CARTESIAN_POINT('Ctrl Pts',(8.78687111468735,1.00000000013172,1.94702234559588));
#147700=CARTESIAN_POINT('Ctrl Pts',(8.71482172704381,0.888963444773286,
1.93376643331344));
#147701=CARTESIAN_POINT('Ctrl Pts',(8.65481743424227,0.769956469677654,
1.92272285170413));
#147702=CARTESIAN_POINT('Ctrl Pts',(8.52552217123475,0.424051722949642,
1.89892299368291));
#147703=CARTESIAN_POINT('Ctrl Pts',(8.48615376474826,0.188791058808303,
1.89167242106493));
#147704=CARTESIAN_POINT('Ctrl Pts',(8.49832975116214,-0.283921315909392,
1.89391444255924));
#147705=CARTESIAN_POINT('Ctrl Pts',(8.54978365242985,-0.516830885583896,
1.90339028676294));
#147706=CARTESIAN_POINT('Ctrl Pts',(8.68409707869062,-0.826237684621147,
1.92811139900698));
#147707=CARTESIAN_POINT('Ctrl Pts',(8.73202369206082,-0.915473690093674,
1.93693131433199));
#147708=CARTESIAN_POINT('Ctrl Pts',(8.78687111474133,-1.00000000021493,
1.94702234560581));
#147709=CARTESIAN_POINT('Origin',(1.11022302462516E-15,0.999999999999982,
2.22044604925031E-15));
#147710=CARTESIAN_POINT('Origin',(1.11022302462516E-15,-1.77635683940025E-14,
2.22044604925031E-15));
#147711=CARTESIAN_POINT('',(8.910709775,-1.00000000000002,1.264615079));
#147712=CARTESIAN_POINT('',(8.910709775,0.999999999999982,1.264615079));
#147713=CARTESIAN_POINT('Ctrl Pts',(8.91070977524219,-0.999999999833344,
1.26461507908072));
#147714=CARTESIAN_POINT('Ctrl Pts',(8.83859683236404,-0.888963444559491,
1.25170938549312));
#147715=CARTESIAN_POINT('Ctrl Pts',(8.77853828457744,-0.769956469564432,
1.24096477386405));
#147716=CARTESIAN_POINT('Ctrl Pts',(8.64912487986268,-0.424051722948475,
1.21781593054578));
#147717=CARTESIAN_POINT('Ctrl Pts',(8.60971913623194,-0.188791058808248,
1.21077110255089));
#147718=CARTESIAN_POINT('Ctrl Pts',(8.62190650920452,0.283921315907853,
1.21295037893395));
#147719=CARTESIAN_POINT('Ctrl Pts',(8.67340901888982,0.516830885581736,
1.2221583686789));
#147720=CARTESIAN_POINT('Ctrl Pts',(8.80784430855032,0.826237684479382,
1.24620795789709));
#147721=CARTESIAN_POINT('Ctrl Pts',(8.85581397133016,0.915473689824291,
1.25479065095093));
#147722=CARTESIAN_POINT('Ctrl Pts',(8.91070977524219,0.999999999833308,
1.26461507908072));
#147723=CARTESIAN_POINT('',(8.926027492,-1.00000000000002,1.151535151));
#147724=CARTESIAN_POINT('Origin',(1.11022302462516E-15,-1.00000000000002,
2.22044604925031E-15));
#147725=CARTESIAN_POINT('',(8.926027492,0.999999999999982,1.151535151));
#147726=CARTESIAN_POINT('Ctrl Pts',(8.92602749223077,0.999999999828974,
1.15153515131936));
#147727=CARTESIAN_POINT('Ctrl Pts',(8.85307990351357,0.888963444557652,
1.14479106076096));
#147728=CARTESIAN_POINT('Ctrl Pts',(8.79232723139907,0.769956469565621,
1.13917068070444));
#147729=CARTESIAN_POINT('Ctrl Pts',(8.66141907032706,0.424051722951004,
1.12705657192987));
#147730=CARTESIAN_POINT('Ctrl Pts',(8.6215592131525,0.188791058808435,1.12336414473294));
#147731=CARTESIAN_POINT('Ctrl Pts',(8.63388715588223,-0.283921315911035,
1.12450569350138));
#147732=CARTESIAN_POINT('Ctrl Pts',(8.68598332699613,-0.516830885586233,
1.12933109859576));
#147733=CARTESIAN_POINT('Ctrl Pts',(8.82197203024378,-0.826237684481341,
1.14191292820709));
#147734=CARTESIAN_POINT('Ctrl Pts',(8.87049631618663,-0.915473689822919,
1.14640122864087));
#147735=CARTESIAN_POINT('Ctrl Pts',(8.92602749223077,-0.99999999982901,
1.15153515131936));
#147736=CARTESIAN_POINT('Origin',(1.11022302462516E-15,0.999999999999982,
2.22044604925031E-15));
#147737=CARTESIAN_POINT('Origin',(1.11022302462516E-15,-1.77635683940025E-14,
2.22044604925031E-15));
#147738=CARTESIAN_POINT('',(8.988197099,-1.00000000000002,0.460774244000002));
#147739=CARTESIAN_POINT('',(8.988197099,0.999999999999982,0.460774244000002));
#147740=CARTESIAN_POINT('Ctrl Pts',(8.98819709915994,-0.999999999884687,
0.460774244177401));
#147741=CARTESIAN_POINT('Ctrl Pts',(8.91521760431959,-0.888963444596554,
0.454384659487097));
#147742=CARTESIAN_POINT('Ctrl Pts',(8.85443769501692,-0.76995646958452,
0.449066909228441));
#147743=CARTESIAN_POINT('Ctrl Pts',(8.72347022429716,-0.424051722949224,
0.437611784522525));
#147744=CARTESIAN_POINT('Ctrl Pts',(8.68359162309196,-0.188791058808323,
0.434127620564111));
#147745=CARTESIAN_POINT('Ctrl Pts',(8.69592528211311,0.283921315908744,
0.435205656129238));
#147746=CARTESIAN_POINT('Ctrl Pts',(8.74804585567359,0.516830885583003,
0.439759927834071));
#147747=CARTESIAN_POINT('Ctrl Pts',(8.88409573694761,0.826237684499239,
0.451662014005322));
#147748=CARTESIAN_POINT('Ctrl Pts',(8.93264163465328,0.9154736898609,0.455910188236056));
#147749=CARTESIAN_POINT('Ctrl Pts',(8.98819709915994,0.999999999884651,
0.4607742441774));
#147750=CARTESIAN_POINT('',(8.993316745,-1.00000000000002,0.346776472999999));
#147751=CARTESIAN_POINT('Origin',(1.11022302462516E-15,-1.00000000000002,
2.22044604925031E-15));
#147752=CARTESIAN_POINT('',(8.993316745,0.999999999999982,0.346776472999999));
#147753=CARTESIAN_POINT('Ctrl Pts',(8.99331674501375,0.999999999990159,
0.346776473469501));
#147754=CARTESIAN_POINT('Ctrl Pts',(8.9200582861779,0.888963444672463,0.346598504082614));
#147755=CARTESIAN_POINT('Ctrl Pts',(8.85904637943988,0.769956469625277,
0.34644657757194));
#147756=CARTESIAN_POINT('Ctrl Pts',(8.72757931577641,0.424051722950287,
0.346115753738563));
#147757=CARTESIAN_POINT('Ctrl Pts',(8.68754893604615,0.18879105880837,0.346011201221874));
#147758=CARTESIAN_POINT('Ctrl Pts',(8.69992957774535,-0.283921315910157,
0.346043086182914));
#147759=CARTESIAN_POINT('Ctrl Pts',(8.75224857096816,-0.516830885584986,
0.346179200834908));
#147760=CARTESIAN_POINT('Ctrl Pts',(8.88881765021394,-0.826237684539527,
0.346520446308495));
#147761=CARTESIAN_POINT('Ctrl Pts',(8.93754891983274,-0.915473689935908,
0.346640994702773));
#147762=CARTESIAN_POINT('Ctrl Pts',(8.99331674501375,-0.999999999990195,
0.346776473469501));
#147763=CARTESIAN_POINT('Origin',(1.11022302462516E-15,0.999999999999982,
2.22044604925031E-15));
#147764=CARTESIAN_POINT('Origin',(1.11022302462516E-15,-1.50000000000002,
2.22044604925031E-15));
#147765=CARTESIAN_POINT('',(2.50000000035605,-1.09999999964397,2.52660774908075E-15));
#147766=CARTESIAN_POINT('',(-2.5,-1.10000000000002,2.52660774903715E-15));
#147767=CARTESIAN_POINT('Origin',(1.11022302462516E-15,-1.10000000000002,
2.22044604925031E-15));
#147768=CARTESIAN_POINT('',(2.9,-1.50000000000002,2.57559362100305E-15));
#147769=CARTESIAN_POINT('',(2.9,-1.50000000000002,2.57559362100305E-15));
#147770=CARTESIAN_POINT('Origin',(1.11022302462516E-15,-1.50000000000002,
2.22044604925031E-15));
#147771=CARTESIAN_POINT('Origin',(1.11022302462516E-15,-1.10000000000002,
2.22044604925031E-15));
#147772=CARTESIAN_POINT('Origin',(-6.,-1.30000000000002,2.22044604925031E-15));
#147773=CARTESIAN_POINT('',(-4.5,-1.30000000000002,2.40414306912242E-15));
#147774=CARTESIAN_POINT('',(-7.5,-1.30000000000002,2.40414306912242E-15));
#147775=CARTESIAN_POINT('Origin',(-6.,-1.30000000000002,2.22044604925031E-15));
#147776=CARTESIAN_POINT('',(-4.30000000017802,-1.50000000017804,2.42863600508356E-15));
#147777=CARTESIAN_POINT('',(-4.5,-1.30000000000002,2.40414306912242E-15));
#147778=CARTESIAN_POINT('Origin',(-6.,-1.50000000000002,2.22044604925031E-15));
#147779=CARTESIAN_POINT('Origin',(-6.,-1.30000000000002,2.22044604925031E-15));
#147780=CARTESIAN_POINT('Origin',(6.,-1.30000000000002,2.22044604925031E-15));
#147781=CARTESIAN_POINT('',(7.5,-1.30000000000002,2.40414306912242E-15));
#147782=CARTESIAN_POINT('',(4.5,-1.30000000000002,2.40414306912242E-15));
#147783=CARTESIAN_POINT('Origin',(6.,-1.30000000000002,2.22044604925031E-15));
#147784=CARTESIAN_POINT('',(7.69999999982198,-1.50000000017804,2.42863600508356E-15));
#147785=CARTESIAN_POINT('',(7.5,-1.30000000000002,2.40414306912242E-15));
#147786=CARTESIAN_POINT('Origin',(6.,-1.50000000000002,2.22044604925031E-15));
#147787=CARTESIAN_POINT('Origin',(6.,-1.30000000000002,2.22044604925031E-15));
#147788=CARTESIAN_POINT('Origin',(1.11022302462516E-15,2.49999999999998,
2.22044604925031E-15));
#147789=CARTESIAN_POINT('',(8.99999999982198,2.29999999982196,3.32262816846113E-15));
#147790=CARTESIAN_POINT('',(-9.,2.29999999999998,3.32262816848293E-15));
#147791=CARTESIAN_POINT('Origin',(1.11022302462516E-15,2.29999999999998,
2.22044604925031E-15));
#147792=CARTESIAN_POINT('',(8.8,2.49999999999998,3.29813523249998E-15));
#147793=CARTESIAN_POINT('',(8.8,2.49999999999998,3.29813523249998E-15));
#147794=CARTESIAN_POINT('Origin',(1.11022302462516E-15,2.49999999999998,
2.22044604925031E-15));
#147795=CARTESIAN_POINT('Origin',(1.11022302462516E-15,2.29999999999998,
2.22044604925031E-15));
#147796=CARTESIAN_POINT('Origin',(6.,2.49999999999998,2.22044604925031E-15));
#147797=CARTESIAN_POINT('',(4.49999999982198,2.29999999982196,2.40414306914422E-15));
#147798=CARTESIAN_POINT('Origin',(6.,2.29999999999998,2.22044604925031E-15));
#147799=CARTESIAN_POINT('',(4.3,2.49999999999998,2.42863600510536E-15));
#147800=CARTESIAN_POINT('',(4.3,2.49999999999998,2.42863600510536E-15));
#147801=CARTESIAN_POINT('Origin',(6.,2.49999999999998,2.22044604925031E-15));
#147802=CARTESIAN_POINT('Origin',(-6.,2.49999999999998,2.22044604925031E-15));
#147803=CARTESIAN_POINT('',(-7.50000000017802,2.29999999982196,2.40414306914422E-15));
#147804=CARTESIAN_POINT('Origin',(-6.,2.29999999999998,2.22044604925031E-15));
#147805=CARTESIAN_POINT('',(-7.7,2.49999999999998,2.42863600510536E-15));
#147806=CARTESIAN_POINT('',(-7.7,2.49999999999998,2.42863600510536E-15));
#147807=CARTESIAN_POINT('Origin',(-6.,2.49999999999998,2.22044604925031E-15));
#147808=CARTESIAN_POINT('Origin',(1.11022302462516E-15,4.99999999999998,
2.22044604925031E-15));
#147809=CARTESIAN_POINT('',(3.49999999982198,4.79999999982196,2.64907242893008E-15));
#147810=CARTESIAN_POINT('',(-3.5,4.79999999999998,2.64907242895189E-15));
#147811=CARTESIAN_POINT('Origin',(1.11022302462516E-15,4.79999999999998,
2.22044604925031E-15));
#147812=CARTESIAN_POINT('',(3.3,4.99999999999998,2.62457949296894E-15));
#147813=CARTESIAN_POINT('',(3.3,4.99999999999998,2.62457949296894E-15));
#147814=CARTESIAN_POINT('Origin',(1.11022302462516E-15,4.99999999999998,
2.22044604925031E-15));
#147815=CARTESIAN_POINT('Origin',(1.11022302462516E-15,4.79999999999998,
2.22044604925031E-15));
#147816=CARTESIAN_POINT('Origin',(1.11022302462516E-15,4.79999999999998,
2.22044604925031E-15));
#147817=CARTESIAN_POINT('',(-2.5,4.79999999999998,2.52660774903715E-15));
#147818=CARTESIAN_POINT('Origin',(1.11022302462516E-15,4.79999999999998,
2.22044604925031E-15));
#147819=CARTESIAN_POINT('',(-2.69999999982198,5.00000000017801,2.5511006849983E-15));
#147820=CARTESIAN_POINT('',(-2.5,4.79999999999998,2.52660774903715E-15));
#147821=CARTESIAN_POINT('Origin',(1.11022302462516E-15,4.99999999999998,
2.22044604925031E-15));
#147822=CARTESIAN_POINT('Origin',(-6.,-1.50000000000002,2.22044604925031E-15));
#147823=CARTESIAN_POINT('',(-7.5,-1.50000000000002,2.40414306912242E-15));
#147824=CARTESIAN_POINT('Origin',(6.,-1.50000000000002,2.22044604925031E-15));
#147825=CARTESIAN_POINT('',(4.5,-1.50000000000002,2.40414306912242E-15));
#147826=CARTESIAN_POINT('Origin',(1.11022302462516E-15,-1.00000000000002,
2.22044604925031E-15));
#147827=CARTESIAN_POINT('',(8.671878177,-1.32768940200002,0.0866025400000026));
#147828=CARTESIAN_POINT('',(8.671878177,-1.32768940200002,-0.0866025400000003));
#147829=CARTESIAN_POINT('Ctrl Pts',(8.67187817702724,-1.32768940206672,
0.0866025400494723));
#147830=CARTESIAN_POINT('Ctrl Pts',(8.66616846994706,-1.3334449271527,0.0819858522682004));
#147831=CARTESIAN_POINT('Ctrl Pts',(8.66092780725788,-1.33873894467796,
0.0762673294526388));
#147832=CARTESIAN_POINT('Ctrl Pts',(8.64993438117684,-1.34985996696303,
0.0603505832064055));
#147833=CARTESIAN_POINT('Ctrl Pts',(8.64487598591024,-1.35499086504381,
0.0494502637821226));
#147834=CARTESIAN_POINT('Ctrl Pts',(8.63800999226789,-1.36196031874185,
0.0255744021040338));
#147835=CARTESIAN_POINT('Ctrl Pts',(8.63624826494697,-1.36375173570061,
0.0128536662840273));
#147836=CARTESIAN_POINT('Ctrl Pts',(8.63624826494697,-1.36375173570061,
2.22044604925031E-15));
#147837=CARTESIAN_POINT('Ctrl Pts',(8.63624826494697,-1.36375173570061,
-0.00730777731083654));
#147838=CARTESIAN_POINT('Ctrl Pts',(8.63681787290187,-1.36317274212995,
-0.0145911248958308));
#147839=CARTESIAN_POINT('Ctrl Pts',(8.63907576227445,-1.3608789882621,-0.0288572911900964));
#147840=CARTESIAN_POINT('Ctrl Pts',(8.64075793401352,-1.35917045581577,
-0.0357924289474276));
#147841=CARTESIAN_POINT('Ctrl Pts',(8.64690488602001,-1.35293307609673,
-0.0542397254755866));
#147842=CARTESIAN_POINT('Ctrl Pts',(8.65245472483424,-1.34730670087632,
-0.0648458367127547));
#147843=CARTESIAN_POINT('Ctrl Pts',(8.66314315367645,-1.33650155461798,
-0.0786155019109556));
#147844=CARTESIAN_POINT('Ctrl Pts',(8.66736782138124,-1.33223595142604,
-0.0829556097415421));
#147845=CARTESIAN_POINT('Ctrl Pts',(8.67187817702726,-1.3276894020667,-0.0866025400494835));
#147846=CARTESIAN_POINT('Ctrl Pts',(8.99331674490455,-1.00000000018596,
0.346776473354771));
#147847=CARTESIAN_POINT('Ctrl Pts',(8.88752172769541,-1.10901473823108,
0.261175104387876));
#147848=CARTESIAN_POINT('Ctrl Pts',(8.78035308155774,-1.21834403191783,
0.174311900770753));
#147849=CARTESIAN_POINT('Ctrl Pts',(8.67187817714367,-1.32768940195315,
0.0866025397638899));
#147850=CARTESIAN_POINT('',(8.644730737,-1.32768940200002,0.691087263000001));
#147851=CARTESIAN_POINT('Ctrl Pts',(8.64473073694086,-1.32768940194368,
0.69108726299106));
#147852=CARTESIAN_POINT('Ctrl Pts',(8.76063136896071,-1.21834383455991,
0.61345446945312));
#147853=CARTESIAN_POINT('Ctrl Pts',(8.87515482087759,-1.10901465443497,
0.53654755682168));
#147854=CARTESIAN_POINT('Ctrl Pts',(8.9881970992204,-1.00000000007974,0.460774244214116));
#147855=CARTESIAN_POINT('',(8.629204753,-1.32768940200002,0.863595070000001));
#147856=CARTESIAN_POINT('Ctrl Pts',(8.64473073689486,-1.3276894020015,0.691087262840869));
#147857=CARTESIAN_POINT('Ctrl Pts',(8.63991163031322,-1.33223595135028,
0.694315206512238));
#147858=CARTESIAN_POINT('Ctrl Pts',(8.63531492562229,-1.33650155453273,
0.698259146043817));
#147859=CARTESIAN_POINT('Ctrl Pts',(8.62343522198836,-1.34730670078397,
0.711015275232578));
#147860=CARTESIAN_POINT('Ctrl Pts',(8.6169570007115,-1.35293307600527,0.721081205667737));
#147861=CARTESIAN_POINT('Ctrl Pts',(8.60918119161373,-1.35917045572572,
0.738903230273293));
#147862=CARTESIAN_POINT('Ctrl Pts',(8.60688413084748,-1.36087898817255,
0.745659660492595));
#147863=CARTESIAN_POINT('Ctrl Pts',(8.6033565217857,-1.36317274204141,0.759665999752384));
#147864=CARTESIAN_POINT('Ctrl Pts',(8.6021363326606,-1.36375173561258,0.766868967457794));
#147865=CARTESIAN_POINT('Ctrl Pts',(8.6014812685525,-1.36375173561308,0.774147325805647));
#147866=CARTESIAN_POINT('Ctrl Pts',(8.60032907478934,-1.36375173561396,
0.786949247007953));
#147867=CARTESIAN_POINT('Ctrl Pts',(8.60094343194574,-1.36196031865609,
0.799776692904925));
#147868=CARTESIAN_POINT('Ctrl Pts',(8.60564156937475,-1.35499086495975,
0.82417190030865));
#147869=CARTESIAN_POINT('Ctrl Pts',(8.60970250392851,-1.3498599668798,0.835481769307738));
#147870=CARTESIAN_POINT('Ctrl Pts',(8.61922490753858,-1.33873894463695,
0.852319882468268));
#147871=CARTESIAN_POINT('Ctrl Pts',(8.62393186837942,-1.33344492716415,
0.858485153528086));
#147872=CARTESIAN_POINT('Ctrl Pts',(8.6292047530988,-1.3276894021372,0.863595070052561));
#147873=CARTESIAN_POINT('Ctrl Pts',(8.92602749216612,-1.00000000026639,
1.1515351511352));
#147874=CARTESIAN_POINT('Ctrl Pts',(8.8283316221154,-1.10901473835186,1.0567949958371));
#147875=CARTESIAN_POINT('Ctrl Pts',(8.72938076294725,-1.2183440320791,0.960674954515168));
#147876=CARTESIAN_POINT('Ctrl Pts',(8.6292047530771,-1.32768940215461,0.863595070094576));
#147877=CARTESIAN_POINT('',(8.547981008,-1.32768940200002,1.463212838));
#147878=CARTESIAN_POINT('Ctrl Pts',(8.54798100788837,-1.32768940187192,
1.46321283800514));
#147879=CARTESIAN_POINT('Ctrl Pts',(8.67037400794378,-1.21834383453907,
1.39628182386026));
#147880=CARTESIAN_POINT('Ctrl Pts',(8.79133030455683,-1.10901465446516,
1.32995031896543));
#147881=CARTESIAN_POINT('Ctrl Pts',(8.91070977524376,-1.00000000016074,
1.26461507917722));
#147882=CARTESIAN_POINT('',(8.517054046,-1.32768940200002,1.633634441));
#147883=CARTESIAN_POINT('Ctrl Pts',(8.54798100783859,-1.32768940196088,
1.4632128377687));
#147884=CARTESIAN_POINT('Ctrl Pts',(8.5428919508647,-1.33223595136504,1.46599580531845));
#147885=CARTESIAN_POINT('Ctrl Pts',(8.53796021908521,-1.33650155459769,
1.4695118223078));
#147886=CARTESIAN_POINT('Ctrl Pts',(8.52498488898969,-1.34730670089114,
1.48115171069211));
#147887=CARTESIAN_POINT('Ctrl Pts',(8.5176304440792,-1.3529330761124,1.49059641537225));
#147888=CARTESIAN_POINT('Ctrl Pts',(8.50828838413339,-1.35917045583282,
1.50764967559236));
#147889=CARTESIAN_POINT('Ctrl Pts',(8.50539492892274,-1.36087898827965,
1.51417299947031));
#147890=CARTESIAN_POINT('Ctrl Pts',(8.50062600240598,-1.36317274214851,
1.52780674088759));
#147891=CARTESIAN_POINT('Ctrl Pts',(8.49876505635617,-1.36375173571968,
1.53487133465274));
#147892=CARTESIAN_POINT('Ctrl Pts',(8.4974602023311,-1.36375173572018,1.54206167297575));
#147893=CARTESIAN_POINT('Ctrl Pts',(8.49516509159167,-1.36375173572105,
1.55470877555439));
#147894=CARTESIAN_POINT('Ctrl Pts',(8.49462713214117,-1.36196031876316,
1.56753965247642));
#147895=CARTESIAN_POINT('Ctrl Pts',(8.49711958671715,-1.35499086506676,
1.59225778973971));
#147896=CARTESIAN_POINT('Ctrl Pts',(8.50015036430107,-1.34985996698678,
1.6038861478983));
#147897=CARTESIAN_POINT('Ctrl Pts',(8.50812507669321,-1.33873894473423,
1.62151005745983));
#147898=CARTESIAN_POINT('Ctrl Pts',(8.51226043806651,-1.33344492724917,
1.62807243767969));
#147899=CARTESIAN_POINT('Ctrl Pts',(8.51705404632889,-1.3276894022084,1.63363444093218));
#147900=CARTESIAN_POINT('Ctrl Pts',(8.78687111486193,-0.999999999752185,
1.94702234585691));
#147901=CARTESIAN_POINT('Ctrl Pts',(8.69806098154262,-1.10901473805156,
1.84390619609545));
#147902=CARTESIAN_POINT('Ctrl Pts',(8.60812460334816,-1.2183440319946,1.73930321896202));
#147903=CARTESIAN_POINT('Ctrl Pts',(8.51705404621577,-1.327689402286,1.63363444110997));
#147904=CARTESIAN_POINT('',(8.382407962,-1.32768940200002,2.223557482));
#147905=CARTESIAN_POINT('Ctrl Pts',(8.38240796213464,-1.32768940171091,
2.22355748287687));
#147906=CARTESIAN_POINT('Ctrl Pts',(8.51030789375738,-1.21834383440846,
2.16786713730407));
#147907=CARTESIAN_POINT('Ctrl Pts',(8.63672316609019,-1.10901465436549,
2.11264510242942));
#147908=CARTESIAN_POINT('Ctrl Pts',(8.7614786558207,-1.00000000009201,2.05827397640414));
#147909=CARTESIAN_POINT('',(8.336329029,-1.32768940200002,2.390520747));
#147910=CARTESIAN_POINT('Ctrl Pts',(8.38240796207935,-1.32768940188413,
2.22355748240969));
#147911=CARTESIAN_POINT('Ctrl Pts',(8.37708992878106,-1.33223595136664,
2.22587306701158));
#147912=CARTESIAN_POINT('Ctrl Pts',(8.37186287728827,-1.33650155467049,
2.22893285255653));
#147913=CARTESIAN_POINT('Ctrl Pts',(8.3578963904289,-1.34730670102585,2.23936278260429));
#147914=CARTESIAN_POINT('Ctrl Pts',(8.34972493555017,-1.35293307624908,
2.24811021831966));
#147915=CARTESIAN_POINT('Ctrl Pts',(8.3388918415288,-1.35917045597279,2.26425741132905));
#147916=CARTESIAN_POINT('Ctrl Pts',(8.33542528827331,-1.36087898842084,
2.27049510689713));
#147917=CARTESIAN_POINT('Ctrl Pts',(8.32945344089288,-1.36317274229213,
2.28364647960213));
#147918=CARTESIAN_POINT('Ctrl Pts',(8.32696672116126,-1.36375173586451,
2.29051581947185));
#147919=CARTESIAN_POINT('Ctrl Pts',(8.32502258313609,-1.36375173586619,
2.29756024539374));
#147920=CARTESIAN_POINT('Ctrl Pts',(8.32160303430179,-1.36375173586915,
2.30995070231481));
#147921=CARTESIAN_POINT('Ctrl Pts',(8.31991708957669,-1.36196031891332,
2.32268170358541));
#147922=CARTESIAN_POINT('Ctrl Pts',(8.32018379351913,-1.35499086522079,
2.34752375480154));
#147923=CARTESIAN_POINT('Ctrl Pts',(8.32216001209317,-1.3498599671427,2.3593769774175));
#147924=CARTESIAN_POINT('Ctrl Pts',(8.32852282561185,-1.3387389448062,2.37764478615217));
#147925=CARTESIAN_POINT('Ctrl Pts',(8.33205329208909,-1.33344492721209,
2.3845514392093));
#147926=CARTESIAN_POINT('Ctrl Pts',(8.33632902867257,-1.32768940204801,
2.39052074728081));
#147927=CARTESIAN_POINT('Ctrl Pts',(8.57696801758913,-1.00000000005396,
2.72683325934723));
#147928=CARTESIAN_POINT('Ctrl Pts',(8.4977586683085,-1.10901473814976,2.61617134608161));
#147929=CARTESIAN_POINT('Ctrl Pts',(8.41756088626376,-1.21834403188794,
2.50392763516743));
#147930=CARTESIAN_POINT('Ctrl Pts',(8.33632902879468,-1.32768940197433,
2.3905207471223));
#147931=CARTESIAN_POINT('',(8.149344695,-1.32768940200002,2.965999351));
#147932=CARTESIAN_POINT('Ctrl Pts',(8.1493446952874,-1.32768940216563,2.96599935145307));
#147933=CARTESIAN_POINT('Ctrl Pts',(8.281721783784,-1.21834383463976,2.92199806015237));
#147934=CARTESIAN_POINT('Ctrl Pts',(8.41257821073727,-1.10901465437208,
2.87833011043717));
#147935=CARTESIAN_POINT('Ctrl Pts',(8.54170526199449,-0.999999999874976,
2.83536086230067));
#147936=CARTESIAN_POINT('',(8.088484791,-1.32768940200002,3.128159987));
#147937=CARTESIAN_POINT('Ctrl Pts',(8.14934469528429,-1.32768940220673,
2.96599935134145));
#147938=CARTESIAN_POINT('Ctrl Pts',(8.14384050348253,-1.33223595163132,
2.96782890925026));
#147939=CARTESIAN_POINT('Ctrl Pts',(8.13836021756285,-1.33650155488223,
2.97040782769713));
#147940=CARTESIAN_POINT('Ctrl Pts',(8.12351502401358,-1.3473067011882,2.97954382365383));
#147941=CARTESIAN_POINT('Ctrl Pts',(8.11459235092013,-1.35293307640658,
2.98752356120022));
#147942=CARTESIAN_POINT('Ctrl Pts',(8.10235544453278,-1.35917045612245,
3.00263467930046));
#147943=CARTESIAN_POINT('Ctrl Pts',(8.09834370388334,-1.36087898856765,
3.00853652430322));
#147944=CARTESIAN_POINT('Ctrl Pts',(8.09121701744786,-1.36317274243324,
3.02109964117804));
#147945=CARTESIAN_POINT('Ctrl Pts',(8.08812454564212,-1.36375173600275,
3.02771841926748));
#147946=CARTESIAN_POINT('Ctrl Pts',(8.08555677667574,-1.36375173600163,
3.03456021521294));
#147947=CARTESIAN_POINT('Ctrl Pts',(8.08104032194735,-1.36375173599966,
3.04659426580439));
#147948=CARTESIAN_POINT('Ctrl Pts',(8.07821996618797,-1.36196031903889,
3.05912288888715));
#147949=CARTESIAN_POINT('Ctrl Pts',(8.0762587721631,-1.35499086533698,3.08388884046511));
#147950=CARTESIAN_POINT('Ctrl Pts',(8.07716452038241,-1.34985996725432,
3.09587149235794));
#147951=CARTESIAN_POINT('Ctrl Pts',(8.08186420533724,-1.33873894491981,
3.11463611845345));
#147952=CARTESIAN_POINT('Ctrl Pts',(8.08476135158299,-1.33344492733438,
3.12183143591672));
#147953=CARTESIAN_POINT('Ctrl Pts',(8.08848479065032,-1.32768940218083,
3.12815998737018));
#147954=CARTESIAN_POINT('Ctrl Pts',(8.29800821672472,-1.00000000020416,
3.48468931635154));
#147955=CARTESIAN_POINT('Ctrl Pts',(8.22903739841269,-1.10901473827415,
3.3673726241933));
#147956=CARTESIAN_POINT('Ctrl Pts',(8.15922391772688,-1.21834403198615,
3.2483918998115));
#147957=CARTESIAN_POINT('Ctrl Pts',(8.0884847908968,-1.32768940204711,3.12815998710355));
#147958=CARTESIAN_POINT('',(7.850667698,-1.32768940200002,3.684560736));
#147959=CARTESIAN_POINT('Ctrl Pts',(7.85066769785711,-1.32768940157742,
3.68456073683881));
#147960=CARTESIAN_POINT('Ctrl Pts',(7.98645612010734,-1.21834383433082,
3.65260277261618));
#147961=CARTESIAN_POINT('Ctrl Pts',(8.12070012204856,-1.109014654343,3.62084049699315));
#147962=CARTESIAN_POINT('Ctrl Pts',(8.25315907913426,-1.00000000012426,
3.58961909013581));
#147963=CARTESIAN_POINT('',(7.77551683,-1.32768940200002,3.840613121));
#147964=CARTESIAN_POINT('Ctrl Pts',(7.85066769791922,-1.32768940194829,
3.68456073583356));
#147965=CARTESIAN_POINT('Ctrl Pts',(7.84502166401928,-1.3322359514189,3.68588953652913));
#147966=CARTESIAN_POINT('Ctrl Pts',(7.83933226760092,-1.33650155471162,
3.68796682397788));
#147967=CARTESIAN_POINT('Ctrl Pts',(7.82372789202242,-1.34730670105384,
3.69573532823493));
#147968=CARTESIAN_POINT('Ctrl Pts',(7.81412584082864,-1.35293307627325,
3.70288311945405));
#147969=CARTESIAN_POINT('Ctrl Pts',(7.80058364644547,-1.35917045599075,
3.71683649680359));
#147970=CARTESIAN_POINT('Ctrl Pts',(7.79605901857717,-1.36087898843652,
3.7223549730541));
#147971=CARTESIAN_POINT('Ctrl Pts',(7.78783487297178,-1.36317274230327,
3.73422868326695));
#147972=CARTESIAN_POINT('Ctrl Pts',(7.78416154785463,-1.36375173587338,
3.74054360906622));
#147973=CARTESIAN_POINT('Ctrl Pts',(7.78099082211099,-1.36375173587283,
3.74712768891714));
#147974=CARTESIAN_POINT('Ctrl Pts',(7.7754138253233,-1.36375173587187,3.75870844207817));
#147975=CARTESIAN_POINT('Ctrl Pts',(7.77148176637241,-1.36196031891213,
3.77093381386658));
#147976=CARTESIAN_POINT('Ctrl Pts',(7.76730846475425,-1.3549908652122,3.7954242649276));
#147977=CARTESIAN_POINT('Ctrl Pts',(7.76713645006289,-1.3498599671305,3.80743986883125));
#147978=CARTESIAN_POINT('Ctrl Pts',(7.77013516735406,-1.33873894479117,
3.82655023058136));
#147979=CARTESIAN_POINT('Ctrl Pts',(7.77237566726015,-1.33344492719834,
3.83397628000857));
#147980=CARTESIAN_POINT('Ctrl Pts',(7.77551682988422,-1.32768940203628,
3.84061312108624));
#147981=CARTESIAN_POINT('Ctrl Pts',(7.95223773319059,-1.00000000030882,
4.2144887031835));
#147982=CARTESIAN_POINT('Ctrl Pts',(7.8940607583389,-1.10901473835463,4.09146179706751));
#147983=CARTESIAN_POINT('Ctrl Pts',(7.83519367612302,-1.21834403204217,
3.96670202196033));
#147984=CARTESIAN_POINT('Ctrl Pts',(7.77551682979918,-1.32768940207848,
3.8406131211631));
#147985=CARTESIAN_POINT('',(7.488781739,-1.32768940200002,4.373456205));
#147986=CARTESIAN_POINT('Ctrl Pts',(7.48878173910531,-1.32768940203771,
4.3734562055302));
#147987=CARTESIAN_POINT('Ctrl Pts',(7.62688820723029,-1.2183438345691,4.3537988749128));
#147988=CARTESIAN_POINT('Ctrl Pts',(7.76343893103024,-1.1090146543582,4.33419800434109));
#147989=CARTESIAN_POINT('Ctrl Pts',(7.89816331292909,-0.999999999917447,
4.3149758149713));
#147990=CARTESIAN_POINT('',(7.399944978,-1.32768940200002,4.522143898));
#147991=CARTESIAN_POINT('Ctrl Pts',(7.48878173912938,-1.32768940209639,
4.37345620537261));
#147992=CARTESIAN_POINT('Ctrl Pts',(7.48303932181701,-1.33223595148124,
4.37427355014363));
#147993=CARTESIAN_POINT('Ctrl Pts',(7.47718662272123,-1.33650155469588,
4.37583248146923));
#147994=CARTESIAN_POINT('Ctrl Pts',(7.46094870251594,-1.34730670096865,
4.38217094653701));
#147995=CARTESIAN_POINT('Ctrl Pts',(7.45074458329346,-1.35293307618431,
4.38842924161994));
#147996=CARTESIAN_POINT('Ctrl Pts',(7.43600613470365,-1.35917045589565,
4.40111253383242));
#147997=CARTESIAN_POINT('Ctrl Pts',(7.43100504926068,-1.36087898833917,
4.40620320980585));
#147998=CARTESIAN_POINT('Ctrl Pts',(7.42174966047235,-1.3631727422014,4.41729191322548));
#147999=CARTESIAN_POINT('Ctrl Pts',(7.41752505749903,-1.36375173576924,
4.42325214266577));
#148000=CARTESIAN_POINT('Ctrl Pts',(7.41377690379883,-1.36375173576648,
4.42952549528285));
#148001=CARTESIAN_POINT('Ctrl Pts',(7.4071842676527,-1.36375173576164,4.44055970959978));
#148002=CARTESIAN_POINT('Ctrl Pts',(7.4021721641394,-1.36196031879803,4.45238339858913));
#148003=CARTESIAN_POINT('Ctrl Pts',(7.39582035590394,-1.3549908650908,4.47640116642154));
#148004=CARTESIAN_POINT('Ctrl Pts',(7.39457196326603,-1.34985996700553,
4.48835297975807));
#148005=CARTESIAN_POINT('Ctrl Pts',(7.39584556898714,-1.33873894466817,
4.5076552117413));
#148006=CARTESIAN_POINT('Ctrl Pts',(7.39741138335892,-1.33344492708259,
4.51525220292776));
#148007=CARTESIAN_POINT('Ctrl Pts',(7.39994497873345,-1.32768940192929,
4.52214389767129));
#148008=CARTESIAN_POINT('Ctrl Pts',(7.54244050677706,-1.00000000021305,
4.91035550626368));
#148009=CARTESIAN_POINT('Ctrl Pts',(7.49552578212922,-1.10901473827983,
4.78260892651342));
#148010=CARTESIAN_POINT('Ctrl Pts',(7.44807906146581,-1.21834403198914,
4.65307459304683));
#148011=CARTESIAN_POINT('Ctrl Pts',(7.39994497847541,-1.32768940204821,
4.52214389786548));
#148012=CARTESIAN_POINT('',(7.066600514,-1.32768940200002,5.027139175));
#148013=CARTESIAN_POINT('Ctrl Pts',(7.06660051407375,-1.32768940204712,
5.02713917571187));
#148014=CARTESIAN_POINT('Ctrl Pts',(7.20591307568901,-1.21834383453908,
5.01994074814748));
#148015=CARTESIAN_POINT('Ctrl Pts',(7.34367109490997,-1.10901465428964,
5.01265909749143));
#148016=CARTESIAN_POINT('Ctrl Pts',(7.47957617982504,-0.999999999810885,
5.00559089155299));
#148017=CARTESIAN_POINT('',(6.964793122,-1.32768940200002,5.167265029));
#148018=CARTESIAN_POINT('Ctrl Pts',(7.06660051416282,-1.32768940218437,
5.0271391753499));
#148019=CARTESIAN_POINT('Ctrl Pts',(7.06080794801293,-1.33223595147841,
5.0274384834299));
#148020=CARTESIAN_POINT('Ctrl Pts',(7.05483906874339,-1.33650155461117,
5.02846650704578));
#148021=CARTESIAN_POINT('Ctrl Pts',(7.0380983421117,-1.34730670081975,5.0333238993322));
#148022=CARTESIAN_POINT('Ctrl Pts',(7.02737431242565,-1.35293307604024,
5.03864231015989));
#148023=CARTESIAN_POINT('Ctrl Pts',(7.01155827494509,-1.35917045575939,
5.04995339881578));
#148024=CARTESIAN_POINT('Ctrl Pts',(7.00612099772445,-1.36087898820575,
5.05457528737984));
#148025=CARTESIAN_POINT('Ctrl Pts',(6.99590888469631,-1.36317274207367,
5.06478970428213));
#148026=CARTESIAN_POINT('Ctrl Pts',(6.99116701788302,-1.36375173564436,
5.07034724909893));
#148027=CARTESIAN_POINT('Ctrl Pts',(6.9868716141528,-1.36375173564439,5.07625936513458));
#148028=CARTESIAN_POINT('Ctrl Pts',(6.9793164186734,-1.36375173564445,5.08665819959848));
#148029=CARTESIAN_POINT('Ctrl Pts',(6.97326462510242,-1.36196031868576,
5.09798500839568));
#148030=CARTESIAN_POINT('Ctrl Pts',(6.96478545126267,-1.35499086498787,
5.121336716054));
#148031=CARTESIAN_POINT('Ctrl Pts',(6.96247073199497,-1.34985996690716,
5.13312850985036));
#148032=CARTESIAN_POINT('Ctrl Pts',(6.96200897181235,-1.33873894460026,
5.15246720181947));
#148033=CARTESIAN_POINT('Ctrl Pts',(6.9628874936231,-1.33344492704721,5.16017396823523));
#148034=CARTESIAN_POINT('Ctrl Pts',(6.96479312271032,-1.32768940192987,
5.16726502875217));
#148035=CARTESIAN_POINT('Ctrl Pts',(7.07191598493006,-1.0000000000433,5.56668701305468));
#148036=CARTESIAN_POINT('Ctrl Pts',(7.03664124030446,-1.1090147382238,5.43524929978373));
#148037=CARTESIAN_POINT('Ctrl Pts',(7.00099689432893,-1.21834403204728,
5.30198334200609));
#148038=CARTESIAN_POINT('Ctrl Pts',(6.96479312204206,-1.32768940221948,
5.16726502916683));
#148039=CARTESIAN_POINT('',(6.587523177,-1.32768940200002,5.640346578));
#148040=CARTESIAN_POINT('Ctrl Pts',(6.58752317677662,-1.3276894017101,5.64034657789402));
#148041=CARTESIAN_POINT('Ctrl Pts',(6.72692016891382,-1.2183438343021,5.64566501082948));
#148042=CARTESIAN_POINT('Ctrl Pts',(6.86477633685045,-1.10901465415312,
5.6507612075996));
#148043=CARTESIAN_POINT('Ctrl Pts',(7.00076789681646,-0.999999999774394,
5.65590389407081));
#148044=CARTESIAN_POINT('',(6.473564847,-1.32768940200002,5.770782381));
#148045=CARTESIAN_POINT('Ctrl Pts',(6.58752317690416,-1.32768940185458,
5.64034657752293));
#148046=CARTESIAN_POINT('Ctrl Pts',(6.58172709993427,-1.33223595135912,
5.64012543898217));
#148047=CARTESIAN_POINT('Ctrl Pts',(6.57569009804838,-1.33650155468271,
5.64061427785487));
#148048=CARTESIAN_POINT('Ctrl Pts',(6.55858135111834,-1.34730670105205,
5.64395148859084));
#148049=CARTESIAN_POINT('Ctrl Pts',(6.5474237545518,-1.35293307627263,5.64828719444978));
#148050=CARTESIAN_POINT('Ctrl Pts',(6.53065746961772,-1.359170455992,5.65813500931785));
#148051=CARTESIAN_POINT('Ctrl Pts',(6.52482777837964,-1.36087898843847,
5.66225089774472));
#148052=CARTESIAN_POINT('Ctrl Pts',(6.51374116304361,-1.36317274230659,
5.6715087876528));
#148053=CARTESIAN_POINT('Ctrl Pts',(6.50852021111509,-1.36375173587738,
5.67661890176379));
#148054=CARTESIAN_POINT('Ctrl Pts',(6.50371214142148,-1.36375173587751,
5.6821221803364));
#148055=CARTESIAN_POINT('Ctrl Pts',(6.49525521660246,-1.36375173587774,
5.69180190964827));
#148056=CARTESIAN_POINT('Ctrl Pts',(6.48821245845978,-1.36196031891918,
5.7025406414498));
#148057=CARTESIAN_POINT('Ctrl Pts',(6.47767418834347,-1.35499086522148,
5.72503827471508));
#148058=CARTESIAN_POINT('Ctrl Pts',(6.47431177920769,-1.34985996714087,
5.73657510838082));
#148059=CARTESIAN_POINT('Ctrl Pts',(6.47211837095175,-1.33873894483526,
5.7557945565959));
#148060=CARTESIAN_POINT('Ctrl Pts',(6.47230252687583,-1.33344492728374,
5.76354904792197));
#148061=CARTESIAN_POINT('Ctrl Pts',(6.47356484669523,-1.32768940216811,
5.77078238118694));
#148062=CARTESIAN_POINT('Ctrl Pts',(6.54445255389812,-0.999999999960807,
6.17819882898586));
#148063=CARTESIAN_POINT('Ctrl Pts',(6.52110180080846,-1.10901473814172,
6.04412824156698));
#148064=CARTESIAN_POINT('Ctrl Pts',(6.49754681684949,-1.21834403196544,
5.90820363880618));
#148065=CARTESIAN_POINT('Ctrl Pts',(6.47356484676908,-1.32768940213768,
5.77078238114983));
#148066=CARTESIAN_POINT('',(6.055406976,-1.32768940200002,6.208141225));
#148067=CARTESIAN_POINT('Ctrl Pts',(6.05540697605073,-1.32768940208598,
6.20814122513386));
#148068=CARTESIAN_POINT('Ctrl Pts',(6.19376605621082,-1.21834383468118,
6.22593369766439));
#148069=CARTESIAN_POINT('Ctrl Pts',(6.33061043617276,-1.10901465453519,
6.24336671027083));
#148070=CARTESIAN_POINT('Ctrl Pts',(6.46559354722401,-1.00000000015905,
6.26067888325481));
#148071=CARTESIAN_POINT('',(5.930215234,-1.32768940200002,6.327836787));
#148072=CARTESIAN_POINT('Ctrl Pts',(6.05540697612598,-1.3276894021538,6.20814122496572));
#148073=CARTESIAN_POINT('Ctrl Pts',(6.04965405520633,-1.33223595161668,
6.20740142034682));
#148074=CARTESIAN_POINT('Ctrl Pts',(6.04359753738465,-1.33650155490257,
6.20734713862694));
#148075=CARTESIAN_POINT('Ctrl Pts',(6.02625852002746,-1.34730670124086,
6.2091372984766));
#148076=CARTESIAN_POINT('Ctrl Pts',(6.01475719098768,-1.35293307646214,
6.21245539081279));
#148077=CARTESIAN_POINT('Ctrl Pts',(5.99717565086845,-1.35917045618277,
6.22076064307861));
#148078=CARTESIAN_POINT('Ctrl Pts',(5.99100048285915,-1.36087898862972,
6.22433739265493));
#148079=CARTESIAN_POINT('Ctrl Pts',(5.97912862812348,-1.3631727424988,6.23256421648311));
#148080=CARTESIAN_POINT('Ctrl Pts',(5.97347062711498,-1.36375173607007,
6.23718575625434));
#148081=CARTESIAN_POINT('Ctrl Pts',(5.96818860320827,-1.36375173607066,
6.24223588820087));
#148082=CARTESIAN_POINT('Ctrl Pts',(5.95889803923611,-1.36375173607169,
6.25111857687207));
#148083=CARTESIAN_POINT('Ctrl Pts',(5.95092102066963,-1.36196031911392,
6.26118276972391));
#148084=CARTESIAN_POINT('Ctrl Pts',(5.93840850223206,-1.35499086541765,
6.28264519088178));
#148085=CARTESIAN_POINT('Ctrl Pts',(5.93402547536983,-1.34985996733775,
6.29383417661584));
#148086=CARTESIAN_POINT('Ctrl Pts',(5.93011807903562,-1.33873894492255,
6.31277963757132));
#148087=CARTESIAN_POINT('Ctrl Pts',(5.92960638637303,-1.33344492723105,
6.32051941938347));
#148088=CARTESIAN_POINT('Ctrl Pts',(5.93021523353628,-1.32768940195741,
6.32783678700507));
#148089=CARTESIAN_POINT('Ctrl Pts',(5.96429703904196,-0.999999999791277,
6.73996742082874));
#148090=CARTESIAN_POINT('Ctrl Pts',(5.95305828402978,-1.10901473792973,
6.60434341685274));
#148091=CARTESIAN_POINT('Ctrl Pts',(5.94178231297559,-1.21834403171087,
6.46685455414235));
#148092=CARTESIAN_POINT('Ctrl Pts',(5.93021523383119,-1.32768940184066,
6.3278367868887));
#148093=CARTESIAN_POINT('',(5.474536198,-1.32768940200002,6.725951571));
#148094=CARTESIAN_POINT('Ctrl Pts',(5.47453619793898,-1.32768940194877,
6.72595157108985));
#148095=CARTESIAN_POINT('Ctrl Pts',(5.61074338033991,-1.21834383447162,
6.75607482866063));
#148096=CARTESIAN_POINT('Ctrl Pts',(5.74547418201546,-1.10901465425249,
6.78570429670652));
#148097=CARTESIAN_POINT('Ctrl Pts',(5.87836203967684,-0.999999999803763,
6.81504656873444));
#148098=CARTESIAN_POINT('',(5.339119014,-1.32768940200002,6.833943172));
#148099=CARTESIAN_POINT('Ctrl Pts',(5.47453619794346,-1.3276894019521,6.72595157108191));
#148100=CARTESIAN_POINT('Ctrl Pts',(5.46887275217696,-1.33223595140147,
6.72469905685192));
#148101=CARTESIAN_POINT('Ctrl Pts',(5.46284548190358,-1.33650155467468,
6.72410209158784));
#148102=CARTESIAN_POINT('Ctrl Pts',(5.44541579765377,-1.34730670099757,
6.72433078725384));
#148103=CARTESIAN_POINT('Ctrl Pts',(5.43366333807954,-1.35293307621405,
6.7266045507431));
#148104=CARTESIAN_POINT('Ctrl Pts',(5.41540809900001,-1.35917045592674,
6.73330037140443));
#148105=CARTESIAN_POINT('Ctrl Pts',(5.40893717304231,-1.36087898837075,
6.73630918424745));
#148106=CARTESIAN_POINT('Ctrl Pts',(5.39637566410318,-1.36317274223397,
6.74343870445049));
#148107=CARTESIAN_POINT('Ctrl Pts',(5.39032616891342,-1.36375173580231,
6.74753445996235));
#148108=CARTESIAN_POINT('Ctrl Pts',(5.38461271854601,-1.36375173580003,
6.75209078459071));
#148109=CARTESIAN_POINT('Ctrl Pts',(5.37456331758125,-1.36375173579604,
6.76010491443722));
#148110=CARTESIAN_POINT('Ctrl Pts',(5.36571626485717,-1.36196031883328,
6.76941353737756));
#148111=CARTESIAN_POINT('Ctrl Pts',(5.35133024154627,-1.35499086512764,
6.78966794363456));
#148112=CARTESIAN_POINT('Ctrl Pts',(5.34596188651656,-1.34985996704315,
6.80041899430357));
#148113=CARTESIAN_POINT('Ctrl Pts',(5.34037196225801,-1.33873894475413,
6.81893792987469));
#148114=CARTESIAN_POINT('Ctrl Pts',(5.33916854083174,-1.33344492722887,
6.82660068560842));
#148115=CARTESIAN_POINT('Ctrl Pts',(5.33911901311749,-1.32768940214345,
6.83394317210648));
#148116=CARTESIAN_POINT('Ctrl Pts',(5.33612051055408,-1.00000000012717,
7.24746975809871));
#148117=CARTESIAN_POINT('Ctrl Pts',(5.33708424139336,-1.10901473818033,
7.11138430241068));
#148118=CARTESIAN_POINT('Ctrl Pts',(5.33817807065952,-1.21834403187569,
6.97343815934646));
#148119=CARTESIAN_POINT('Ctrl Pts',(5.33911901369835,-1.32768940192048,
6.83394317193563));
#148120=CARTESIAN_POINT('',(4.84958767583258,-1.32768940194837,7.18960850739358));
#148121=CARTESIAN_POINT('Ctrl Pts',(4.8495876755192,-1.32768940181776,7.18960850804234));
#148122=CARTESIAN_POINT('Ctrl Pts',(4.9825462995355,-1.21834383449911,7.2318200159394));
#148123=CARTESIAN_POINT('Ctrl Pts',(5.11407874926017,-1.10901465444024,
7.27340738041884));
#148124=CARTESIAN_POINT('Ctrl Pts',(5.24380141818337,-1.00000000015116,
7.31454350482227));
#148125=CARTESIAN_POINT('',(4.705035349,-1.32768940200002,7.285026664));
#148126=CARTESIAN_POINT('Ctrl Pts',(4.84958767607712,-1.32768940218148,
7.18960850722729));
#148127=CARTESIAN_POINT('Ctrl Pts',(4.84405930425442,-1.33223595156484,
7.18785336792304));
#148128=CARTESIAN_POINT('Ctrl Pts',(4.83810980963135,-1.33650155477901,
7.18671852554355));
#148129=CARTESIAN_POINT('Ctrl Pts',(4.82072979213366,-1.34730670106102,
7.1853839156919));
#148130=CARTESIAN_POINT('Ctrl Pts',(4.80882082591909,-1.35293307628648,
7.18659504331653));
#148131=CARTESIAN_POINT('Ctrl Pts',(4.79003886832668,-1.35917045601382,
7.19162752154787));
#148132=CARTESIAN_POINT('Ctrl Pts',(4.78332428450956,-1.36087898846319,
7.19404417246096));
#148133=CARTESIAN_POINT('Ctrl Pts',(4.77017425924559,-1.36317274233714,
7.20001898632598));
#148134=CARTESIAN_POINT('Ctrl Pts',(4.76378197684948,-1.36375173591085,
7.20355598095978));
#148135=CARTESIAN_POINT('Ctrl Pts',(4.75768310136027,-1.36375173591383,
7.20758181342034));
#148136=CARTESIAN_POINT('Ctrl Pts',(4.74695577526567,-1.36375173591908,
7.2146628593743));
#148137=CARTESIAN_POINT('Ctrl Pts',(4.73730991964322,-1.36196031896553,
7.22314096483992));
#148138=CARTESIAN_POINT('Ctrl Pts',(4.72116621924342,-1.35499086527729,
7.24202427961917));
#148139=CARTESIAN_POINT('Ctrl Pts',(4.71485575887476,-1.3498599672013,7.25225083408192));
#148140=CARTESIAN_POINT('Ctrl Pts',(4.70762831330155,-1.33873894475924,
7.27019414118161));
#148141=CARTESIAN_POINT('Ctrl Pts',(4.70574285233601,-1.33344492702836,
7.27771817531577));
#148142=CARTESIAN_POINT('Ctrl Pts',(4.70503534864307,-1.32768940170969,
7.28502666373681));
#148143=CARTESIAN_POINT('Ctrl Pts',(4.66498067879555,-0.999999999952129,
7.6966197299416));
#148144=CARTESIAN_POINT('Ctrl Pts',(4.67813913625212,-1.10901473800108,
7.56116850237982));
#148145=CARTESIAN_POINT('Ctrl Pts',(4.6915939591275,-1.21834403169194,7.42387573995099));
#148146=CARTESIAN_POINT('Ctrl Pts',(4.70503534858688,-1.32768940173079,
7.28502666374798));
#148147=CARTESIAN_POINT('',(4.185593123,-1.32768940200002,7.595378945));
#148148=CARTESIAN_POINT('Ctrl Pts',(4.18559312299156,-1.32768940217896,
7.59537894538274));
#148149=CARTESIAN_POINT('Ctrl Pts',(4.31423268431486,-1.21834383483831,
7.64933884133742));
#148150=CARTESIAN_POINT('Ctrl Pts',(4.44150776048922,-1.10901465475701,
7.70254926521416));
#148151=CARTESIAN_POINT('Ctrl Pts',(4.56702079035568,-1.00000000044527,
7.75514803807409));
#148152=CARTESIAN_POINT('',(4.033069504,-1.32768940200002,7.677455405));
#148153=CARTESIAN_POINT('Ctrl Pts',(4.18559312312533,-1.32768940225632,
7.5953789452207));
#148154=CARTESIAN_POINT('Ctrl Pts',(4.18024433645438,-1.33223595154869,
7.5931353122223));
#148155=CARTESIAN_POINT('Ctrl Pts',(4.17442051933056,-1.33650155468029,
7.59147172983892));
#148156=CARTESIAN_POINT('Ctrl Pts',(4.15723010228811,-1.34730670089189,
7.58858455999571));
#148157=CARTESIAN_POINT('Ctrl Pts',(4.1452605134269,-1.35293307611646,7.58872330047544));
#148158=CARTESIAN_POINT('Ctrl Pts',(4.12610305860312,-1.35917045584226,
7.59205191773052));
#148159=CARTESIAN_POINT('Ctrl Pts',(4.11919887880873,-1.36087898829106,
7.59385694926454));
#148160=CARTESIAN_POINT('Ctrl Pts',(4.10556621349489,-1.36317274216386,
7.59862895110864));
#148161=CARTESIAN_POINT('Ctrl Pts',(4.09888261079392,-1.363751735737,7.6015787070655));
#148162=CARTESIAN_POINT('Ctrl Pts',(4.09244741474498,-1.36375173573942,
7.60504163372407));
#148163=CARTESIAN_POINT('Ctrl Pts',(4.0811285336459,-1.36375173574369,7.61113258337114));
#148164=CARTESIAN_POINT('Ctrl Pts',(4.07076153788779,-1.36196031878918,
7.61871191064466));
#148165=CARTESIAN_POINT('Ctrl Pts',(4.0529901399933,-1.35499086509918,7.63607209660278));
#148166=CARTESIAN_POINT('Ctrl Pts',(4.04578838240849,-1.34985996702232,
7.64569181665736));
#148167=CARTESIAN_POINT('Ctrl Pts',(4.03698160687458,-1.33873894472513,
7.66291502582498));
#148168=CARTESIAN_POINT('Ctrl Pts',(4.03442928704495,-1.33344492717922,
7.67023975875926));
#148169=CARTESIAN_POINT('Ctrl Pts',(4.03306950367077,-1.32768940206933,
7.67745540499325));
#148170=CARTESIAN_POINT('Ctrl Pts',(3.95628116425374,-0.999999999912974,
8.08380104597694));
#148171=CARTESIAN_POINT('Ctrl Pts',(3.98152840407528,-1.10901473807425,
7.95007462013823));
#148172=CARTESIAN_POINT('Ctrl Pts',(4.00723589014992,-1.21834403187787,
7.81454063889855));
#148173=CARTESIAN_POINT('Ctrl Pts',(4.03306950377905,-1.32768940202923,
7.67745540498167));
#148174=CARTESIAN_POINT('',(3.48789863553934,-1.3276894017749,7.93999585849295));
#148175=CARTESIAN_POINT('Ctrl Pts',(3.48789863503969,-1.32768940145685,
7.93999585890388));
#148176=CARTESIAN_POINT('Ctrl Pts',(3.61118340371515,-1.21834383408035,
8.00526968952849));
#148177=CARTESIAN_POINT('Ctrl Pts',(3.73317636241191,-1.10901465396194,
8.06967475372053));
#148178=CARTESIAN_POINT('Ctrl Pts',(3.8534691962495,-0.999999999613144,
8.13331268060684));
#148179=CARTESIAN_POINT('',(3.328631754,-1.32768940200002,8.00806979));
#148180=CARTESIAN_POINT('Ctrl Pts',(3.48789863549781,-1.32768940169677,
7.93999585844058));
#148181=CARTESIAN_POINT('Ctrl Pts',(3.48277249902714,-1.3322359511742,7.93728179597329));
#148182=CARTESIAN_POINT('Ctrl Pts',(3.47712124905877,-1.33650155447281,
7.93510286764403));
#148183=CARTESIAN_POINT('Ctrl Pts',(3.46025883926026,-1.34730670081657,
7.93068638354843));
#148184=CARTESIAN_POINT('Ctrl Pts',(3.44832499984238,-1.35293307603251,
7.92975161983458));
#148185=CARTESIAN_POINT('Ctrl Pts',(3.42894629234951,-1.35917045574422,
7.93134957605619));
#148186=CARTESIAN_POINT('Ctrl Pts',(3.42190810497448,-1.36087898818788,
7.93252845516265));
#148187=CARTESIAN_POINT('Ctrl Pts',(3.40790256181813,-1.36317274205037,
7.93605922364059));
#148188=CARTESIAN_POINT('Ctrl Pts',(3.400981451253,-1.36375173561834,7.9383979912236));
#148189=CARTESIAN_POINT('Ctrl Pts',(3.39426174706129,-1.36375173561571,
7.94127013063417));
#148190=CARTESIAN_POINT('Ctrl Pts',(3.38244244393533,-1.3637517356111,7.94632194323559));
#148191=CARTESIAN_POINT('Ctrl Pts',(3.37143777699997,-1.36196031864773,
7.95294146803599));
#148192=CARTESIAN_POINT('Ctrl Pts',(3.35218176646765,-1.35499086494101,
7.96863875117293));
#148193=CARTESIAN_POINT('Ctrl Pts',(3.34414669599052,-1.34985996685599,
7.97757418449405));
#148194=CARTESIAN_POINT('Ctrl Pts',(3.33383149747034,-1.33873894463069,
7.99393862469351));
#148195=CARTESIAN_POINT('Ctrl Pts',(3.33063286857535,-1.33344492718698,
8.00100508209111));
#148196=CARTESIAN_POINT('Ctrl Pts',(3.32863175374708,-1.32768940219364,
8.0080697900861));
#148197=CARTESIAN_POINT('Ctrl Pts',(3.21572799953932,-1.00000000015765,
8.4058963490006));
#148198=CARTESIAN_POINT('Ctrl Pts',(3.25286074564109,-1.10901473828874,
8.27497141166348));
#148199=CARTESIAN_POINT('Ctrl Pts',(3.29061391319593,-1.21834403206225,
8.14228745177371));
#148200=CARTESIAN_POINT('Ctrl Pts',(3.32863175377034,-1.32768940218508,
8.00806979008571));
#148201=CARTESIAN_POINT('',(2.76212164,-1.32768940200002,8.220684592));
#148202=CARTESIAN_POINT('Ctrl Pts',(2.76212164018736,-1.3276894021635,8.22068459194698));
#148203=CARTESIAN_POINT('Ctrl Pts',(2.87905899951266,-1.21834383472095,
8.29674681085366));
#148204=CARTESIAN_POINT('Ctrl Pts',(2.99478762493089,-1.10901465453746,
8.37182796377343));
#148205=CARTESIAN_POINT('Ctrl Pts',(3.10889173535243,-1.00000000012429,
8.44599266964046));
#148206=CARTESIAN_POINT('',(2.59739382,-1.32768940200002,8.274207905));
#148207=CARTESIAN_POINT('Ctrl Pts',(2.76212164024878,-1.32768940219308,
8.22068459189514));
#148208=CARTESIAN_POINT('Ctrl Pts',(2.7572594268428,-1.33223595159149,8.21752195217762));
#148209=CARTESIAN_POINT('Ctrl Pts',(2.75182624485655,-1.33650155481904,
8.21484522147967));
#148210=CARTESIAN_POINT('Ctrl Pts',(2.73542760884484,-1.34730670110944,
8.20893498211433));
#148211=CARTESIAN_POINT('Ctrl Pts',(2.72362560313124,-1.35293307633198,
8.20693424036016));
#148212=CARTESIAN_POINT('Ctrl Pts',(2.7041816689267,-1.3591704560546,8.20678866972344));
#148213=CARTESIAN_POINT('Ctrl Pts',(2.69706614131622,-1.36087898850225,
8.20733190475376));
#148214=CARTESIAN_POINT('Ctrl Pts',(2.68280048471137,-1.36317274237276,
8.20959301218039));
#148215=CARTESIAN_POINT('Ctrl Pts',(2.67569759099157,-1.36375173594474,
8.21130196100192));
#148216=CARTESIAN_POINT('Ctrl Pts',(2.66874748175985,-1.36375173594604,
8.21356018838122));
#148217=CARTESIAN_POINT('Ctrl Pts',(2.65652291868142,-1.36375173594831,
8.21753218970139));
#148218=CARTESIAN_POINT('Ctrl Pts',(2.64496918366811,-1.36196031899179,
8.22313861549781));
#148219=CARTESIAN_POINT('Ctrl Pts',(2.62438359855294,-1.35499086529792,
8.23704661050358));
#148220=CARTESIAN_POINT('Ctrl Pts',(2.61557990883475,-1.34985996721918,
8.24522581422891));
#148221=CARTESIAN_POINT('Ctrl Pts',(2.60383933905131,-1.33873894490892,
8.26059972886249));
#148222=CARTESIAN_POINT('Ctrl Pts',(2.60002015447877,-1.33344492734899,
8.26735101603766));
#148223=CARTESIAN_POINT('Ctrl Pts',(2.59739381999828,-1.32768940222356,
8.27420790518699));
#148224=CARTESIAN_POINT('Ctrl Pts',(2.44928368525819,-0.999999999982718,
8.66031231708415));
#148225=CARTESIAN_POINT('Ctrl Pts',(2.49800296686794,-1.10901473814178,
8.53324299868092));
#148226=CARTESIAN_POINT('Ctrl Pts',(2.54749784986341,-1.21834403194323,
8.40447735317845));
#148227=CARTESIAN_POINT('Ctrl Pts',(2.59739382035255,-1.32768940209275,
8.27420790521288));
#148228=CARTESIAN_POINT('',(2.0141056646537,-1.3276894019719,8.43518520740466));
#148229=CARTESIAN_POINT('Ctrl Pts',(2.01410566413619,-1.32768940192452,
8.43518520800257));
#148230=CARTESIAN_POINT('Ctrl Pts',(2.12375410335396,-1.21834383447808,
8.52142340685227));
#148231=CARTESIAN_POINT('Ctrl Pts',(2.23228661674759,-1.10901465429013,
8.606576139125));
#148232=CARTESIAN_POINT('Ctrl Pts',(2.33928330464296,-0.999999999872262,
8.69067049328867));
#148233=CARTESIAN_POINT('',(1.845243197,-1.32768940200002,8.473726964));
#148234=CARTESIAN_POINT('Ctrl Pts',(2.01410566493824,-1.32768940228522,
8.43518520744022));
#148235=CARTESIAN_POINT('Ctrl Pts',(2.00954652218687,-1.33223595171976,
8.43159945409989));
#148236=CARTESIAN_POINT('Ctrl Pts',(2.00437515284886,-1.33650155497982,
8.42844647242926));
#148237=CARTESIAN_POINT('Ctrl Pts',(1.98857232265249,-1.34730670129488,
8.42109006353587));
#148238=CARTESIAN_POINT('Ctrl Pts',(1.97699717345129,-1.35293307651467,
8.41803945254678));
#148239=CARTESIAN_POINT('Ctrl Pts',(1.95764456366011,-1.3591704562329,8.41615152711446));
#148240=CARTESIAN_POINT('Ctrl Pts',(1.95050898585904,-1.36087898867897,
8.41605474426427));
#148241=CARTESIAN_POINT('Ctrl Pts',(1.93609807448668,-1.3631727425463,8.41702798554097));
#148242=CARTESIAN_POINT('Ctrl Pts',(1.92887058593775,-1.36375173611669,
8.41809335615413));
#148243=CARTESIAN_POINT('Ctrl Pts',(1.92174602986137,-1.36375173611642,
8.41971948958691));
#148244=CARTESIAN_POINT('Ctrl Pts',(1.90921463182692,-1.36375173611594,
8.422579699414));
#148245=CARTESIAN_POINT('Ctrl Pts',(1.89720485262119,-1.36196031915664,
8.42712788656892));
#148246=CARTESIAN_POINT('Ctrl Pts',(1.87545543596194,-1.3549908654575,8.43913461445686));
#148247=CARTESIAN_POINT('Ctrl Pts',(1.8659540091429,-1.34985996737619,8.4464917344525));
#148248=CARTESIAN_POINT('Ctrl Pts',(1.85288259622497,-1.3387389449445,8.46075134181751));
#148249=CARTESIAN_POINT('Ctrl Pts',(1.8484736057682,-1.33344492723396,8.4671331014014));
#148250=CARTESIAN_POINT('Ctrl Pts',(1.84524319731389,-1.32768940193907,
8.47372696410058));
#148251=CARTESIAN_POINT('Ctrl Pts',(1.66311917770952,-0.999999999928505,
8.84500054279377));
#148252=CARTESIAN_POINT('Ctrl Pts',(1.7230327356253,-1.10901473804792,8.72280993090161));
#148253=CARTESIAN_POINT('Ctrl Pts',(1.78387083017168,-1.21834403180964,
8.59899934519942));
#148254=CARTESIAN_POINT('Ctrl Pts',(1.84524319736451,-1.32768940192018,
8.47372696410889));
#148255=CARTESIAN_POINT('',(1.249873295,-1.32768940200002,8.581770672));
#148256=CARTESIAN_POINT('Ctrl Pts',(1.24987329474725,-1.32768940183712,
8.58177067208187));
#148257=CARTESIAN_POINT('Ctrl Pts',(1.35134998891948,-1.21834383452832,
8.67749051148483));
#148258=CARTESIAN_POINT('Ctrl Pts',(1.45181255013311,-1.10901465447807,
8.7720292232633));
#148259=CARTESIAN_POINT('Ctrl Pts',(1.55084034091679,-1.00000000019697,
8.86537614731829));
#148260=CARTESIAN_POINT('',(1.078235761,-1.32768940200002,8.605020555));
#148261=CARTESIAN_POINT('Ctrl Pts',(1.24987329478272,-1.32768940185216,
8.5817706720615));
#148262=CARTESIAN_POINT('Ctrl Pts',(1.24565393021003,-1.33223595135743,
8.57779067543879));
#148263=CARTESIAN_POINT('Ctrl Pts',(1.24078601032253,-1.33650155468153,
8.5741868287156));
#148264=CARTESIAN_POINT('Ctrl Pts',(1.22570622100733,-1.34730670104963,
8.56544347974055));
#148265=CARTESIAN_POINT('Ctrl Pts',(1.21445112461428,-1.3529330762685,8.56136756123979));
#148266=CARTESIAN_POINT('Ctrl Pts',(1.19534565507141,-1.35917045598511,
8.55775248147335));
#148267=CARTESIAN_POINT('Ctrl Pts',(1.18824747855661,-1.36087898843056,
8.55701645997985));
#148268=CARTESIAN_POINT('Ctrl Pts',(1.17380734060152,-1.36317274229666,
8.55669399913736));
#148269=CARTESIAN_POINT('Ctrl Pts',(1.1665134487113,-1.36375173586643,8.55710721380306));
#148270=CARTESIAN_POINT('Ctrl Pts',(1.15927180852621,-1.36375173586557,
8.55808816061781));
#148271=CARTESIAN_POINT('Ctrl Pts',(1.14653447098409,-1.36375173586405,
8.55981355022169));
#148272=CARTESIAN_POINT('Ctrl Pts',(1.1341653432657,-1.36196031890375,8.56326687940421));
#148273=CARTESIAN_POINT('Ctrl Pts',(1.11142720857434,-1.35499086520276,
8.5732756690572));
#148274=CARTESIAN_POINT('Ctrl Pts',(1.10130454455473,-1.34985996712054,
8.57975147011711));
#148275=CARTESIAN_POINT('Ctrl Pts',(1.08700753210465,-1.33873894480506,
8.59278195993714));
#148276=CARTESIAN_POINT('Ctrl Pts',(1.0820442345278,-1.33344492724318,8.59874280941312));
#148277=CARTESIAN_POINT('Ctrl Pts',(1.07823576149092,-1.32768940211611,
8.60502055540426));
#148278=CARTESIAN_POINT('Ctrl Pts',(0.863564212198985,-0.999999999788603,
8.9584740249227));
#148279=CARTESIAN_POINT('Ctrl Pts',(0.934189657823288,-1.10901473803966,
8.84214592630361));
#148280=CARTESIAN_POINT('Ctrl Pts',(1.00588113150084,-1.2183440319341,8.72428725023411));
#148281=CARTESIAN_POINT('Ctrl Pts',(1.07823576132974,-1.32768940217741,
8.60502055536268));
#148282=CARTESIAN_POINT('',(0.475577681,-1.32768940200002,8.659260764));
#148283=CARTESIAN_POINT('Ctrl Pts',(0.475577680456158,-1.32768940202431,
8.65926076450709));
#148284=CARTESIAN_POINT('Ctrl Pts',(0.568065599076004,-1.21834383457737,
8.76369156484591));
#148285=CARTESIAN_POINT('Ctrl Pts',(0.659649342801168,-1.10901465438963,
8.86685508625391));
#148286=CARTESIAN_POINT('Ctrl Pts',(0.749910923085495,-0.999999999972138,
8.96870300589438));
#148287=CARTESIAN_POINT('',(0.302547006,-1.32768940200002,8.667031581));
#148288=CARTESIAN_POINT('Ctrl Pts',(0.475577681121856,-1.32768940229424,
8.6592607642002));
#148289=CARTESIAN_POINT('Ctrl Pts',(0.471732066689365,-1.33223595165813,
8.65491856908753));
#148290=CARTESIAN_POINT('Ctrl Pts',(0.467206790057779,-1.33650155485448,
8.65089287353958));
#148291=CARTESIAN_POINT('Ctrl Pts',(0.452971455449953,-1.34730670111979,
8.64083298092142));
#148292=CARTESIAN_POINT('Ctrl Pts',(0.442127031285838,-1.35293307634352,
8.63576457180456));
#148293=CARTESIAN_POINT('Ctrl Pts',(0.423422528000211,-1.35917045606807,
8.63045144419511));
#148294=CARTESIAN_POINT('Ctrl Pts',(0.416418903115651,-1.36087898851643,
8.62908211006862));
#148295=CARTESIAN_POINT('Ctrl Pts',(0.402065802077876,-1.36317274238836,
8.62746654336826));
#148296=CARTESIAN_POINT('Ctrl Pts',(0.394764232974746,-1.36375173596106,
8.62722427512315));
#148297=CARTESIAN_POINT('Ctrl Pts',(0.387463814108889,-1.36375173596304,
8.62755213731119));
#148298=CARTESIAN_POINT('Ctrl Pts',(0.374623090611254,-1.36375173596654,
8.62812881486619));
#148299=CARTESIAN_POINT('Ctrl Pts',(0.361994203322082,-1.36196031901124,
8.63045948189726));
#148300=CARTESIAN_POINT('Ctrl Pts',(0.338450424685213,-1.35499086531967,
8.63838974842051));
#148301=CARTESIAN_POINT('Ctrl Pts',(0.327788025201015,-1.34985996724206,
8.64393209119936));
#148302=CARTESIAN_POINT('Ctrl Pts',(0.312380524047815,-1.33873894481487,
8.65562854990332));
#148303=CARTESIAN_POINT('Ctrl Pts',(0.306902880703474,-1.33344492710504,
8.66112049633992));
#148304=CARTESIAN_POINT('Ctrl Pts',(0.302547006590515,-1.32768940181038,
8.66703158125051));
#148305=CARTESIAN_POINT('Ctrl Pts',(0.0570563368422528,-1.00000000016179,
8.99981914104469));
#148306=CARTESIAN_POINT('Ctrl Pts',(0.13782503550806,-1.10901473824052,
8.89029016145374));
#148307=CARTESIAN_POINT('Ctrl Pts',(0.219792670612582,-1.21834403196144,
8.77933232408725));
#148308=CARTESIAN_POINT('Ctrl Pts',(0.302547006027248,-1.32768940203058,
8.66703158104984));
#148309=CARTESIAN_POINT('',(-0.302547007,-1.32768940200002,8.667031581));
#148310=CARTESIAN_POINT('Ctrl Pts',(-0.302547007479097,-1.32768940183626,
8.6670315811936));
#148311=CARTESIAN_POINT('Ctrl Pts',(-0.219792522734839,-1.21834383445799,
8.77933252688754));
#148312=CARTESIAN_POINT('Ctrl Pts',(-0.137824974935764,-1.10901465433772,
8.89029024572902));
#148313=CARTESIAN_POINT('Ctrl Pts',(-0.057056338302778,-0.999999999986948,
8.99981914121027));
#148314=CARTESIAN_POINT('',(-0.475577681,-1.32768940200002,8.659260764));
#148315=CARTESIAN_POINT('Ctrl Pts',(-0.302547006808484,-1.32768940209839,
8.66703158095471));
#148316=CARTESIAN_POINT('Ctrl Pts',(-0.305987908599572,-1.33223595155284,
8.6623621479303));
#148317=CARTESIAN_POINT('Ctrl Pts',(-0.310134107298285,-1.33650155483069,
8.65794701589456));
#148318=CARTESIAN_POINT('Ctrl Pts',(-0.323410372907654,-1.34730670115792,
8.64665157582216));
#148319=CARTESIAN_POINT('Ctrl Pts',(-0.333756811921427,-1.35293307637481,
8.64063148394742));
#148320=CARTESIAN_POINT('Ctrl Pts',(-0.35190975129218,-1.35917045608826,
8.63366308668714));
#148321=CARTESIAN_POINT('Ctrl Pts',(-0.358762435478124,-1.36087898853258,
8.63167146500544));
#148322=CARTESIAN_POINT('Ctrl Pts',(-0.372912936869241,-1.3631727423964,
8.62877580004926));
#148323=CARTESIAN_POINT('Ctrl Pts',(-0.380163395243697,-1.36375173596503,
8.6278799994992));
#148324=CARTESIAN_POINT('Ctrl Pts',(-0.387463814108889,-1.36375173596304,
8.62755213731119));
#148325=CARTESIAN_POINT('Ctrl Pts',(-0.400304537606773,-1.36375173595955,
8.62697545975618));
#148326=CARTESIAN_POINT('Ctrl Pts',(-0.413091504089375,-1.36196031899726,
8.62816469948271));
#148327=CARTESIAN_POINT('Ctrl Pts',(-0.437251366001838,-1.35499086529249,
8.63395259304714));
#148328=CARTESIAN_POINT('Ctrl Pts',(-0.448367653573954,-1.34985996720843,
8.63851685386684));
#148329=CARTESIAN_POINT('Ctrl Pts',(-0.464761590912138,-1.33873894491584,
8.64878510818524));
#148330=CARTESIAN_POINT('Ctrl Pts',(-0.470709476999125,-1.33344492738548,
8.65376393332434));
#148331=CARTESIAN_POINT('Ctrl Pts',(-0.475577681121838,-1.32768940229425,
8.65926076420018));
#148332=CARTESIAN_POINT('Ctrl Pts',(-0.749910923381223,-1.00000000008659,
8.9687030057548));
#148333=CARTESIAN_POINT('Ctrl Pts',(-0.659649273775829,-1.10901473822727,
8.86685500789799));
#148334=CARTESIAN_POINT('Ctrl Pts',(-0.568065432473346,-1.21834403201054,
8.76369137626223));
#148335=CARTESIAN_POINT('Ctrl Pts',(-0.475577680748764,-1.32768940214297,
8.65926076437218));
#148336=CARTESIAN_POINT('',(-1.07823576159075,-1.32768940191118,8.60502055527694));
#148337=CARTESIAN_POINT('Ctrl Pts',(-1.07823576225904,-1.32768940182398,
8.60502055560243));
#148338=CARTESIAN_POINT('Ctrl Pts',(-1.00588100192119,-1.21834383435451,
8.72428746560446));
#148339=CARTESIAN_POINT('Ctrl Pts',(-0.934189604625298,-1.10901465414413,
8.8421460157062));
#148340=CARTESIAN_POINT('Ctrl Pts',(-0.86356421329429,-0.999999999704432,
8.95847402490167));
#148341=CARTESIAN_POINT('',(-1.249873295,-1.32768940200002,8.581770672));
#148342=CARTESIAN_POINT('Ctrl Pts',(-1.07823576149091,-1.32768940211609,
8.60502055540429));
#148343=CARTESIAN_POINT('Ctrl Pts',(-1.08124424645351,-1.33223595151502,
8.60006148014486));
#148344=CARTESIAN_POINT('Ctrl Pts',(-1.08497798435395,-1.33650155474298,
8.59529245980227));
#148345=CARTESIAN_POINT('Ctrl Pts',(-1.09718828812372,-1.34730670103304,
8.58285241662335));
#148346=CARTESIAN_POINT('Ctrl Pts',(-1.10695343853787,-1.35293307625488,
8.5759291122228));
#148347=CARTESIAN_POINT('Ctrl Pts',(-1.12440865719427,-1.35917045597631,
8.5673615507366));
#148348=CARTESIAN_POINT('Ctrl Pts',(-1.13105522689638,-1.36087898842353,
8.56476367686195));
#148349=CARTESIAN_POINT('Ctrl Pts',(-1.14488919712259,-1.36317274229316,
8.56061122783271));
#148350=CARTESIAN_POINT('Ctrl Pts',(-1.15203016834083,-1.3637517358647,
8.5590691074326));
#148351=CARTESIAN_POINT('Ctrl Pts',(-1.1592718085262,-1.36375173586557,
8.55808816061781));
#148352=CARTESIAN_POINT('Ctrl Pts',(-1.17200914606821,-1.36375173586709,
8.55636277101395));
#148353=CARTESIAN_POINT('Ctrl Pts',(-1.18485123861067,-1.36196031890983,
8.55640100836933));
#148354=CARTESIAN_POINT('Ctrl Pts',(-1.20943266280315,-1.35499086521458,
8.55999992824462));
#148355=CARTESIAN_POINT('Ctrl Pts',(-1.22091333665684,-1.34985996713517,
8.56354935835334));
#148356=CARTESIAN_POINT('Ctrl Pts',(-1.23816171620794,-1.3387389447467,
8.57230673456117));
#148357=CARTESIAN_POINT('Ctrl Pts',(-1.24453195642251,-1.33344492708842,
8.57673235212775));
#148358=CARTESIAN_POINT('Ctrl Pts',(-1.2498732947827,-1.32768940185218,
8.58177067206149));
#148359=CARTESIAN_POINT('Ctrl Pts',(-1.5508403411853,-1.00000000030594,
8.86537614716069));
#148360=CARTESIAN_POINT('Ctrl Pts',(-1.4518124743483,-1.1090147383101,8.77202915141815));
#148361=CARTESIAN_POINT('Ctrl Pts',(-1.35134980606935,-1.21834403195577,
8.6774903386024));
#148362=CARTESIAN_POINT('Ctrl Pts',(-1.24987329501286,-1.32768940194995,
8.58177067192916));
#148363=CARTESIAN_POINT('',(-1.845243197,-1.32768940200002,8.473726964));
#148364=CARTESIAN_POINT('Ctrl Pts',(-1.84524319784118,-1.3276894017423,
8.47372696418715));
#148365=CARTESIAN_POINT('Ctrl Pts',(-1.78387071989928,-1.21834383431895,
8.59899957133592));
#148366=CARTESIAN_POINT('Ctrl Pts',(-1.72303269008614,-1.1090146541547,
8.72281002482354));
#148367=CARTESIAN_POINT('Ctrl Pts',(-1.66311917818115,-0.999999999760975,
8.84500054287555));
#148368=CARTESIAN_POINT('',(-2.014105665,-1.32768940200002,8.435185207));
#148369=CARTESIAN_POINT('Ctrl Pts',(-1.84524319731387,-1.32768940193905,
8.4737269641006));
#148370=CARTESIAN_POINT('Ctrl Pts',(-1.8477950429561,-1.33223595150089,
8.46851817393294));
#148371=CARTESIAN_POINT('Ctrl Pts',(-1.85108625832112,-1.33650155487643,
8.46343366240974));
#148372=CARTESIAN_POINT('Ctrl Pts',(-1.86213229025263,-1.34730670128967,
8.44994917584068));
#148373=CARTESIAN_POINT('Ctrl Pts',(-1.87123752882059,-1.35293307651039,
8.44217840129406));
#148374=CARTESIAN_POINT('Ctrl Pts',(-1.88785448760807,-1.35917045623014,
8.43208065655475));
#148375=CARTESIAN_POINT('Ctrl Pts',(-1.89424142855602,-1.36087898867676,
8.42889744704194));
#148376=CARTESIAN_POINT('Ctrl Pts',(-1.9076474846242,-1.3631727425452,8.42352164702133));
#148377=CARTESIAN_POINT('Ctrl Pts',(-1.9146214737849,-1.36375173611614,
8.42134562301972));
#148378=CARTESIAN_POINT('Ctrl Pts',(-1.92174602986137,-1.36375173611642,
8.41971948958691));
#148379=CARTESIAN_POINT('Ctrl Pts',(-1.93427742789579,-1.36375173611689,
8.41685927975983));
#148380=CARTESIAN_POINT('Ctrl Pts',(-1.94707124951948,-1.36196031915856,
8.41574620688258));
#148381=CARTESIAN_POINT('Ctrl Pts',(-1.9718763208155,-1.35499086546122,
8.41712717668837));
#148382=CARTESIAN_POINT('Ctrl Pts',(-1.98362894531338,-1.34985996738079,
8.41963319816523));
#148383=CARTESIAN_POINT('Ctrl Pts',(-2.00159289302696,-1.33873894504213,
8.42680918689579));
#148384=CARTESIAN_POINT('Ctrl Pts',(-2.00833419776163,-1.33344492744846,
8.43064596424567));
#148385=CARTESIAN_POINT('Ctrl Pts',(-2.01410566493822,-1.32768940228524,
8.43518520744021));
#148386=CARTESIAN_POINT('Ctrl Pts',(-2.33928330581808,-0.999999999832172,
8.69067049301388));
#148387=CARTESIAN_POINT('Ctrl Pts',(-2.23228653562601,-1.10901473810327,
8.60657607417562));
#148388=CARTESIAN_POINT('Ctrl Pts',(-2.12375390641409,-1.21834403201796,
8.5214232507742));
#148389=CARTESIAN_POINT('Ctrl Pts',(-2.01410566492906,-1.32768940228112,
8.43518520744663));
#148390=CARTESIAN_POINT('',(-2.59739382,-1.32768940200002,8.274207905));
#148391=CARTESIAN_POINT('Ctrl Pts',(-2.59739382005672,-1.32768940220198,
8.27420790519126));
#148392=CARTESIAN_POINT('Ctrl Pts',(-2.54749775952752,-1.21834383473538,
8.40447758822955));
#148393=CARTESIAN_POINT('Ctrl Pts',(-2.49800292915253,-1.10901465452695,
8.53324309624464));
#148394=CARTESIAN_POINT('Ctrl Pts',(-2.44928368495601,-1.00000000008884,
8.66031231705933));
#148395=CARTESIAN_POINT('',(-2.762121641,-1.32768940200002,8.220684592));
#148396=CARTESIAN_POINT('Ctrl Pts',(-2.59739381999827,-1.32768940222354,
8.27420790518701));
#148397=CARTESIAN_POINT('Ctrl Pts',(-2.59946848029277,-1.33223595162173,
8.26879133857389));
#148398=CARTESIAN_POINT('Ctrl Pts',(-2.60229067402789,-1.33650155484869,
8.26343227370457));
#148399=CARTESIAN_POINT('Ctrl Pts',(-2.61208349771735,-1.34730670113423,
8.24901191321329));
#148400=CARTESIAN_POINT('Ctrl Pts',(-2.62045551441409,-1.35293307635233,
8.24045623422956));
#148401=CARTESIAN_POINT('Ctrl Pts',(-2.63610042335359,-1.35917045606773,
8.22890960734339));
#148402=CARTESIAN_POINT('Ctrl Pts',(-2.64217631165495,-1.36087898851275,
8.22516669152494));
#148403=CARTESIAN_POINT('Ctrl Pts',(-2.65504651588519,-1.36317274237799,
8.21861082329637));
#148404=CARTESIAN_POINT('Ctrl Pts',(-2.66179737252854,-1.36375173594733,
8.21581841576039));
#148405=CARTESIAN_POINT('Ctrl Pts',(-2.66874748175985,-1.36375173594604,
8.21356018838122));
#148406=CARTESIAN_POINT('Ctrl Pts',(-2.68097204483843,-1.36375173594376,
8.20958818706101));
#148407=CARTESIAN_POINT('Ctrl Pts',(-2.6936145872141,-1.3619603189827,8.20733276576193));
#148408=CARTESIAN_POINT('Ctrl Pts',(-2.71844358976387,-1.35499086528025,
8.20648466674614));
#148409=CARTESIAN_POINT('Ctrl Pts',(-2.73037353968324,-1.34985996719732,
8.20792710258216));
#148410=CARTESIAN_POINT('Ctrl Pts',(-2.74890842063211,-1.33873894477131,
8.2134639270796));
#148411=CARTESIAN_POINT('Ctrl Pts',(-2.7559665130382,-1.33344492707015,
8.21668097286978));
#148412=CARTESIAN_POINT('Ctrl Pts',(-2.76212164068402,-1.32768940178609,
8.22068459217825));
#148413=CARTESIAN_POINT('Ctrl Pts',(-3.10889173601996,-1.00000000022005,
8.44599266929272));
#148414=CARTESIAN_POINT('Ctrl Pts',(-2.99478753806051,-1.10901473827084,
8.37182790653102));
#148415=CARTESIAN_POINT('Ctrl Pts',(-2.87905878935271,-1.21834403196374,
8.29674667337776));
#148416=CARTESIAN_POINT('Ctrl Pts',(-2.76212164114016,-1.32768940200595,
8.22068459179305));
#148417=CARTESIAN_POINT('',(-3.328631754,-1.32768940200002,8.00806979));
#148418=CARTESIAN_POINT('Ctrl Pts',(-3.32863175341881,-1.32768940231455,
8.00806979009162));
#148419=CARTESIAN_POINT('Ctrl Pts',(-3.29061384423879,-1.21834383487425,
8.14228769397692));
#148420=CARTESIAN_POINT('Ctrl Pts',(-3.25286071676859,-1.10901465469334,
8.27497151221575));
#148421=CARTESIAN_POINT('Ctrl Pts',(-3.21572799918201,-1.00000000028271,
8.40589634900339));
#148422=CARTESIAN_POINT('',(-3.487898636,-1.32768940200002,7.939995858));
#148423=CARTESIAN_POINT('Ctrl Pts',(-3.32863175374707,-1.32768940219362,
8.00806979008613));
#148424=CARTESIAN_POINT('Ctrl Pts',(-3.3302125247748,-1.33223595146223,
8.00248905800613));
#148425=CARTESIAN_POINT('Ctrl Pts',(-3.3325429742706,-1.33650155457232,
7.99689858780651));
#148426=CARTESIAN_POINT('Ctrl Pts',(-3.34100374369261,-1.3473067007662,
7.9816584576379));
#148427=CARTESIAN_POINT('Ctrl Pts',(-3.3485751319546,-1.35293307599117,
7.97238675950792));
#148428=CARTESIAN_POINT('Ctrl Pts',(-3.36312202742945,-1.35917045571755,
7.95948421711507));
#148429=CARTESIAN_POINT('Ctrl Pts',(-3.3688379436014,-1.36087898816654,
7.95521173074453));
#148430=CARTESIAN_POINT('Ctrl Pts',(-3.38106867267251,-1.36317274203975,
7.94752857829612));
#148431=CARTESIAN_POINT('Ctrl Pts',(-3.38754204286878,-1.36375173561309,
7.94414227004508));
#148432=CARTESIAN_POINT('Ctrl Pts',(-3.39426174706129,-1.36375173561571,
7.94127013063417));
#148433=CARTESIAN_POINT('Ctrl Pts',(-3.40608105018694,-1.36375173562033,
7.93621831803288));
#148434=CARTESIAN_POINT('Ctrl Pts',(-3.4184705229962,-1.3619603186662,7.93283870763021));
#148435=CARTESIAN_POINT('Ctrl Pts',(-3.44312354827155,-1.35499086497692,
7.9297683681713));
#148436=CARTESIAN_POINT('Ctrl Pts',(-3.45513477067233,-1.34985996690043,
7.93013560471274));
#148437=CARTESIAN_POINT('Ctrl Pts',(-3.47409135267749,-1.33873894453579,
7.93398868563539));
#148438=CARTESIAN_POINT('Ctrl Pts',(-3.48140940496856,-1.3334449269038,
7.93656009797619));
#148439=CARTESIAN_POINT('Ctrl Pts',(-3.48789863549779,-1.32768940169679,
7.93999585844057));
#148440=CARTESIAN_POINT('Ctrl Pts',(-3.8534691968536,-1.00000000021841,
8.13331267965086));
#148441=CARTESIAN_POINT('Ctrl Pts',(-3.73317627069964,-1.10901473822962,
8.06967470393504));
#148442=CARTESIAN_POINT('Ctrl Pts',(-3.61118318198707,-1.21834403188243,
8.00526957087236));
#148443=CARTESIAN_POINT('Ctrl Pts',(-3.48789863585382,-1.32768940188326,
7.93999585808051));
#148444=CARTESIAN_POINT('',(-4.033069504,-1.32768940200002,7.677455405));
#148445=CARTESIAN_POINT('Ctrl Pts',(-4.03306950415229,-1.327689401891,7.67745540494174));
#148446=CARTESIAN_POINT('Ctrl Pts',(-4.00723584390747,-1.2183438344254,
7.81454088623289));
#148447=CARTESIAN_POINT('Ctrl Pts',(-3.98152838506235,-1.1090146542176,
7.9500747228005));
#148448=CARTESIAN_POINT('Ctrl Pts',(-3.95628116463241,-0.999999999779801,
8.08380104593988));
#148449=CARTESIAN_POINT('',(-4.185593123,-1.32768940200002,7.595378945));
#148450=CARTESIAN_POINT('Ctrl Pts',(-4.03306950367076,-1.32768940206931,
7.67745540499327));
#148451=CARTESIAN_POINT('Ctrl Pts',(-4.03414365800827,-1.33223595145271,
7.67175543994932));
#148452=CARTESIAN_POINT('Ctrl Pts',(-4.03596359994506,-1.33650155466611,
7.66597857532337));
#148453=CARTESIAN_POINT('Ctrl Pts',(-4.04302419413378,-1.34730670093839,
7.65004137978482));
#148454=CARTESIAN_POINT('Ctrl Pts',(-4.04973399360729,-1.35293307615463,
7.64012831277831));
#148455=CARTESIAN_POINT('Ctrl Pts',(-4.06306575258347,-1.3591704558669,
7.6259737385784));
#148456=CARTESIAN_POINT('Ctrl Pts',(-4.0683756754347,-1.36087898831076,
7.62120608120941));
#148457=CARTESIAN_POINT('Ctrl Pts',(-4.0798684547153,-1.36317274217366,
7.61245750477904));
#148458=CARTESIAN_POINT('Ctrl Pts',(-4.08601221869673,-1.36375173574185,
7.60850456038226));
#148459=CARTESIAN_POINT('Ctrl Pts',(-4.09244741474498,-1.36375173573942,
7.60504163372406));
#148460=CARTESIAN_POINT('Ctrl Pts',(-4.10376629584433,-1.36375173573516,
7.59895068407684));
#148461=CARTESIAN_POINT('Ctrl Pts',(-4.11580294633933,-1.36196031877213,
7.59447409521846));
#148462=CARTESIAN_POINT('Ctrl Pts',(-4.1400815026765,-1.35499086506602,
7.58920623590949));
#148463=CARTESIAN_POINT('Ctrl Pts',(-4.15207729025624,-1.3498599669813,
7.5884953163971));
#148464=CARTESIAN_POINT('Ctrl Pts',(-4.17130294590846,-1.33873894473932,
7.59063363102621));
#148465=CARTESIAN_POINT('Ctrl Pts',(-4.17882203729309,-1.33344492727405,
7.59253870638845));
#148466=CARTESIAN_POINT('Ctrl Pts',(-4.1855931231253,-1.32768940225634,
7.59537894522069));
#148467=CARTESIAN_POINT('Ctrl Pts',(-4.5670207909907,-1.00000000006023,
7.75514803814698));
#148468=CARTESIAN_POINT('Ctrl Pts',(-4.44150766456477,-1.10901473824446,
7.7025492248208));
#148469=CARTESIAN_POINT('Ctrl Pts',(-4.314232452478,-1.21834403207158,7.64933874389548));
#148470=CARTESIAN_POINT('Ctrl Pts',(-4.18559312311081,-1.32768940224796,
7.59537894523824));
#148471=CARTESIAN_POINT('',(-4.705035349,-1.32768940200002,7.285026664));
#148472=CARTESIAN_POINT('Ctrl Pts',(-4.70503534876328,-1.32768940166456,
7.2850266637129));
#148473=CARTESIAN_POINT('Ctrl Pts',(-4.6915939350508,-1.21834383431014,
7.42387599047203));
#148474=CARTESIAN_POINT('Ctrl Pts',(-4.67813912632766,-1.10901465421366,
7.56116860636961));
#148475=CARTESIAN_POINT('Ctrl Pts',(-4.66498067897969,-0.999999999886532,
7.69661972990669));
#148476=CARTESIAN_POINT('',(-4.849587676,-1.32768940200002,7.189608507));
#148477=CARTESIAN_POINT('Ctrl Pts',(-4.70503534864306,-1.32768940170967,
7.28502666373683));
#148478=CARTESIAN_POINT('Ctrl Pts',(-4.70559423778767,-1.33223595129557,
7.27925335840597));
#148479=CARTESIAN_POINT('Ctrl Pts',(-4.70688901904333,-1.33650155469243,
7.27333661116777));
#148480=CARTESIAN_POINT('Ctrl Pts',(-4.71249259024252,-1.34730670111821,
7.25683066707283));
#148481=CARTESIAN_POINT('Ctrl Pts',(-4.71828677756059,-1.35293307633343,
7.24635604537204));
#148482=CARTESIAN_POINT('Ctrl Pts',(-4.73029606054557,-1.35917045604412,
7.23106340366536));
#148483=CARTESIAN_POINT('Ctrl Pts',(-4.7351572376969,-1.36087898848742,
7.22583896166849));
#148484=CARTESIAN_POINT('Ctrl Pts',(-4.74581953408189,-1.3631727423492,
7.21609539964255));
#148485=CARTESIAN_POINT('Ctrl Pts',(-4.75158422587188,-1.36375173591682,
7.21160764588035));
#148486=CARTESIAN_POINT('Ctrl Pts',(-4.75768310136027,-1.36375173591383,
7.20758181342034));
#148487=CARTESIAN_POINT('Ctrl Pts',(-4.76841042745518,-1.36375173590859,
7.20050076746617));
#148488=CARTESIAN_POINT('Ctrl Pts',(-4.77999734360254,-1.36196031894457,
7.19496324300642));
#148489=CARTESIAN_POINT('Ctrl Pts',(-4.80370595434182,-1.35499086523651,
7.18754027753896));
#148490=CARTESIAN_POINT('Ctrl Pts',(-4.81558972407364,-1.34985996715084,
7.18575692587118));
#148491=CARTESIAN_POINT('Ctrl Pts',(-4.83492966004746,-1.33873894484204,
7.18616325779104));
#148492=CARTESIAN_POINT('Ctrl Pts',(-4.84258925152041,-1.33344492729326,
7.18738665775673));
#148493=CARTESIAN_POINT('Ctrl Pts',(-4.84958767607709,-1.3276894021815,
7.18960850722728));
#148494=CARTESIAN_POINT('Ctrl Pts',(-5.24380141911386,-1.00000000018046,
7.31454350411914));
#148495=CARTESIAN_POINT('Ctrl Pts',(-5.11407865044419,-1.10901473830268,
7.2734073480866));
#148496=CARTESIAN_POINT('Ctrl Pts',(-4.98254606029434,-1.21834403206745,
7.23181993899048));
#148497=CARTESIAN_POINT('Ctrl Pts',(-4.84958767607749,-1.32768940218177,
7.18960850722668));
#148498=CARTESIAN_POINT('',(-5.339119013,-1.32768940200002,6.833943172));
#148499=CARTESIAN_POINT('Ctrl Pts',(-5.33911901336203,-1.3276894020463,
6.83394317203873));
#148500=CARTESIAN_POINT('Ctrl Pts',(-5.33817806862293,-1.21834383468527,
6.97343841116911));
#148501=CARTESIAN_POINT('Ctrl Pts',(-5.33708424031203,-1.10901465458379,
7.11138440702185));
#148502=CARTESIAN_POINT('Ctrl Pts',(-5.33612051020986,-1.00000000025242,
7.24746975819661));
#148503=CARTESIAN_POINT('',(-5.474536199,-1.32768940200002,6.725951571));
#148504=CARTESIAN_POINT('Ctrl Pts',(-5.33911901311747,-1.32768940214016,
6.83394317211069));
#148505=CARTESIAN_POINT('Ctrl Pts',(-5.33915813729677,-1.33223595149941,
6.82814301021648));
#148506=CARTESIAN_POINT('Ctrl Pts',(-5.33991733300375,-1.33650155469162,
6.82213401903261));
#148507=CARTESIAN_POINT('Ctrl Pts',(-5.34401876437182,-1.34730670095398,
6.80519222304139));
#148508=CARTESIAN_POINT('Ctrl Pts',(-5.34885068813799,-1.35293307617826,
6.79424038213928));
#148509=CARTESIAN_POINT('Ctrl Pts',(-5.35944080343791,-1.35917045590364,
6.77793280028018));
#148510=CARTESIAN_POINT('Ctrl Pts',(-5.36381409554641,-1.36087898835228,
6.77229363778862));
#148511=CARTESIAN_POINT('Ctrl Pts',(-5.37356006248996,-1.36317274222478,
6.76163353959512));
#148512=CARTESIAN_POINT('Ctrl Pts',(-5.37889926817801,-1.36375173579776,
6.75664710921955));
#148513=CARTESIAN_POINT('Ctrl Pts',(-5.38461271854601,-1.36375173580003,
6.75209078459071));
#148514=CARTESIAN_POINT('Ctrl Pts',(-5.39466211951056,-1.36375173580403,
6.74407665474437));
#148515=CARTESIAN_POINT('Ctrl Pts',(-5.40570601027229,-1.36196031884925,
6.73752277956918));
#148516=CARTESIAN_POINT('Ctrl Pts',(-5.42865378761812,-1.35499086515872,
6.72800447328541));
#148517=CARTESIAN_POINT('Ctrl Pts',(-5.4403298583754,-1.34985996708161,
6.72516304795477));
#148518=CARTESIAN_POINT('Ctrl Pts',(-5.4596283610753,-1.33873894460838,
6.72383412557344));
#148519=CARTESIAN_POINT('Ctrl Pts',(-5.46736678229439,-1.33344492683944,
6.72436600006063));
#148520=CARTESIAN_POINT('Ctrl Pts',(-5.47453619853397,-1.32768940147805,
6.72595157121251));
#148521=CARTESIAN_POINT('Ctrl Pts',(-5.87836203986568,-0.999999999941251,
6.81504656838998));
#148522=CARTESIAN_POINT('Ctrl Pts',(-5.74547408034092,-1.10901473795678,
6.78570427387046));
#148523=CARTESIAN_POINT('Ctrl Pts',(-5.61074313513168,-1.21834403161385,
6.75607477404509));
#148524=CARTESIAN_POINT('Ctrl Pts',(-5.47453619872126,-1.32768940161921,
6.72595157087805));
#148525=CARTESIAN_POINT('',(-5.93021523354241,-1.32768940189191,6.32783678686983));
#148526=CARTESIAN_POINT('Ctrl Pts',(-5.93021523412515,-1.32768940176286,
6.32783678671984));
#148527=CARTESIAN_POINT('Ctrl Pts',(-5.94178233414468,-1.21834383430549,
6.46685480485237));
#148528=CARTESIAN_POINT('Ctrl Pts',(-5.95305829295893,-1.10901465410688,
6.60434352087773));
#148529=CARTESIAN_POINT('Ctrl Pts',(-5.96429703934163,-0.999999999678912,
6.73996742071359));
#148530=CARTESIAN_POINT('',(-6.055406976,-1.32768940200002,6.208141225));
#148531=CARTESIAN_POINT('Ctrl Pts',(-5.93021523353202,-1.32768940199765,
6.32783678695391));
#148532=CARTESIAN_POINT('Ctrl Pts',(-5.92973427764573,-1.33223595152411,
6.32205646756782));
#148533=CARTESIAN_POINT('Ctrl Pts',(-5.92995177522349,-1.33650155486746,
6.31600361284212));
#148534=CARTESIAN_POINT('Ctrl Pts',(-5.93251804458815,-1.34730670125214,
6.29876236986105));
#148535=CARTESIAN_POINT('Ctrl Pts',(-5.93634880100404,-1.35293307647141,
6.28742148754437));
#148536=CARTESIAN_POINT('Ctrl Pts',(-5.94543448325041,-1.35917045618876,
6.27023026460104));
#148537=CARTESIAN_POINT('Ctrl Pts',(-5.94928467914374,-1.3608789886345,
6.26422178483839));
#148538=CARTESIAN_POINT('Ctrl Pts',(-5.95803584785762,-1.36317274250118,
6.25273097932687));
#148539=CARTESIAN_POINT('Ctrl Pts',(-5.9629065793017,-1.36375173607124,
6.24728602014727));
#148540=CARTESIAN_POINT('Ctrl Pts',(-5.96818860320827,-1.36375173607065,
6.24223588820087));
#148541=CARTESIAN_POINT('Ctrl Pts',(-5.97747916718048,-1.36375173606962,
6.23335319952962));
#148542=CARTESIAN_POINT('Ctrl Pts',(-5.98789111364512,-1.36196031910978,
6.22583574159617));
#148543=CARTESIAN_POINT('Ctrl Pts',(-6.00989329559083,-1.3549908654096,
6.21429873031894));
#148544=CARTESIAN_POINT('Ctrl Pts',(-6.02126765851763,-1.34985996732778,
6.21042210882142));
#148545=CARTESIAN_POINT('Ctrl Pts',(-6.0403693472299,-1.33873894496681,
6.20736863188564));
#148546=CARTESIAN_POINT('Ctrl Pts',(-6.04812429250931,-1.33344492734667,
6.20720469845112));
#148547=CARTESIAN_POINT('Ctrl Pts',(-6.05540697612596,-1.32768940215382,
6.20814122496572));
#148548=CARTESIAN_POINT('Ctrl Pts',(-6.46559354791635,-0.999999999885754,
6.26067888293268));
#148549=CARTESIAN_POINT('Ctrl Pts',(-6.33061033303081,-1.10901473812568,
6.24336669663294));
#148550=CARTESIAN_POINT('Ctrl Pts',(-6.19376580688885,-1.21834403200888,
6.22593366519494));
#148551=CARTESIAN_POINT('Ctrl Pts',(-6.05540697622249,-1.32768940224085,
6.20814122474999));
#148552=CARTESIAN_POINT('',(-6.473564847,-1.32768940200002,5.770782381));
#148553=CARTESIAN_POINT('Ctrl Pts',(-6.47356484705234,-1.32768940202094,
5.77078238100751));
#148554=CARTESIAN_POINT('Ctrl Pts',(-6.49754686040969,-1.21834383453442,
5.90820388664413));
#148555=CARTESIAN_POINT('Ctrl Pts',(-6.52110181902666,-1.10901465430655,
6.04412834439049));
#148556=CARTESIAN_POINT('Ctrl Pts',(-6.54445255418411,-0.999999999849286,
6.17819882884537));
#148557=CARTESIAN_POINT('',(-6.587523177,-1.32768940200002,5.640346578));
#148558=CARTESIAN_POINT('Ctrl Pts',(-6.47356484669524,-1.32768940216809,
5.77078238118696));
#148559=CARTESIAN_POINT('Ctrl Pts',(-6.47256768322408,-1.33223595155632,
5.76506844435758));
#148560=CARTESIAN_POINT('Ctrl Pts',(-6.47224173153327,-1.33650155477443,
5.75902046047074));
#148561=CARTESIAN_POINT('Ctrl Pts',(-6.47325217673578,-1.3473067010545,
5.74161858722323));
#148562=CARTESIAN_POINT('Ctrl Pts',(-6.47605092279891,-1.35293307627464,
5.72997997360681));
#148563=CARTESIAN_POINT('Ctrl Pts',(-6.48355901941539,-1.3591704559933,
5.71204352319526));
#148564=CARTESIAN_POINT('Ctrl Pts',(-6.48685511957833,-1.3608789884395,
5.70571410290666));
#148565=CARTESIAN_POINT('Ctrl Pts',(-6.49454103079465,-1.36317274230711,
5.69348510728424));
#148566=CARTESIAN_POINT('Ctrl Pts',(-6.49890407172791,-1.36375173587764,
5.68762545890897));
#148567=CARTESIAN_POINT('Ctrl Pts',(-6.50371214142148,-1.36375173587751,
5.6821221803364));
#148568=CARTESIAN_POINT('Ctrl Pts',(-6.51216906624052,-1.36375173587729,
5.67244245102451));
#148569=CARTESIAN_POINT('Ctrl Pts',(-6.52186523753564,-1.36196031891828,
5.6640219364811));
#148570=CARTESIAN_POINT('Ctrl Pts',(-6.54274467544731,-1.35499086521973,
5.65055910943509));
#148571=CARTESIAN_POINT('Ctrl Pts',(-6.55372575086093,-1.34985996713871,
5.64567850404374));
#148572=CARTESIAN_POINT('Ctrl Pts',(-6.57247683027915,-1.33873894474862,
5.64092505731962));
#148573=CARTESIAN_POINT('Ctrl Pts',(-6.58018586159814,-1.33344492709045,
5.64006663589892));
#148574=CARTESIAN_POINT('Ctrl Pts',(-6.58752317690413,-1.3276894018546,
5.64034657752293));
#148575=CARTESIAN_POINT('Ctrl Pts',(-7.00076789692398,-0.999999999893324,
5.65590389374847));
#148576=CARTESIAN_POINT('Ctrl Pts',(-6.86477623251869,-1.10901473799573,
5.65076120332883));
#148577=CARTESIAN_POINT('Ctrl Pts',(-6.72691991747828,-1.21834403174059,
5.64566500091207));
#148578=CARTESIAN_POINT('Ctrl Pts',(-6.58752317688628,-1.32768940183436,
5.64034657757489));
#148579=CARTESIAN_POINT('',(-6.964793123,-1.32768940200002,5.167265029));
#148580=CARTESIAN_POINT('Ctrl Pts',(-6.9647931225424,-1.32768940189471,
5.1672650290375));
#148581=CARTESIAN_POINT('Ctrl Pts',(-7.00099696010947,-1.21834383456653,
5.3019835847847));
#148582=CARTESIAN_POINT('Ctrl Pts',(-7.03664126779649,-1.10901465449722,
5.43524940021246));
#148583=CARTESIAN_POINT('Ctrl Pts',(-7.07191598528383,-1.00000000019748,
5.56668701235598));
#148584=CARTESIAN_POINT('',(-7.066600514,-1.32768940200002,5.027139175));
#148585=CARTESIAN_POINT('Ctrl Pts',(-6.96479312275204,-1.32768940180384,
5.16726502890744));
#148586=CARTESIAN_POINT('Ctrl Pts',(-6.96328778019254,-1.3322359512407,
5.1616634797066));
#148587=CARTESIAN_POINT('Ctrl Pts',(-6.96242100357657,-1.33650155450293,
5.155669061255));
#148588=CARTESIAN_POINT('Ctrl Pts',(-6.9618674891292,-1.34730670082041,
5.13824666716369));
#148589=CARTESIAN_POINT('Ctrl Pts',(-6.96361169098159,-1.35293307604079,
5.12640402952092));
#148590=CARTESIAN_POINT('Ctrl Pts',(-6.9694817511883,-1.35917045575974,
5.10786676539327));
#148591=CARTESIAN_POINT('Ctrl Pts',(-6.97219721736018,-1.36087898820603,
5.10126736534918));
#148592=CARTESIAN_POINT('Ctrl Pts',(-6.97875598864058,-1.36317274207381,
5.08839864029793));
#148593=CARTESIAN_POINT('Ctrl Pts',(-6.98257621042259,-1.36375173564443,
5.08217148117021));
#148594=CARTESIAN_POINT('Ctrl Pts',(-6.9868716141528,-1.36375173564439,
5.07625936513458));
#148595=CARTESIAN_POINT('Ctrl Pts',(-6.9944268096322,-1.36375173564433,
5.06586053067068));
#148596=CARTESIAN_POINT('Ctrl Pts',(-7.00332913788735,-1.36196031868552,
5.05660475654901));
#148597=CARTESIAN_POINT('Ctrl Pts',(-7.02291772280706,-1.35499086498739,
5.04132450850107));
#148598=CARTESIAN_POINT('Ctrl Pts',(-7.03341709754474,-1.34985996690657,
5.0354792149805));
#148599=CARTESIAN_POINT('Ctrl Pts',(-7.05166659470129,-1.33873894466853,
5.02906407052158));
#148600=CARTESIAN_POINT('Ctrl Pts',(-7.05926764317835,-1.33344492720299,
5.02751807262591));
#148601=CARTESIAN_POINT('Ctrl Pts',(-7.06660051416279,-1.32768940218439,
5.0271391753499));
#148602=CARTESIAN_POINT('Ctrl Pts',(-7.47957617995657,-0.999999999937531,
5.00559089112874));
#148603=CARTESIAN_POINT('Ctrl Pts',(-7.34367099065878,-1.1090147381492,
5.01265910249651));
#148604=CARTESIAN_POINT('Ctrl Pts',(-7.20591282440991,-1.2183440320037,
5.01994076071517));
#148605=CARTESIAN_POINT('Ctrl Pts',(-7.06660051417724,-1.32768940220666,
5.02713917529118));
#148606=CARTESIAN_POINT('',(-7.399944979,-1.32768940200002,4.522143897));
#148607=CARTESIAN_POINT('Ctrl Pts',(-7.39994497873908,-1.3276894021564,
4.52214389722653));
#148608=CARTESIAN_POINT('Ctrl Pts',(-7.44807914856805,-1.21834383484025,
4.65307482860847));
#148609=CARTESIAN_POINT('Ctrl Pts',(-7.49552581838299,-1.10901465478351,
4.78260902385036));
#148610=CARTESIAN_POINT('Ctrl Pts',(-7.5424405069824,-1.00000000049598,
4.9103555054297));
#148611=CARTESIAN_POINT('',(-7.488781739,-1.32768940200002,4.373456206));
#148612=CARTESIAN_POINT('Ctrl Pts',(-7.39994497860661,-1.32768940221744,
4.52214389732625));
#148613=CARTESIAN_POINT('Ctrl Pts',(-7.39794357718913,-1.33223595153308,
4.5166998362934));
#148614=CARTESIAN_POINT('Ctrl Pts',(-7.39654295448025,-1.33650155468582,
4.51080724699966));
#148615=CARTESIAN_POINT('Ctrl Pts',(-7.39442993696486,-1.34730670091578,
4.4935046071502));
#148616=CARTESIAN_POINT('Ctrl Pts',(-7.39510555131524,-1.3529330761409,
4.48155329543664));
#148617=CARTESIAN_POINT('Ctrl Pts',(-7.39929031283406,-1.35917045586763,
4.46256446874344));
#148618=CARTESIAN_POINT('Ctrl Pts',(-7.40140328167635,-1.36087898831677,
4.45574822343215));
#148619=CARTESIAN_POINT('Ctrl Pts',(-7.40678210564818,-1.36317274219025,
4.44234338035806));
#148620=CARTESIAN_POINT('Ctrl Pts',(-7.41002875009816,-1.36375173576373,
4.43579884790071));
#148621=CARTESIAN_POINT('Ctrl Pts',(-7.41377690379883,-1.36375173576648,
4.42952549528285));
#148622=CARTESIAN_POINT('Ctrl Pts',(-7.42036953994479,-1.36375173577133,
4.41849128096622));
#148623=CARTESIAN_POINT('Ctrl Pts',(-7.42840634884571,-1.36196031881741,
4.40847476931493));
#148624=CARTESIAN_POINT('Ctrl Pts',(-7.44654636500287,-1.3549908651285,
4.39150012783265));
#148625=CARTESIAN_POINT('Ctrl Pts',(-7.45647950427152,-1.34985996705218,
4.3847372090463));
#148626=CARTESIAN_POINT('Ctrl Pts',(-7.47408048527612,-1.33873894477316,
4.37671201771834));
#148627=CARTESIAN_POINT('Ctrl Pts',(-7.48151235206001,-1.3334449272496,
4.37449089080898));
#148628=CARTESIAN_POINT('Ctrl Pts',(-7.48878173904294,-1.32768940216483,
4.37345620538491));
#148629=CARTESIAN_POINT('Ctrl Pts',(-7.89816331290478,-0.999999999857505,
4.31497581514083));
#148630=CARTESIAN_POINT('Ctrl Pts',(-7.76343882751087,-1.10901473804168,
4.3341980192771));
#148631=CARTESIAN_POINT('Ctrl Pts',(-7.62688795793261,-1.21834403186849,
4.35379891056257));
#148632=CARTESIAN_POINT('Ctrl Pts',(-7.48878173899302,-1.32768940204296,
4.37345620571205));
#148633=CARTESIAN_POINT('',(-7.77551683,-1.32768940200002,3.840613121));
#148634=CARTESIAN_POINT('Ctrl Pts',(-7.77551682982721,-1.32768940206457,
3.84061312113776));
#148635=CARTESIAN_POINT('Ctrl Pts',(-7.83519378383851,-1.21834383471285,
3.96670224946581));
#148636=CARTESIAN_POINT('Ctrl Pts',(-7.89406080304461,-1.10901465462005,
4.09146189152694));
#148637=CARTESIAN_POINT('Ctrl Pts',(-7.952237733216,-1.00000000029693,4.21448870316095));
#148638=CARTESIAN_POINT('',(-7.85066769791133,-1.32768940203921,3.68456073648917));
#148639=CARTESIAN_POINT('Ctrl Pts',(-7.77551682988423,-1.32768940203625,
3.84061312108627));
#148640=CARTESIAN_POINT('Ctrl Pts',(-7.77303548357002,-1.33223595146919,
3.83537038038259));
#148641=CARTESIAN_POINT('Ctrl Pts',(-7.77111229166754,-1.33650155472793,
3.82962706364747));
#148642=CARTESIAN_POINT('Ctrl Pts',(-7.76745678383559,-1.34730670104337,
3.81258348842368));
#148643=CARTESIAN_POINT('Ctrl Pts',(-7.76705837104186,-1.35293307626466,
3.80061972757349));
#148644=CARTESIAN_POINT('Ctrl Pts',(-7.76952414064379,-1.3591704559852,
3.78133222518374));
#148645=CARTESIAN_POINT('Ctrl Pts',(-7.77101759977719,-1.36087898843209,
3.77435401500558));
#148646=CARTESIAN_POINT('Ctrl Pts',(-7.77517316931866,-1.36317274230107,
3.76052098182607));
#148647=CARTESIAN_POINT('Ctrl Pts',(-7.77782009636727,-1.36375173587229,
3.75371176876822));
#148648=CARTESIAN_POINT('Ctrl Pts',(-7.78099082211098,-1.36375173587283,
3.74712768891714));
#148649=CARTESIAN_POINT('Ctrl Pts',(-7.78656781889864,-1.36375173587379,
3.73554693575616));
#148650=CARTESIAN_POINT('Ctrl Pts',(-7.79367440078957,-1.36196031891597,
3.7248503336419));
#148651=CARTESIAN_POINT('Ctrl Pts',(-7.81021979544659,-1.35499086521966,
3.70631796856791));
#148652=CARTESIAN_POINT('Ctrl Pts',(-7.81950672345208,-1.34985996713973,
3.69869187556753));
#148653=CARTESIAN_POINT('Ctrl Pts',(-7.83631747555383,-1.33873894480565,
3.68912125148975));
#148654=CARTESIAN_POINT('Ctrl Pts',(-7.8435203236244,-1.33344492721708,
3.6862428787659));
#148655=CARTESIAN_POINT('Ctrl Pts',(-7.85066769778106,-1.32768940205954,
3.68456073586607));
#148656=CARTESIAN_POINT('Ctrl Pts',(-8.25315907915067,-1.0000000002333,
3.58961908982468));
#148657=CARTESIAN_POINT('Ctrl Pts',(-8.12070002029395,-1.10901473821362,
3.62084052066842));
#148658=CARTESIAN_POINT('Ctrl Pts',(-7.98645587500192,-1.21834403183509,
3.65260282999209));
#148659=CARTESIAN_POINT('Ctrl Pts',(-7.85066769773845,-1.32768940180501,
3.68456073655596));
#148660=CARTESIAN_POINT('',(-8.088484791,-1.32768940200002,3.128159987));
#148661=CARTESIAN_POINT('Ctrl Pts',(-8.08848479089928,-1.32768940204577,
3.12815998710086));
#148662=CARTESIAN_POINT('Ctrl Pts',(-8.15922404537986,-1.21834383466874,
3.2483921167694));
#148663=CARTESIAN_POINT('Ctrl Pts',(-8.2290374513845,-1.10901465455067,
3.3673727142875));
#148664=CARTESIAN_POINT('Ctrl Pts',(-8.29800821672838,-1.00000000020229,
3.48468931634764));
#148665=CARTESIAN_POINT('',(-8.14934469545831,-1.32768940190648,2.96599935139841));
#148666=CARTESIAN_POINT('Ctrl Pts',(-8.08848479065033,-1.32768940218081,
3.1281599873702));
#148667=CARTESIAN_POINT('Ctrl Pts',(-8.08554347786003,-1.33223595160539,
3.12316077857491));
#148668=CARTESIAN_POINT('Ctrl Pts',(-8.08311320122475,-1.33650155485665,
3.11761297634637));
#148669=CARTESIAN_POINT('Ctrl Pts',(-8.07794463509115,-1.34730670116671,
3.10096569075218));
#148670=CARTESIAN_POINT('Ctrl Pts',(-8.07647540293555,-1.35293307638893,
3.08908580593355));
#148671=CARTESIAN_POINT('Ctrl Pts',(-8.07720232768916,-1.35917045611106,
3.06965491947504));
#148672=CARTESIAN_POINT('Ctrl Pts',(-8.07806425265739,-1.36087898855854,
3.06257092887488));
#148673=CARTESIAN_POINT('Ctrl Pts',(-8.08096310956339,-1.3631727424287,
3.04842108103817));
#148674=CARTESIAN_POINT('Ctrl Pts',(-8.08298900770923,-1.36375173600051,
3.04140201115875));
#148675=CARTESIAN_POINT('Ctrl Pts',(-8.08555677667574,-1.36375173600163,
3.03456021521294));
#148676=CARTESIAN_POINT('Ctrl Pts',(-8.09007323140408,-1.3637517360036,
3.02252616462162));
#148677=CARTESIAN_POINT('Ctrl Pts',(-8.0961923682646,-1.36196031904677,
3.01123559479314));
#148678=CARTESIAN_POINT('Ctrl Pts',(-8.11100992762966,-1.35499086535231,
2.99129471782953));
#148679=CARTESIAN_POINT('Ctrl Pts',(-8.11957587148718,-1.34985996727329,
2.98286685142906));
#148680=CARTESIAN_POINT('Ctrl Pts',(-8.13546104438258,-1.33873894489342,
2.97182785162225));
#148681=CARTESIAN_POINT('Ctrl Pts',(-8.14237688063509,-1.33344492724556,
2.96831540803315));
#148682=CARTESIAN_POINT('Ctrl Pts',(-8.14934469550913,-1.327689402021,2.96599935126671));
#148683=CARTESIAN_POINT('Ctrl Pts',(-8.54170526199855,-0.99999999983659,
2.83536086241028));
#148684=CARTESIAN_POINT('Ctrl Pts',(-8.41257811164622,-1.10901473799347,
2.87833014352137));
#148685=CARTESIAN_POINT('Ctrl Pts',(-8.28172154505887,-1.21834403179278,
2.92199813961197));
#148686=CARTESIAN_POINT('Ctrl Pts',(-8.14934469551528,-1.32768940194035,
2.96599935148564));
#148687=CARTESIAN_POINT('',(-8.336329029,-1.32768940200002,2.390520747));
#148688=CARTESIAN_POINT('Ctrl Pts',(-8.33632902896119,-1.32768940187384,
2.39052074690615));
#148689=CARTESIAN_POINT('Ctrl Pts',(-8.41756103301671,-1.21834383447248,
2.50392783959535));
#148690=CARTESIAN_POINT('Ctrl Pts',(-8.49775872931061,-1.10901465432932,
2.61617143085006));
#148691=CARTESIAN_POINT('Ctrl Pts',(-8.57696801776182,-0.999999999956059,
2.72683325912717));
#148692=CARTESIAN_POINT('',(-8.382407962,-1.32768940200002,2.223557482));
#148693=CARTESIAN_POINT('Ctrl Pts',(-8.33632902867258,-1.32768940204799,
2.39052074728083));
#148694=CARTESIAN_POINT('Ctrl Pts',(-8.33295143111257,-1.33223595148368,
2.3858053210651));
#148695=CARTESIAN_POINT('Ctrl Pts',(-8.33003363689228,-1.33650155474458,
2.38049770096133));
#148696=CARTESIAN_POINT('Ctrl Pts',(-8.32339362671072,-1.34730670105808,
2.36438073912204));
#148697=CARTESIAN_POINT('Ctrl Pts',(-8.32086540459087,-1.35293307627555,
2.3526803801806));
#148698=CARTESIAN_POINT('Ctrl Pts',(-8.31984763173159,-1.35917045598988,
2.33326255572514));
#148699=CARTESIAN_POINT('Ctrl Pts',(-8.3200710828237,-1.3608789884345,2.32612982083004));
#148700=CARTESIAN_POINT('Ctrl Pts',(-8.32168988720682,-1.36317274229893,
2.31177708459179));
#148701=CARTESIAN_POINT('Ctrl Pts',(-8.32307844511106,-1.36375173586787,
2.3046046713151));
#148702=CARTESIAN_POINT('Ctrl Pts',(-8.32502258313608,-1.36375173586619,
2.29756024539374));
#148703=CARTESIAN_POINT('Ctrl Pts',(-8.32844213197043,-1.36375173586324,
2.28516978847247));
#148704=CARTESIAN_POINT('Ctrl Pts',(-8.33352455611133,-1.3619603189015,
2.27337615596146));
#148705=CARTESIAN_POINT('Ctrl Pts',(-8.34649497791398,-1.3549908651978,
2.25218731932978));
#148706=CARTESIAN_POINT('Ctrl Pts',(-8.3542709696827,-1.34985996711426,
2.24302553575725));
#148707=CARTESIAN_POINT('Ctrl Pts',(-8.36910266521966,-1.33873894473671,
2.23060703981489));
#148708=CARTESIAN_POINT('Ctrl Pts',(-8.37567580732036,-1.33344492709784,
2.2264888055179));
#148709=CARTESIAN_POINT('Ctrl Pts',(-8.38240796207933,-1.32768940188415,
2.2235574824097));
#148710=CARTESIAN_POINT('Ctrl Pts',(-8.76147865594041,-1.00000000018313,
2.05827397549611));
#148711=CARTESIAN_POINT('Ctrl Pts',(-8.63672307032885,-1.10901473824795,
2.11264514330979));
#148712=CARTESIAN_POINT('Ctrl Pts',(-8.51030766293713,-1.21834403195478,
2.16786723695558));
#148713=CARTESIAN_POINT('Ctrl Pts',(-8.38240796203887,-1.32768940201087,
2.22355748206797));
#148714=CARTESIAN_POINT('',(-8.517054046,-1.32768940200002,1.633634441));
#148715=CARTESIAN_POINT('Ctrl Pts',(-8.51705404654846,-1.32768940205777,
1.63363444058708));
#148716=CARTESIAN_POINT('Ctrl Pts',(-8.60812476791986,-1.21834383457677,
1.73930340900002));
#148717=CARTESIAN_POINT('Ctrl Pts',(-8.69806104988347,-1.10901465435411,
1.8439062745251));
#148718=CARTESIAN_POINT('Ctrl Pts',(-8.78687111490327,-0.999999999901667,
1.94702234497933));
#148719=CARTESIAN_POINT('',(-8.547981008,-1.32768940200002,1.463212837));
#148720=CARTESIAN_POINT('Ctrl Pts',(-8.51705404632891,-1.32768940220838,
1.6336344409322));
#148721=CARTESIAN_POINT('Ctrl Pts',(-8.5132673585444,-1.33223595152413,
1.62924076322205));
#148722=CARTESIAN_POINT('Ctrl Pts',(-8.50988553919814,-1.33650155467649,
1.62421605920029));
#148723=CARTESIAN_POINT('Ctrl Pts',(-8.501827546491,-1.34730670090064,1.6087591855685));
#148724=CARTESIAN_POINT('Ctrl Pts',(-8.49826069015918,-1.3529330761202,
1.59733255691655));
#148725=CARTESIAN_POINT('Ctrl Pts',(-8.49550641418745,-1.35917045583786,
1.57808413536979));
#148726=CARTESIAN_POINT('Ctrl Pts',(-8.49508959230381,-1.36087898828368,
1.57096008476704));
#148727=CARTESIAN_POINT('Ctrl Pts',(-8.49541531049769,-1.36317274215052,
1.55652001991911));
#148728=CARTESIAN_POINT('Ctrl Pts',(-8.49615534830605,-1.36375173572067,
1.54925201129861));
#148729=CARTESIAN_POINT('Ctrl Pts',(-8.4974602023311,-1.36375173572018,
1.54206167297576));
#148730=CARTESIAN_POINT('Ctrl Pts',(-8.49975531307054,-1.3637517357193,
1.52941457039706));
#148731=CARTESIAN_POINT('Ctrl Pts',(-8.50376010379714,-1.36196031875968,
1.5172128305953));
#148732=CARTESIAN_POINT('Ctrl Pts',(-8.51477895782059,-1.35499086505998,
1.49494663434249));
#148733=CARTESIAN_POINT('Ctrl Pts',(-8.52170238978373,-1.34985996697839,
1.48512469888792));
#148734=CARTESIAN_POINT('Ctrl Pts',(-8.53536119188796,-1.33873894459695,
1.4714266932106));
#148735=CARTESIAN_POINT('Ctrl Pts',(-8.54153871678395,-1.33344492695049,
1.46673582579239));
#148736=CARTESIAN_POINT('Ctrl Pts',(-8.54798100809932,-1.32768940172794,
1.46321283762611));
#148737=CARTESIAN_POINT('Ctrl Pts',(-8.91070977514109,-1.00000000032794,
1.26461507871066));
#148738=CARTESIAN_POINT('Ctrl Pts',(-8.79133021285898,-1.10901473827852,
1.32995036863205));
#148739=CARTESIAN_POINT('Ctrl Pts',(-8.6703737871565,-1.21834403187058,
1.39628194408302));
#148740=CARTESIAN_POINT('Ctrl Pts',(-8.54798100805239,-1.32768940181178,
1.46321283740334));
#148741=CARTESIAN_POINT('',(-8.629204753,-1.32768940200002,0.863595070000001));
#148742=CARTESIAN_POINT('Ctrl Pts',(-8.6292047530183,-1.32768940220178,
0.86359507020837));
#148743=CARTESIAN_POINT('Ctrl Pts',(-8.72938094365667,-1.21834383481036,
0.960675129813629));
#148744=CARTESIAN_POINT('Ctrl Pts',(-8.82833169708263,-1.10901465467741,
1.05679506871452));
#148745=CARTESIAN_POINT('Ctrl Pts',(-8.9260274921021,-1.00000000031437,
1.15153515125643));
#148746=CARTESIAN_POINT('',(-8.644730737,-1.32768940200002,0.691087263000001));
#148747=CARTESIAN_POINT('Ctrl Pts',(-8.62920475309882,-1.32768940213718,
0.863595070052577));
#148748=CARTESIAN_POINT('Ctrl Pts',(-8.62503946318526,-1.33223595143947,
0.859558516080467));
#148749=CARTESIAN_POINT('Ctrl Pts',(-8.62122084706452,-1.33650155457962,
0.85485718399984));
#148750=CARTESIAN_POINT('Ctrl Pts',(-8.6118097500053,-1.34730670079354,
0.840184848108705));
#148751=CARTESIAN_POINT('Ctrl Pts',(-8.60723297769259,-1.35293307601313,
0.829123950240993));
#148752=CARTESIAN_POINT('Ctrl Pts',(-8.60276437442064,-1.35917045573079,
0.810199908575198));
#148753=CARTESIAN_POINT('Ctrl Pts',(-8.60171063556652,-1.3608789881766,
0.803141900931399));
#148754=CARTESIAN_POINT('Ctrl Pts',(-8.60074064508077,-1.36317274204343,
0.788730770385564));
#148755=CARTESIAN_POINT('Ctrl Pts',(-8.60082620444441,-1.36375173561358,
0.781425684153338));
#148756=CARTESIAN_POINT('Ctrl Pts',(-8.60148126855249,-1.36375173561308,
0.77414732580565));
#148757=CARTESIAN_POINT('Ctrl Pts',(-8.60263346231566,-1.3637517356122,
0.76134540460328));
#148758=CARTESIAN_POINT('Ctrl Pts',(-8.60552837540853,-1.36196031865257,
0.748833798745692));
#148759=CARTESIAN_POINT('Ctrl Pts',(-8.61450694432037,-1.35499086495292,
0.72566951719315));
#148760=CARTESIAN_POINT('Ctrl Pts',(-8.6205220730753,-1.34985996687135,
0.715266510306567));
#148761=CARTESIAN_POINT('Ctrl Pts',(-8.63289800898064,-1.33873894459279,
0.700399283329012));
#148762=CARTESIAN_POINT('Ctrl Pts',(-8.63863017872564,-1.33344492707686,
0.695173550994194));
#148763=CARTESIAN_POINT('Ctrl Pts',(-8.64473073689484,-1.32768940200152,
0.691087262840884));
#148764=CARTESIAN_POINT('Ctrl Pts',(-8.98819709909128,-1.00000000022958,
0.460774243805898));
#148765=CARTESIAN_POINT('Ctrl Pts',(-8.87515473393588,-1.10901473830768,
0.53654761461009));
#148766=CARTESIAN_POINT('Ctrl Pts',(-8.76063115969153,-1.21834403202809,
0.613454609141289));
#148767=CARTESIAN_POINT('Ctrl Pts',(-8.64473073681857,-1.32768940209738,
0.69108726259199));
#148768=CARTESIAN_POINT('',(-8.671878177,-1.32768940200002,0.0866025400000026));
#148769=CARTESIAN_POINT('Ctrl Pts',(-8.67187817713732,-1.32768940195935,
0.0866025397794755));
#148770=CARTESIAN_POINT('Ctrl Pts',(-8.78035327729649,-1.21834383460799,
0.174312059059674));
#148771=CARTESIAN_POINT('Ctrl Pts',(-8.88752180893807,-1.10901465451525,
0.261175170144174));
#148772=CARTESIAN_POINT('Ctrl Pts',(-8.99331674489802,-1.00000000019189,
0.346776473370395));
#148773=CARTESIAN_POINT('',(-8.63624826494697,-1.36375173570061,3.85948676359093E-15));
#148774=CARTESIAN_POINT('Ctrl Pts',(-8.67187817702726,-1.32768940206671,
0.0866025400494883));
#148775=CARTESIAN_POINT('Ctrl Pts',(-8.66736782138124,-1.33223595142604,
0.0829556097415469));
#148776=CARTESIAN_POINT('Ctrl Pts',(-8.66314315367645,-1.33650155461798,
0.078615501910959));
#148777=CARTESIAN_POINT('Ctrl Pts',(-8.65245472483424,-1.34730670087631,
0.0648458367127613));
#148778=CARTESIAN_POINT('Ctrl Pts',(-8.64690488602001,-1.35293307609673,
0.0542397254755955));
#148779=CARTESIAN_POINT('Ctrl Pts',(-8.64075793401352,-1.35917045581577,
0.0357924289474454));
#148780=CARTESIAN_POINT('Ctrl Pts',(-8.63907576227445,-1.3608789882621,
0.0288572911901097));
#148781=CARTESIAN_POINT('Ctrl Pts',(-8.63681787290186,-1.36317274212995,
0.0145911248958308));
#148782=CARTESIAN_POINT('Ctrl Pts',(-8.63624826494697,-1.36375173570061,
0.00730777731084098));
#148783=CARTESIAN_POINT('Ctrl Pts',(-8.63624826494697,-1.36375173570061,
4.44089209850063E-15));
#148784=CARTESIAN_POINT('',(-8.50000000044506,-1.50000000044508,3.26139582858007E-15));
#148785=CARTESIAN_POINT('',(-9.,-1.00000000000002,3.32262816848293E-15));
#148786=CARTESIAN_POINT('Origin',(1.11022302462516E-15,-1.50000000000002,
2.22044604925031E-15));
#148787=CARTESIAN_POINT('',(-8.671878177,-1.32768940200002,-0.0866025400000003));
#148788=CARTESIAN_POINT('Ctrl Pts',(-8.63624826494697,-1.36375173570061,
4.44089209850061E-15));
#148789=CARTESIAN_POINT('Ctrl Pts',(-8.63624826494697,-1.36375173570061,
-0.0128536662840206));
#148790=CARTESIAN_POINT('Ctrl Pts',(-8.63800999226789,-1.36196031874185,
-0.0255744021040272));
#148791=CARTESIAN_POINT('Ctrl Pts',(-8.64487598591024,-1.35499086504381,
-0.0494502637821181));
#148792=CARTESIAN_POINT('Ctrl Pts',(-8.64993438117684,-1.34985996696303,
-0.0603505832064033));
#148793=CARTESIAN_POINT('Ctrl Pts',(-8.66092780725787,-1.33873894467796,
-0.0762673294526308));
#148794=CARTESIAN_POINT('Ctrl Pts',(-8.66616846994706,-1.33344492715271,
-0.0819858522681948));
#148795=CARTESIAN_POINT('Ctrl Pts',(-8.67187817702724,-1.32768940206672,
-0.0866025400494692));
#148796=CARTESIAN_POINT('Ctrl Pts',(-8.99331674490455,-1.00000000018596,
-0.34677647335477));
#148797=CARTESIAN_POINT('Ctrl Pts',(-8.88752172769541,-1.10901473823108,
-0.261175104387876));
#148798=CARTESIAN_POINT('Ctrl Pts',(-8.78035308155773,-1.21834403191783,
-0.174311900770753));
#148799=CARTESIAN_POINT('Ctrl Pts',(-8.67187817714367,-1.32768940195315,
-0.0866025397638889));
#148800=CARTESIAN_POINT('',(-8.644730737,-1.32768940200002,-0.691087262999999));
#148801=CARTESIAN_POINT('Ctrl Pts',(-8.64473073694086,-1.32768940194368,
-0.691087262991059));
#148802=CARTESIAN_POINT('Ctrl Pts',(-8.76063136896071,-1.2183438345599,
-0.613454469453119));
#148803=CARTESIAN_POINT('Ctrl Pts',(-8.87515482087759,-1.10901465443496,
-0.536547556821678));
#148804=CARTESIAN_POINT('Ctrl Pts',(-8.9881970992204,-1.00000000007973,
-0.460774244214113));
#148805=CARTESIAN_POINT('',(-8.629204753,-1.32768940200002,-0.863595069999998));
#148806=CARTESIAN_POINT('Ctrl Pts',(-8.64473073689486,-1.3276894020015,
-0.691087262840871));
#148807=CARTESIAN_POINT('Ctrl Pts',(-8.63991163031322,-1.33223595135028,
-0.694315206512241));
#148808=CARTESIAN_POINT('Ctrl Pts',(-8.63531492562229,-1.33650155453274,
-0.698259146043823));
#148809=CARTESIAN_POINT('Ctrl Pts',(-8.62343522198836,-1.34730670078396,
-0.71101527523258));
#148810=CARTESIAN_POINT('Ctrl Pts',(-8.61695700071149,-1.35293307600527,
-0.721081205667742));
#148811=CARTESIAN_POINT('Ctrl Pts',(-8.60918119161373,-1.35917045572572,
-0.738903230273302));
#148812=CARTESIAN_POINT('Ctrl Pts',(-8.60688413084748,-1.36087898817254,
-0.745659660492604));
#148813=CARTESIAN_POINT('Ctrl Pts',(-8.60335652178569,-1.36317274204141,
-0.759665999752388));
#148814=CARTESIAN_POINT('Ctrl Pts',(-8.6021363326606,-1.36375173561258,
-0.766868967457801));
#148815=CARTESIAN_POINT('Ctrl Pts',(-8.60148126855249,-1.36375173561307,
-0.774147325805654));
#148816=CARTESIAN_POINT('Ctrl Pts',(-8.60032907478934,-1.36375173561395,
-0.786949247007962));
#148817=CARTESIAN_POINT('Ctrl Pts',(-8.60094343194575,-1.36196031865609,
-0.799776692904937));
#148818=CARTESIAN_POINT('Ctrl Pts',(-8.60564156937475,-1.35499086495975,
-0.824171900308657));
#148819=CARTESIAN_POINT('Ctrl Pts',(-8.60970250392851,-1.3498599668798,
-0.835481769307742));
#148820=CARTESIAN_POINT('Ctrl Pts',(-8.61922490753858,-1.33873894463695,
-0.852319882468269));
#148821=CARTESIAN_POINT('Ctrl Pts',(-8.62393186837942,-1.33344492716415,
-0.858485153528086));
#148822=CARTESIAN_POINT('Ctrl Pts',(-8.6292047530988,-1.3276894021372,-0.863595070052561));
#148823=CARTESIAN_POINT('Ctrl Pts',(-8.92602749216612,-1.00000000026639,
-1.1515351511352));
#148824=CARTESIAN_POINT('Ctrl Pts',(-8.8283316221154,-1.10901473835186,
-1.0567949958371));
#148825=CARTESIAN_POINT('Ctrl Pts',(-8.72938076294725,-1.2183440320791,
-0.960674954515165));
#148826=CARTESIAN_POINT('Ctrl Pts',(-8.62920475307709,-1.32768940215461,
-0.863595070094572));
#148827=CARTESIAN_POINT('',(-8.547981008,-1.32768940200002,-1.463212838));
#148828=CARTESIAN_POINT('Ctrl Pts',(-8.54798100788837,-1.32768940187191,
-1.46321283800513));
#148829=CARTESIAN_POINT('Ctrl Pts',(-8.67037400794378,-1.21834383453906,
-1.39628182386025));
#148830=CARTESIAN_POINT('Ctrl Pts',(-8.79133030455683,-1.10901465446515,
-1.32995031896542));
#148831=CARTESIAN_POINT('Ctrl Pts',(-8.91070977524376,-1.00000000016074,
-1.26461507917722));
#148832=CARTESIAN_POINT('',(-8.517054046,-1.32768940200002,-1.633634441));
#148833=CARTESIAN_POINT('Ctrl Pts',(-8.54798100783858,-1.32768940196087,
-1.46321283776869));
#148834=CARTESIAN_POINT('Ctrl Pts',(-8.5428919508647,-1.33223595136503,
-1.46599580531845));
#148835=CARTESIAN_POINT('Ctrl Pts',(-8.53796021908521,-1.33650155459768,
-1.4695118223078));
#148836=CARTESIAN_POINT('Ctrl Pts',(-8.52498488898969,-1.34730670089114,
-1.48115171069211));
#148837=CARTESIAN_POINT('Ctrl Pts',(-8.5176304440792,-1.3529330761124,-1.49059641537225));
#148838=CARTESIAN_POINT('Ctrl Pts',(-8.50828838413339,-1.35917045583282,
-1.50764967559236));
#148839=CARTESIAN_POINT('Ctrl Pts',(-8.50539492892273,-1.36087898827965,
-1.51417299947031));
#148840=CARTESIAN_POINT('Ctrl Pts',(-8.50062600240597,-1.36317274214851,
-1.52780674088759));
#148841=CARTESIAN_POINT('Ctrl Pts',(-8.49876505635617,-1.36375173571968,
-1.53487133465274));
#148842=CARTESIAN_POINT('Ctrl Pts',(-8.49746020233109,-1.36375173572018,
-1.54206167297575));
#148843=CARTESIAN_POINT('Ctrl Pts',(-8.49516509159166,-1.36375173572105,
-1.55470877555439));
#148844=CARTESIAN_POINT('Ctrl Pts',(-8.49462713214117,-1.36196031876316,
-1.56753965247642));
#148845=CARTESIAN_POINT('Ctrl Pts',(-8.49711958671714,-1.35499086506676,
-1.59225778973971));
#148846=CARTESIAN_POINT('Ctrl Pts',(-8.50015036430106,-1.34985996698678,
-1.60388614789829));
#148847=CARTESIAN_POINT('Ctrl Pts',(-8.50812507669321,-1.33873894473423,
-1.62151005745983));
#148848=CARTESIAN_POINT('Ctrl Pts',(-8.51226043806651,-1.33344492724917,
-1.62807243767969));
#148849=CARTESIAN_POINT('Ctrl Pts',(-8.51705404632889,-1.3276894022084,
-1.63363444093218));
#148850=CARTESIAN_POINT('Ctrl Pts',(-8.78687111486193,-0.999999999752181,
-1.94702234585691));
#148851=CARTESIAN_POINT('Ctrl Pts',(-8.69806098154262,-1.10901473805156,
-1.84390619609545));
#148852=CARTESIAN_POINT('Ctrl Pts',(-8.60812460334816,-1.2183440319946,
-1.73930321896202));
#148853=CARTESIAN_POINT('Ctrl Pts',(-8.51705404621577,-1.327689402286,-1.63363444110996));
#148854=CARTESIAN_POINT('',(-8.382407962,-1.32768940200002,-2.223557482));
#148855=CARTESIAN_POINT('Ctrl Pts',(-8.38240796213464,-1.3276894017109,
-2.22355748287687));
#148856=CARTESIAN_POINT('Ctrl Pts',(-8.51030789375738,-1.21834383440846,
-2.16786713730407));
#148857=CARTESIAN_POINT('Ctrl Pts',(-8.63672316609019,-1.10901465436549,
-2.11264510242941));
#148858=CARTESIAN_POINT('Ctrl Pts',(-8.76147865582069,-1.00000000009201,
-2.05827397640414));
#148859=CARTESIAN_POINT('',(-8.336329029,-1.32768940200002,-2.390520747));
#148860=CARTESIAN_POINT('Ctrl Pts',(-8.38240796207935,-1.32768940188413,
-2.22355748240969));
#148861=CARTESIAN_POINT('Ctrl Pts',(-8.37708992878106,-1.33223595136664,
-2.22587306701158));
#148862=CARTESIAN_POINT('Ctrl Pts',(-8.37186287728827,-1.33650155467049,
-2.22893285255653));
#148863=CARTESIAN_POINT('Ctrl Pts',(-8.3578963904289,-1.34730670102584,
-2.23936278260429));
#148864=CARTESIAN_POINT('Ctrl Pts',(-8.34972493555017,-1.35293307624908,
-2.24811021831965));
#148865=CARTESIAN_POINT('Ctrl Pts',(-8.33889184152879,-1.35917045597279,
-2.26425741132905));
#148866=CARTESIAN_POINT('Ctrl Pts',(-8.33542528827331,-1.36087898842084,
-2.27049510689713));
#148867=CARTESIAN_POINT('Ctrl Pts',(-8.32945344089287,-1.36317274229213,
-2.28364647960213));
#148868=CARTESIAN_POINT('Ctrl Pts',(-8.32696672116125,-1.36375173586451,
-2.29051581947185));
#148869=CARTESIAN_POINT('Ctrl Pts',(-8.32502258313608,-1.36375173586619,
-2.29756024539374));
#148870=CARTESIAN_POINT('Ctrl Pts',(-8.32160303430179,-1.36375173586915,
-2.30995070231481));
#148871=CARTESIAN_POINT('Ctrl Pts',(-8.31991708957668,-1.36196031891332,
-2.32268170358541));
#148872=CARTESIAN_POINT('Ctrl Pts',(-8.32018379351912,-1.35499086522079,
-2.34752375480153));
#148873=CARTESIAN_POINT('Ctrl Pts',(-8.32216001209316,-1.3498599671427,
-2.3593769774175));
#148874=CARTESIAN_POINT('Ctrl Pts',(-8.32852282561185,-1.3387389448062,
-2.37764478615217));
#148875=CARTESIAN_POINT('Ctrl Pts',(-8.33205329208909,-1.33344492721209,
-2.3845514392093));
#148876=CARTESIAN_POINT('Ctrl Pts',(-8.33632902867257,-1.32768940204801,
-2.39052074728081));
#148877=CARTESIAN_POINT('Ctrl Pts',(-8.57696801758913,-1.00000000005396,
-2.72683325934723));
#148878=CARTESIAN_POINT('Ctrl Pts',(-8.4977586683085,-1.10901473814976,
-2.61617134608161));
#148879=CARTESIAN_POINT('Ctrl Pts',(-8.41756088626376,-1.21834403188794,
-2.50392763516742));
#148880=CARTESIAN_POINT('Ctrl Pts',(-8.33632902879467,-1.32768940197433,
-2.3905207471223));
#148881=CARTESIAN_POINT('',(-8.149344695,-1.32768940200002,-2.965999351));
#148882=CARTESIAN_POINT('Ctrl Pts',(-8.14934469528739,-1.32768940216563,
-2.96599935145307));
#148883=CARTESIAN_POINT('Ctrl Pts',(-8.281721783784,-1.21834383463976,-2.92199806015237));
#148884=CARTESIAN_POINT('Ctrl Pts',(-8.41257821073727,-1.10901465437208,
-2.87833011043717));
#148885=CARTESIAN_POINT('Ctrl Pts',(-8.54170526199449,-0.999999999874979,
-2.83536086230067));
#148886=CARTESIAN_POINT('',(-8.088484791,-1.32768940200002,-3.128159987));
#148887=CARTESIAN_POINT('Ctrl Pts',(-8.14934469528428,-1.32768940220673,
-2.96599935134145));
#148888=CARTESIAN_POINT('Ctrl Pts',(-8.14384050348253,-1.33223595163131,
-2.96782890925026));
#148889=CARTESIAN_POINT('Ctrl Pts',(-8.13836021756285,-1.33650155488223,
-2.97040782769713));
#148890=CARTESIAN_POINT('Ctrl Pts',(-8.12351502401358,-1.3473067011882,
-2.97954382365383));
#148891=CARTESIAN_POINT('Ctrl Pts',(-8.11459235092013,-1.35293307640658,
-2.98752356120022));
#148892=CARTESIAN_POINT('Ctrl Pts',(-8.10235544453277,-1.35917045612245,
-3.00263467930046));
#148893=CARTESIAN_POINT('Ctrl Pts',(-8.09834370388333,-1.36087898856765,
-3.00853652430322));
#148894=CARTESIAN_POINT('Ctrl Pts',(-8.09121701744787,-1.36317274243323,
-3.02109964117803));
#148895=CARTESIAN_POINT('Ctrl Pts',(-8.08812454564211,-1.36375173600275,
-3.02771841926748));
#148896=CARTESIAN_POINT('Ctrl Pts',(-8.08555677667574,-1.36375173600163,
-3.03456021521294));
#148897=CARTESIAN_POINT('Ctrl Pts',(-8.08104032194735,-1.36375173599966,
-3.04659426580439));
#148898=CARTESIAN_POINT('Ctrl Pts',(-8.07821996618797,-1.36196031903889,
-3.05912288888715));
#148899=CARTESIAN_POINT('Ctrl Pts',(-8.0762587721631,-1.35499086533698,
-3.08388884046511));
#148900=CARTESIAN_POINT('Ctrl Pts',(-8.07716452038241,-1.34985996725432,
-3.09587149235794));
#148901=CARTESIAN_POINT('Ctrl Pts',(-8.08186420533724,-1.3387389449198,
-3.11463611845344));
#148902=CARTESIAN_POINT('Ctrl Pts',(-8.08476135158299,-1.33344492733438,
-3.12183143591671));
#148903=CARTESIAN_POINT('Ctrl Pts',(-8.08848479065032,-1.32768940218083,
-3.12815998737017));
#148904=CARTESIAN_POINT('Ctrl Pts',(-8.29800821672471,-1.00000000020416,
-3.48468931635154));
#148905=CARTESIAN_POINT('Ctrl Pts',(-8.22903739841268,-1.10901473827415,
-3.3673726241933));
#148906=CARTESIAN_POINT('Ctrl Pts',(-8.15922391772688,-1.21834403198615,
-3.24839189981149));
#148907=CARTESIAN_POINT('Ctrl Pts',(-8.0884847908968,-1.32768940204711,
-3.12815998710355));
#148908=CARTESIAN_POINT('',(-7.850667698,-1.32768940200002,-3.684560736));
#148909=CARTESIAN_POINT('Ctrl Pts',(-7.85066769785711,-1.32768940157741,
-3.68456073683881));
#148910=CARTESIAN_POINT('Ctrl Pts',(-7.98645612010734,-1.21834383433082,
-3.65260277261617));
#148911=CARTESIAN_POINT('Ctrl Pts',(-8.12070012204856,-1.109014654343,-3.62084049699314));
#148912=CARTESIAN_POINT('Ctrl Pts',(-8.25315907913426,-1.00000000012425,
-3.58961909013581));
#148913=CARTESIAN_POINT('',(-7.77551683,-1.32768940200002,-3.840613121));
#148914=CARTESIAN_POINT('Ctrl Pts',(-7.85066769791922,-1.32768940194829,
-3.68456073583355));
#148915=CARTESIAN_POINT('Ctrl Pts',(-7.84502166401927,-1.3322359514189,
-3.68588953652913));
#148916=CARTESIAN_POINT('Ctrl Pts',(-7.83933226760092,-1.33650155471162,
-3.68796682397788));
#148917=CARTESIAN_POINT('Ctrl Pts',(-7.82372789202241,-1.34730670105384,
-3.69573532823492));
#148918=CARTESIAN_POINT('Ctrl Pts',(-7.81412584082863,-1.35293307627325,
-3.70288311945405));
#148919=CARTESIAN_POINT('Ctrl Pts',(-7.80058364644548,-1.35917045599074,
-3.71683649680358));
#148920=CARTESIAN_POINT('Ctrl Pts',(-7.79605901857717,-1.36087898843653,
-3.72235497305409));
#148921=CARTESIAN_POINT('Ctrl Pts',(-7.78783487297177,-1.36317274230328,
-3.73422868326696));
#148922=CARTESIAN_POINT('Ctrl Pts',(-7.78416154785462,-1.36375173587338,
-3.74054360906622));
#148923=CARTESIAN_POINT('Ctrl Pts',(-7.78099082211098,-1.36375173587283,
-3.74712768891714));
#148924=CARTESIAN_POINT('Ctrl Pts',(-7.7754138253233,-1.36375173587187,
-3.75870844207817));
#148925=CARTESIAN_POINT('Ctrl Pts',(-7.7714817663724,-1.36196031891213,
-3.77093381386658));
#148926=CARTESIAN_POINT('Ctrl Pts',(-7.76730846475425,-1.3549908652122,
-3.7954242649276));
#148927=CARTESIAN_POINT('Ctrl Pts',(-7.76713645006289,-1.3498599671305,
-3.80743986883124));
#148928=CARTESIAN_POINT('Ctrl Pts',(-7.77013516735406,-1.33873894479117,
-3.82655023058136));
#148929=CARTESIAN_POINT('Ctrl Pts',(-7.77237566726015,-1.33344492719833,
-3.83397628000856));
#148930=CARTESIAN_POINT('Ctrl Pts',(-7.77551682988422,-1.32768940203627,
-3.84061312108624));
#148931=CARTESIAN_POINT('Ctrl Pts',(-7.95223773319059,-1.00000000030882,
-4.2144887031835));
#148932=CARTESIAN_POINT('Ctrl Pts',(-7.8940607583389,-1.10901473835463,
-4.0914617970675));
#148933=CARTESIAN_POINT('Ctrl Pts',(-7.83519367612302,-1.21834403204217,
-3.96670202196032));
#148934=CARTESIAN_POINT('Ctrl Pts',(-7.77551682979917,-1.32768940207849,
-3.84061312116309));
#148935=CARTESIAN_POINT('',(-7.488781739,-1.32768940200002,-4.373456205));
#148936=CARTESIAN_POINT('Ctrl Pts',(-7.4887817391053,-1.3276894020377,-4.3734562055302));
#148937=CARTESIAN_POINT('Ctrl Pts',(-7.62688820723029,-1.21834383456909,
-4.3537988749128));
#148938=CARTESIAN_POINT('Ctrl Pts',(-7.76343893103024,-1.1090146543582,
-4.33419800434109));
#148939=CARTESIAN_POINT('Ctrl Pts',(-7.89816331292909,-0.999999999917443,
-4.3149758149713));
#148940=CARTESIAN_POINT('',(-7.399944978,-1.32768940200002,-4.522143898));
#148941=CARTESIAN_POINT('Ctrl Pts',(-7.48878173912938,-1.32768940209639,
-4.37345620537261));
#148942=CARTESIAN_POINT('Ctrl Pts',(-7.48303932181701,-1.33223595148123,
-4.37427355014363));
#148943=CARTESIAN_POINT('Ctrl Pts',(-7.47718662272123,-1.33650155469588,
-4.37583248146923));
#148944=CARTESIAN_POINT('Ctrl Pts',(-7.46094870251595,-1.34730670096865,
-4.38217094653701));
#148945=CARTESIAN_POINT('Ctrl Pts',(-7.45074458329346,-1.35293307618431,
-4.38842924161994));
#148946=CARTESIAN_POINT('Ctrl Pts',(-7.43600613470365,-1.35917045589565,
-4.40111253383243));
#148947=CARTESIAN_POINT('Ctrl Pts',(-7.43100504926067,-1.36087898833917,
-4.40620320980585));
#148948=CARTESIAN_POINT('Ctrl Pts',(-7.42174966047234,-1.3631727422014,
-4.41729191322548));
#148949=CARTESIAN_POINT('Ctrl Pts',(-7.41752505749903,-1.36375173576924,
-4.42325214266577));
#148950=CARTESIAN_POINT('Ctrl Pts',(-7.41377690379883,-1.36375173576648,
-4.42952549528285));
#148951=CARTESIAN_POINT('Ctrl Pts',(-7.40718426765269,-1.36375173576163,
-4.44055970959978));
#148952=CARTESIAN_POINT('Ctrl Pts',(-7.4021721641394,-1.36196031879803,
-4.45238339858914));
#148953=CARTESIAN_POINT('Ctrl Pts',(-7.39582035590394,-1.3549908650908,
-4.47640116642154));
#148954=CARTESIAN_POINT('Ctrl Pts',(-7.39457196326603,-1.34985996700553,
-4.48835297975807));
#148955=CARTESIAN_POINT('Ctrl Pts',(-7.39584556898713,-1.33873894466816,
-4.50765521174129));
#148956=CARTESIAN_POINT('Ctrl Pts',(-7.39741138335892,-1.3334449270826,
-4.51525220292776));
#148957=CARTESIAN_POINT('Ctrl Pts',(-7.39994497873345,-1.32768940192929,
-4.52214389767129));
#148958=CARTESIAN_POINT('Ctrl Pts',(-7.54244050677706,-1.00000000021305,
-4.91035550626367));
#148959=CARTESIAN_POINT('Ctrl Pts',(-7.49552578212922,-1.10901473827983,
-4.78260892651342));
#148960=CARTESIAN_POINT('Ctrl Pts',(-7.4480790614658,-1.21834403198914,
-4.65307459304682));
#148961=CARTESIAN_POINT('Ctrl Pts',(-7.39994497847541,-1.32768940204821,
-4.52214389786548));
#148962=CARTESIAN_POINT('',(-7.066600514,-1.32768940200002,-5.027139175));
#148963=CARTESIAN_POINT('Ctrl Pts',(-7.06660051407375,-1.32768940204712,
-5.02713917571187));
#148964=CARTESIAN_POINT('Ctrl Pts',(-7.20591307568901,-1.21834383453907,
-5.01994074814747));
#148965=CARTESIAN_POINT('Ctrl Pts',(-7.34367109490997,-1.10901465428964,
-5.01265909749143));
#148966=CARTESIAN_POINT('Ctrl Pts',(-7.47957617982504,-0.999999999810883,
-5.00559089155299));
#148967=CARTESIAN_POINT('',(-6.964793122,-1.32768940200002,-5.167265029));
#148968=CARTESIAN_POINT('Ctrl Pts',(-7.06660051416281,-1.32768940218437,
-5.0271391753499));
#148969=CARTESIAN_POINT('Ctrl Pts',(-7.06080794801292,-1.33223595147841,
-5.0274384834299));
#148970=CARTESIAN_POINT('Ctrl Pts',(-7.05483906874339,-1.33650155461116,
-5.02846650704578));
#148971=CARTESIAN_POINT('Ctrl Pts',(-7.0380983421117,-1.34730670081974,
-5.0333238993322));
#148972=CARTESIAN_POINT('Ctrl Pts',(-7.02737431242565,-1.35293307604024,
-5.03864231015989));
#148973=CARTESIAN_POINT('Ctrl Pts',(-7.01155827494507,-1.35917045575939,
-5.04995339881579));
#148974=CARTESIAN_POINT('Ctrl Pts',(-7.00612099772445,-1.36087898820574,
-5.05457528737984));
#148975=CARTESIAN_POINT('Ctrl Pts',(-6.99590888469632,-1.36317274207366,
-5.06478970428212));
#148976=CARTESIAN_POINT('Ctrl Pts',(-6.99116701788302,-1.36375173564436,
-5.07034724909892));
#148977=CARTESIAN_POINT('Ctrl Pts',(-6.9868716141528,-1.36375173564439,
-5.07625936513457));
#148978=CARTESIAN_POINT('Ctrl Pts',(-6.9793164186734,-1.36375173564445,
-5.08665819959847));
#148979=CARTESIAN_POINT('Ctrl Pts',(-6.97326462510242,-1.36196031868577,
-5.09798500839567));
#148980=CARTESIAN_POINT('Ctrl Pts',(-6.96478545126267,-1.35499086498787,
-5.121336716054));
#148981=CARTESIAN_POINT('Ctrl Pts',(-6.96247073199496,-1.34985996690716,
-5.13312850985035));
#148982=CARTESIAN_POINT('Ctrl Pts',(-6.96200897181234,-1.33873894460026,
-5.15246720181947));
#148983=CARTESIAN_POINT('Ctrl Pts',(-6.9628874936231,-1.3334449270472,-5.16017396823524));
#148984=CARTESIAN_POINT('Ctrl Pts',(-6.96479312271032,-1.32768940192986,
-5.16726502875217));
#148985=CARTESIAN_POINT('Ctrl Pts',(-7.07191598493006,-1.0000000000433,
-5.56668701305467));
#148986=CARTESIAN_POINT('Ctrl Pts',(-7.03664124030446,-1.1090147382238,
-5.43524929978372));
#148987=CARTESIAN_POINT('Ctrl Pts',(-7.00099689432893,-1.21834403204728,
-5.30198334200608));
#148988=CARTESIAN_POINT('Ctrl Pts',(-6.96479312204206,-1.32768940221948,
-5.16726502916683));
#148989=CARTESIAN_POINT('',(-6.587523177,-1.32768940200002,-5.640346578));
#148990=CARTESIAN_POINT('Ctrl Pts',(-6.58752317677662,-1.32768940171009,
-5.64034657789402));
#148991=CARTESIAN_POINT('Ctrl Pts',(-6.72692016891382,-1.2183438343021,
-5.64566501082948));
#148992=CARTESIAN_POINT('Ctrl Pts',(-6.86477633685045,-1.10901465415312,
-5.6507612075996));
#148993=CARTESIAN_POINT('Ctrl Pts',(-7.00076789681646,-0.999999999774391,
-5.65590389407081));
#148994=CARTESIAN_POINT('',(-6.473564847,-1.32768940200002,-5.770782381));
#148995=CARTESIAN_POINT('Ctrl Pts',(-6.58752317690415,-1.32768940185457,
-5.64034657752293));
#148996=CARTESIAN_POINT('Ctrl Pts',(-6.58172709993427,-1.33223595135912,
-5.64012543898217));
#148997=CARTESIAN_POINT('Ctrl Pts',(-6.57569009804838,-1.33650155468271,
-5.64061427785487));
#148998=CARTESIAN_POINT('Ctrl Pts',(-6.55858135111833,-1.34730670105206,
-5.64395148859084));
#148999=CARTESIAN_POINT('Ctrl Pts',(-6.54742375455179,-1.35293307627263,
-5.64828719444978));
#149000=CARTESIAN_POINT('Ctrl Pts',(-6.53065746961771,-1.359170455992,-5.65813500931786));
#149001=CARTESIAN_POINT('Ctrl Pts',(-6.52482777837963,-1.36087898843846,
-5.66225089774472));
#149002=CARTESIAN_POINT('Ctrl Pts',(-6.51374116304362,-1.36317274230659,
-5.67150878765279));
#149003=CARTESIAN_POINT('Ctrl Pts',(-6.50852021111509,-1.36375173587738,
-5.67661890176379));
#149004=CARTESIAN_POINT('Ctrl Pts',(-6.50371214142148,-1.36375173587751,
-5.6821221803364));
#149005=CARTESIAN_POINT('Ctrl Pts',(-6.49525521660246,-1.36375173587773,
-5.69180190964827));
#149006=CARTESIAN_POINT('Ctrl Pts',(-6.48821245845978,-1.36196031891918,
-5.70254064144979));
#149007=CARTESIAN_POINT('Ctrl Pts',(-6.47767418834347,-1.35499086522148,
-5.72503827471508));
#149008=CARTESIAN_POINT('Ctrl Pts',(-6.47431177920769,-1.34985996714086,
-5.73657510838083));
#149009=CARTESIAN_POINT('Ctrl Pts',(-6.47211837095175,-1.33873894483526,
-5.7557945565959));
#149010=CARTESIAN_POINT('Ctrl Pts',(-6.47230252687583,-1.33344492728374,
-5.76354904792197));
#149011=CARTESIAN_POINT('Ctrl Pts',(-6.47356484669523,-1.32768940216811,
-5.77078238118694));
#149012=CARTESIAN_POINT('Ctrl Pts',(-6.54445255389812,-0.999999999960802,
-6.17819882898586));
#149013=CARTESIAN_POINT('Ctrl Pts',(-6.52110180080846,-1.10901473814172,
-6.04412824156698));
#149014=CARTESIAN_POINT('Ctrl Pts',(-6.49754681684949,-1.21834403196543,
-5.90820363880618));
#149015=CARTESIAN_POINT('Ctrl Pts',(-6.47356484676908,-1.32768940213768,
-5.77078238114983));
#149016=CARTESIAN_POINT('',(-6.055406976,-1.32768940200002,-6.208141225));
#149017=CARTESIAN_POINT('Ctrl Pts',(-6.05540697605073,-1.32768940208598,
-6.20814122513386));
#149018=CARTESIAN_POINT('Ctrl Pts',(-6.19376605621082,-1.21834383468118,
-6.22593369766438));
#149019=CARTESIAN_POINT('Ctrl Pts',(-6.33061043617275,-1.10901465453519,
-6.24336671027083));
#149020=CARTESIAN_POINT('Ctrl Pts',(-6.46559354722401,-1.00000000015905,
-6.26067888325481));
#149021=CARTESIAN_POINT('',(-5.930215234,-1.32768940200002,-6.327836787));
#149022=CARTESIAN_POINT('Ctrl Pts',(-6.05540697612598,-1.3276894021538,
-6.20814122496572));
#149023=CARTESIAN_POINT('Ctrl Pts',(-6.04965405520632,-1.33223595161668,
-6.20740142034681));
#149024=CARTESIAN_POINT('Ctrl Pts',(-6.04359753738464,-1.33650155490257,
-6.20734713862694));
#149025=CARTESIAN_POINT('Ctrl Pts',(-6.02625852002746,-1.34730670124085,
-6.20913729847659));
#149026=CARTESIAN_POINT('Ctrl Pts',(-6.01475719098768,-1.35293307646214,
-6.21245539081279));
#149027=CARTESIAN_POINT('Ctrl Pts',(-5.99717565086843,-1.35917045618278,
-6.22076064307862));
#149028=CARTESIAN_POINT('Ctrl Pts',(-5.99100048285914,-1.36087898862972,
-6.22433739265494));
#149029=CARTESIAN_POINT('Ctrl Pts',(-5.97912862812349,-1.3631727424988,
-6.23256421648309));
#149030=CARTESIAN_POINT('Ctrl Pts',(-5.97347062711499,-1.36375173607006,
-6.23718575625433));
#149031=CARTESIAN_POINT('Ctrl Pts',(-5.96818860320827,-1.36375173607065,
-6.24223588820087));
#149032=CARTESIAN_POINT('Ctrl Pts',(-5.95889803923611,-1.36375173607169,
-6.25111857687207));
#149033=CARTESIAN_POINT('Ctrl Pts',(-5.95092102066962,-1.36196031911391,
-6.2611827697239));
#149034=CARTESIAN_POINT('Ctrl Pts',(-5.93840850223206,-1.35499086541765,
-6.28264519088179));
#149035=CARTESIAN_POINT('Ctrl Pts',(-5.93402547536983,-1.34985996733774,
-6.29383417661586));
#149036=CARTESIAN_POINT('Ctrl Pts',(-5.93011807903562,-1.33873894492255,
-6.31277963757132));
#149037=CARTESIAN_POINT('Ctrl Pts',(-5.92960638637303,-1.33344492723105,
-6.32051941938347));
#149038=CARTESIAN_POINT('Ctrl Pts',(-5.93021523353628,-1.32768940195741,
-6.32783678700507));
#149039=CARTESIAN_POINT('Ctrl Pts',(-5.96429703904196,-0.999999999791271,
-6.73996742082874));
#149040=CARTESIAN_POINT('Ctrl Pts',(-5.95305828402978,-1.10901473792973,
-6.60434341685274));
#149041=CARTESIAN_POINT('Ctrl Pts',(-5.94178231297559,-1.21834403171087,
-6.46685455414235));
#149042=CARTESIAN_POINT('Ctrl Pts',(-5.93021523383119,-1.32768940184066,
-6.3278367868887));
#149043=CARTESIAN_POINT('',(-5.474536198,-1.32768940200002,-6.725951571));
#149044=CARTESIAN_POINT('Ctrl Pts',(-5.47453619793898,-1.32768940194877,
-6.72595157108985));
#149045=CARTESIAN_POINT('Ctrl Pts',(-5.61074338033991,-1.21834383447162,
-6.75607482866063));
#149046=CARTESIAN_POINT('Ctrl Pts',(-5.74547418201546,-1.10901465425249,
-6.78570429670652));
#149047=CARTESIAN_POINT('Ctrl Pts',(-5.87836203967683,-0.999999999803766,
-6.81504656873443));
#149048=CARTESIAN_POINT('',(-5.339119014,-1.32768940200002,-6.833943172));
#149049=CARTESIAN_POINT('Ctrl Pts',(-5.47453619794346,-1.3276894019521,
-6.72595157108191));
#149050=CARTESIAN_POINT('Ctrl Pts',(-5.46887275217696,-1.33223595140147,
-6.72469905685192));
#149051=CARTESIAN_POINT('Ctrl Pts',(-5.46284548190358,-1.33650155467468,
-6.72410209158784));
#149052=CARTESIAN_POINT('Ctrl Pts',(-5.44541579765377,-1.34730670099757,
-6.72433078725383));
#149053=CARTESIAN_POINT('Ctrl Pts',(-5.43366333807953,-1.35293307621405,
-6.72660455074311));
#149054=CARTESIAN_POINT('Ctrl Pts',(-5.41540809900002,-1.35917045592673,
-6.73330037140443));
#149055=CARTESIAN_POINT('Ctrl Pts',(-5.40893717304231,-1.36087898837075,
-6.73630918424744));
#149056=CARTESIAN_POINT('Ctrl Pts',(-5.39637566410319,-1.36317274223397,
-6.74343870445049));
#149057=CARTESIAN_POINT('Ctrl Pts',(-5.39032616891343,-1.36375173580231,
-6.74753445996235));
#149058=CARTESIAN_POINT('Ctrl Pts',(-5.38461271854601,-1.36375173580003,
-6.75209078459071));
#149059=CARTESIAN_POINT('Ctrl Pts',(-5.37456331758125,-1.36375173579604,
-6.76010491443722));
#149060=CARTESIAN_POINT('Ctrl Pts',(-5.36571626485716,-1.36196031883327,
-6.76941353737757));
#149061=CARTESIAN_POINT('Ctrl Pts',(-5.35133024154627,-1.35499086512763,
-6.78966794363456));
#149062=CARTESIAN_POINT('Ctrl Pts',(-5.34596188651656,-1.34985996704314,
-6.80041899430357));
#149063=CARTESIAN_POINT('Ctrl Pts',(-5.340371962258,-1.33873894475413,-6.81893792987469));
#149064=CARTESIAN_POINT('Ctrl Pts',(-5.33916854083174,-1.33344492722887,
-6.82660068560841));
#149065=CARTESIAN_POINT('Ctrl Pts',(-5.33911901311749,-1.32768940214345,
-6.83394317210648));
#149066=CARTESIAN_POINT('Ctrl Pts',(-5.33612051055408,-1.00000000012717,
-7.2474697580987));
#149067=CARTESIAN_POINT('Ctrl Pts',(-5.33708424139336,-1.10901473818033,
-7.11138430241067));
#149068=CARTESIAN_POINT('Ctrl Pts',(-5.33817807065952,-1.21834403187569,
-6.97343815934645));
#149069=CARTESIAN_POINT('Ctrl Pts',(-5.33911901369835,-1.32768940192049,
-6.83394317193562));
#149070=CARTESIAN_POINT('',(-4.84958767583258,-1.32768940194837,-7.18960850739357));
#149071=CARTESIAN_POINT('Ctrl Pts',(-4.84958767551919,-1.32768940181776,
-7.18960850804234));
#149072=CARTESIAN_POINT('Ctrl Pts',(-4.9825462995355,-1.21834383449911,
-7.2318200159394));
#149073=CARTESIAN_POINT('Ctrl Pts',(-5.11407874926016,-1.10901465444024,
-7.27340738041884));
#149074=CARTESIAN_POINT('Ctrl Pts',(-5.24380141818337,-1.00000000015115,
-7.31454350482226));
#149075=CARTESIAN_POINT('',(-4.705035349,-1.32768940200002,-7.285026664));
#149076=CARTESIAN_POINT('Ctrl Pts',(-4.84958767607711,-1.32768940218148,
-7.18960850722729));
#149077=CARTESIAN_POINT('Ctrl Pts',(-4.84405930425442,-1.33223595156484,
-7.18785336792303));
#149078=CARTESIAN_POINT('Ctrl Pts',(-4.83810980963134,-1.33650155477901,
-7.18671852554355));
#149079=CARTESIAN_POINT('Ctrl Pts',(-4.82072979213365,-1.34730670106102,
-7.1853839156919));
#149080=CARTESIAN_POINT('Ctrl Pts',(-4.80882082591909,-1.35293307628648,
-7.18659504331653));
#149081=CARTESIAN_POINT('Ctrl Pts',(-4.79003886832667,-1.35917045601382,
-7.19162752154787));
#149082=CARTESIAN_POINT('Ctrl Pts',(-4.78332428450955,-1.36087898846318,
-7.19404417246096));
#149083=CARTESIAN_POINT('Ctrl Pts',(-4.77017425924561,-1.36317274233714,
-7.20001898632597));
#149084=CARTESIAN_POINT('Ctrl Pts',(-4.76378197684949,-1.36375173591085,
-7.20355598095978));
#149085=CARTESIAN_POINT('Ctrl Pts',(-4.75768310136027,-1.36375173591383,
-7.20758181342033));
#149086=CARTESIAN_POINT('Ctrl Pts',(-4.74695577526566,-1.36375173591907,
-7.2146628593743));
#149087=CARTESIAN_POINT('Ctrl Pts',(-4.73730991964321,-1.36196031896553,
-7.22314096483993));
#149088=CARTESIAN_POINT('Ctrl Pts',(-4.72116621924342,-1.35499086527729,
-7.24202427961917));
#149089=CARTESIAN_POINT('Ctrl Pts',(-4.71485575887476,-1.3498599672013,
-7.25225083408193));
#149090=CARTESIAN_POINT('Ctrl Pts',(-4.70762831330155,-1.33873894475924,
-7.2701941411816));
#149091=CARTESIAN_POINT('Ctrl Pts',(-4.70574285233601,-1.33344492702836,
-7.27771817531576));
#149092=CARTESIAN_POINT('Ctrl Pts',(-4.70503534864306,-1.32768940170969,
-7.28502666373681));
#149093=CARTESIAN_POINT('Ctrl Pts',(-4.66498067879555,-0.999999999952127,
-7.69661972994159));
#149094=CARTESIAN_POINT('Ctrl Pts',(-4.67813913625211,-1.10901473800108,
-7.56116850237982));
#149095=CARTESIAN_POINT('Ctrl Pts',(-4.6915939591275,-1.21834403169194,
-7.42387573995099));
#149096=CARTESIAN_POINT('Ctrl Pts',(-4.70503534858687,-1.32768940173078,
-7.28502666374798));
#149097=CARTESIAN_POINT('',(-4.185593123,-1.32768940200002,-7.595378945));
#149098=CARTESIAN_POINT('Ctrl Pts',(-4.18559312299155,-1.32768940217896,
-7.59537894538274));
#149099=CARTESIAN_POINT('Ctrl Pts',(-4.31423268431485,-1.21834383483831,
-7.64933884133742));
#149100=CARTESIAN_POINT('Ctrl Pts',(-4.44150776048922,-1.10901465475701,
-7.70254926521416));
#149101=CARTESIAN_POINT('Ctrl Pts',(-4.56702079035568,-1.00000000044527,
-7.75514803807409));
#149102=CARTESIAN_POINT('',(-4.033069504,-1.32768940200002,-7.677455405));
#149103=CARTESIAN_POINT('Ctrl Pts',(-4.18559312312532,-1.32768940225632,
-7.5953789452207));
#149104=CARTESIAN_POINT('Ctrl Pts',(-4.18024433645438,-1.33223595154869,
-7.5931353122223));
#149105=CARTESIAN_POINT('Ctrl Pts',(-4.17442051933056,-1.33650155468029,
-7.59147172983892));
#149106=CARTESIAN_POINT('Ctrl Pts',(-4.1572301022881,-1.3473067008919,-7.58858455999571));
#149107=CARTESIAN_POINT('Ctrl Pts',(-4.14526051342689,-1.35293307611646,
-7.58872330047545));
#149108=CARTESIAN_POINT('Ctrl Pts',(-4.12610305860312,-1.35917045584226,
-7.59205191773052));
#149109=CARTESIAN_POINT('Ctrl Pts',(-4.11919887880873,-1.36087898829105,
-7.59385694926454));
#149110=CARTESIAN_POINT('Ctrl Pts',(-4.10556621349489,-1.36317274216386,
-7.59862895110864));
#149111=CARTESIAN_POINT('Ctrl Pts',(-4.09888261079392,-1.36375173573699,
-7.60157870706549));
#149112=CARTESIAN_POINT('Ctrl Pts',(-4.09244741474498,-1.36375173573942,
-7.60504163372406));
#149113=CARTESIAN_POINT('Ctrl Pts',(-4.0811285336459,-1.36375173574368,
-7.61113258337114));
#149114=CARTESIAN_POINT('Ctrl Pts',(-4.07076153788779,-1.36196031878918,
-7.61871191064466));
#149115=CARTESIAN_POINT('Ctrl Pts',(-4.0529901399933,-1.35499086509917,
-7.63607209660278));
#149116=CARTESIAN_POINT('Ctrl Pts',(-4.04578838240849,-1.34985996702232,
-7.64569181665736));
#149117=CARTESIAN_POINT('Ctrl Pts',(-4.03698160687458,-1.33873894472513,
-7.66291502582497));
#149118=CARTESIAN_POINT('Ctrl Pts',(-4.03442928704494,-1.33344492717922,
-7.67023975875926));
#149119=CARTESIAN_POINT('Ctrl Pts',(-4.03306950367077,-1.32768940206933,
-7.67745540499324));
#149120=CARTESIAN_POINT('Ctrl Pts',(-3.95628116425374,-0.99999999991297,
-8.08380104597694));
#149121=CARTESIAN_POINT('Ctrl Pts',(-3.98152840407528,-1.10901473807425,
-7.95007462013823));
#149122=CARTESIAN_POINT('Ctrl Pts',(-4.00723589014992,-1.21834403187787,
-7.81454063889854));
#149123=CARTESIAN_POINT('Ctrl Pts',(-4.03306950377905,-1.32768940202923,
-7.67745540498166));
#149124=CARTESIAN_POINT('',(-3.48789863553934,-1.3276894017749,-7.93999585849295));
#149125=CARTESIAN_POINT('Ctrl Pts',(-3.48789863503968,-1.32768940145685,
-7.93999585890387));
#149126=CARTESIAN_POINT('Ctrl Pts',(-3.61118340371515,-1.21834383408035,
-8.00526968952849));
#149127=CARTESIAN_POINT('Ctrl Pts',(-3.7331763624119,-1.10901465396194,
-8.06967475372052));
#149128=CARTESIAN_POINT('Ctrl Pts',(-3.85346919624949,-0.999999999613144,
-8.13331268060684));
#149129=CARTESIAN_POINT('',(-3.328631754,-1.32768940200002,-8.00806979));
#149130=CARTESIAN_POINT('Ctrl Pts',(-3.48789863549781,-1.32768940169677,
-7.93999585844058));
#149131=CARTESIAN_POINT('Ctrl Pts',(-3.48277249902713,-1.3322359511742,
-7.93728179597329));
#149132=CARTESIAN_POINT('Ctrl Pts',(-3.47712124905877,-1.3365015544728,
-7.93510286764403));
#149133=CARTESIAN_POINT('Ctrl Pts',(-3.46025883926027,-1.34730670081656,
-7.93068638354844));
#149134=CARTESIAN_POINT('Ctrl Pts',(-3.44832499984238,-1.35293307603251,
-7.92975161983458));
#149135=CARTESIAN_POINT('Ctrl Pts',(-3.42894629234947,-1.35917045574423,
-7.93134957605619));
#149136=CARTESIAN_POINT('Ctrl Pts',(-3.42190810497447,-1.36087898818788,
-7.93252845516265));
#149137=CARTESIAN_POINT('Ctrl Pts',(-3.40790256181816,-1.36317274205036,
-7.93605922364059));
#149138=CARTESIAN_POINT('Ctrl Pts',(-3.40098145125301,-1.36375173561834,
-7.93839799122359));
#149139=CARTESIAN_POINT('Ctrl Pts',(-3.39426174706129,-1.36375173561571,
-7.94127013063417));
#149140=CARTESIAN_POINT('Ctrl Pts',(-3.38244244393535,-1.36375173561109,
-7.94632194323558));
#149141=CARTESIAN_POINT('Ctrl Pts',(-3.37143777699998,-1.36196031864774,
-7.95294146803597));
#149142=CARTESIAN_POINT('Ctrl Pts',(-3.35218176646764,-1.35499086494101,
-7.96863875117293));
#149143=CARTESIAN_POINT('Ctrl Pts',(-3.34414669599052,-1.34985996685599,
-7.97757418449405));
#149144=CARTESIAN_POINT('Ctrl Pts',(-3.33383149747034,-1.33873894463069,
-7.9939386246935));
#149145=CARTESIAN_POINT('Ctrl Pts',(-3.33063286857535,-1.33344492718698,
-8.00100508209111));
#149146=CARTESIAN_POINT('Ctrl Pts',(-3.32863175374708,-1.32768940219364,
-8.0080697900861));
#149147=CARTESIAN_POINT('Ctrl Pts',(-3.21572799953932,-1.00000000015765,
-8.40589634900059));
#149148=CARTESIAN_POINT('Ctrl Pts',(-3.25286074564109,-1.10901473828873,
-8.27497141166348));
#149149=CARTESIAN_POINT('Ctrl Pts',(-3.29061391319593,-1.21834403206224,
-8.14228745177371));
#149150=CARTESIAN_POINT('Ctrl Pts',(-3.32863175377033,-1.32768940218507,
-8.00806979008571));
#149151=CARTESIAN_POINT('',(-2.76212164,-1.32768940200002,-8.220684592));
#149152=CARTESIAN_POINT('Ctrl Pts',(-2.76212164018735,-1.3276894021635,
-8.22068459194698));
#149153=CARTESIAN_POINT('Ctrl Pts',(-2.87905899951265,-1.21834383472095,
-8.29674681085365));
#149154=CARTESIAN_POINT('Ctrl Pts',(-2.99478762493088,-1.10901465453746,
-8.37182796377343));
#149155=CARTESIAN_POINT('Ctrl Pts',(-3.10889173535242,-1.00000000012429,
-8.44599266964046));
#149156=CARTESIAN_POINT('',(-2.59739382,-1.32768940200002,-8.274207905));
#149157=CARTESIAN_POINT('Ctrl Pts',(-2.76212164024878,-1.32768940219308,
-8.22068459189514));
#149158=CARTESIAN_POINT('Ctrl Pts',(-2.7572594268428,-1.33223595159149,
-8.21752195217761));
#149159=CARTESIAN_POINT('Ctrl Pts',(-2.75182624485655,-1.33650155481903,
-8.21484522147966));
#149160=CARTESIAN_POINT('Ctrl Pts',(-2.73542760884484,-1.34730670110943,
-8.20893498211433));
#149161=CARTESIAN_POINT('Ctrl Pts',(-2.72362560313124,-1.35293307633198,
-8.20693424036015));
#149162=CARTESIAN_POINT('Ctrl Pts',(-2.7041816689267,-1.3591704560546,-8.20678866972344));
#149163=CARTESIAN_POINT('Ctrl Pts',(-2.69706614131622,-1.36087898850225,
-8.20733190475376));
#149164=CARTESIAN_POINT('Ctrl Pts',(-2.68280048471138,-1.36317274237276,
-8.20959301218038));
#149165=CARTESIAN_POINT('Ctrl Pts',(-2.67569759099158,-1.36375173594474,
-8.21130196100191));
#149166=CARTESIAN_POINT('Ctrl Pts',(-2.66874748175985,-1.36375173594603,
-8.21356018838122));
#149167=CARTESIAN_POINT('Ctrl Pts',(-2.65652291868143,-1.36375173594831,
-8.21753218970138));
#149168=CARTESIAN_POINT('Ctrl Pts',(-2.64496918366811,-1.36196031899179,
-8.2231386154978));
#149169=CARTESIAN_POINT('Ctrl Pts',(-2.62438359855294,-1.35499086529792,
-8.23704661050358));
#149170=CARTESIAN_POINT('Ctrl Pts',(-2.61557990883475,-1.34985996721919,
-8.24522581422892));
#149171=CARTESIAN_POINT('Ctrl Pts',(-2.60383933905131,-1.33873894490893,
-8.26059972886249));
#149172=CARTESIAN_POINT('Ctrl Pts',(-2.60002015447877,-1.33344492734899,
-8.26735101603765));
#149173=CARTESIAN_POINT('Ctrl Pts',(-2.59739381999828,-1.32768940222356,
-8.27420790518698));
#149174=CARTESIAN_POINT('Ctrl Pts',(-2.44928368525819,-0.999999999982717,
-8.66031231708415));
#149175=CARTESIAN_POINT('Ctrl Pts',(-2.49800296686794,-1.10901473814177,
-8.53324299868092));
#149176=CARTESIAN_POINT('Ctrl Pts',(-2.54749784986341,-1.21834403194323,
-8.40447735317844));
#149177=CARTESIAN_POINT('Ctrl Pts',(-2.59739382035255,-1.32768940209275,
-8.27420790521288));
#149178=CARTESIAN_POINT('',(-2.01410566465369,-1.3276894019719,-8.43518520740466));
#149179=CARTESIAN_POINT('Ctrl Pts',(-2.01410566413619,-1.32768940192452,
-8.43518520800257));
#149180=CARTESIAN_POINT('Ctrl Pts',(-2.12375410335395,-1.21834383447808,
-8.52142340685227));
#149181=CARTESIAN_POINT('Ctrl Pts',(-2.23228661674758,-1.10901465429013,
-8.606576139125));
#149182=CARTESIAN_POINT('Ctrl Pts',(-2.33928330464295,-0.999999999872264,
-8.69067049328867));
#149183=CARTESIAN_POINT('',(-1.845243197,-1.32768940200002,-8.473726964));
#149184=CARTESIAN_POINT('Ctrl Pts',(-2.01410566493824,-1.32768940228522,
-8.43518520744022));
#149185=CARTESIAN_POINT('Ctrl Pts',(-2.00954652218688,-1.33223595171976,
-8.43159945409989));
#149186=CARTESIAN_POINT('Ctrl Pts',(-2.00437515284886,-1.33650155497982,
-8.42844647242926));
#149187=CARTESIAN_POINT('Ctrl Pts',(-1.98857232265248,-1.34730670129488,
-8.42109006353586));
#149188=CARTESIAN_POINT('Ctrl Pts',(-1.97699717345128,-1.35293307651467,
-8.41803945254678));
#149189=CARTESIAN_POINT('Ctrl Pts',(-1.9576445636601,-1.3591704562329,-8.41615152711445));
#149190=CARTESIAN_POINT('Ctrl Pts',(-1.95050898585903,-1.36087898867897,
-8.41605474426427));
#149191=CARTESIAN_POINT('Ctrl Pts',(-1.9360980744867,-1.3631727425463,-8.41702798554097));
#149192=CARTESIAN_POINT('Ctrl Pts',(-1.92887058593776,-1.36375173611669,
-8.41809335615413));
#149193=CARTESIAN_POINT('Ctrl Pts',(-1.92174602986137,-1.36375173611641,
-8.41971948958691));
#149194=CARTESIAN_POINT('Ctrl Pts',(-1.90921463182691,-1.36375173611594,
-8.422579699414));
#149195=CARTESIAN_POINT('Ctrl Pts',(-1.89720485262118,-1.36196031915664,
-8.42712788656892));
#149196=CARTESIAN_POINT('Ctrl Pts',(-1.87545543596194,-1.3549908654575,
-8.43913461445685));
#149197=CARTESIAN_POINT('Ctrl Pts',(-1.8659540091429,-1.34985996737619,
-8.44649173445249));
#149198=CARTESIAN_POINT('Ctrl Pts',(-1.85288259622497,-1.3387389449445,
-8.46075134181751));
#149199=CARTESIAN_POINT('Ctrl Pts',(-1.8484736057682,-1.33344492723397,
-8.46713310140139));
#149200=CARTESIAN_POINT('Ctrl Pts',(-1.84524319731389,-1.32768940193907,
-8.47372696410058));
#149201=CARTESIAN_POINT('Ctrl Pts',(-1.66311917770952,-0.999999999928504,
-8.84500054279377));
#149202=CARTESIAN_POINT('Ctrl Pts',(-1.7230327356253,-1.10901473804792,
-8.72280993090161));
#149203=CARTESIAN_POINT('Ctrl Pts',(-1.78387083017168,-1.21834403180964,
-8.59899934519942));
#149204=CARTESIAN_POINT('Ctrl Pts',(-1.84524319736451,-1.32768940192018,
-8.47372696410889));
#149205=CARTESIAN_POINT('',(-1.249873295,-1.32768940200002,-8.581770672));
#149206=CARTESIAN_POINT('Ctrl Pts',(-1.24987329474725,-1.32768940183712,
-8.58177067208186));
#149207=CARTESIAN_POINT('Ctrl Pts',(-1.35134998891948,-1.21834383452832,
-8.67749051148482));
#149208=CARTESIAN_POINT('Ctrl Pts',(-1.45181255013311,-1.10901465447807,
-8.7720292232633));
#149209=CARTESIAN_POINT('Ctrl Pts',(-1.55084034091679,-1.00000000019697,
-8.86537614731828));
#149210=CARTESIAN_POINT('',(-1.078235761,-1.32768940200002,-8.605020555));
#149211=CARTESIAN_POINT('Ctrl Pts',(-1.24987329478272,-1.32768940185216,
-8.5817706720615));
#149212=CARTESIAN_POINT('Ctrl Pts',(-1.24565393021003,-1.33223595135743,
-8.57779067543879));
#149213=CARTESIAN_POINT('Ctrl Pts',(-1.24078601032253,-1.33650155468153,
-8.5741868287156));
#149214=CARTESIAN_POINT('Ctrl Pts',(-1.22570622100734,-1.34730670104963,
-8.56544347974055));
#149215=CARTESIAN_POINT('Ctrl Pts',(-1.21445112461428,-1.3529330762685,
-8.56136756123979));
#149216=CARTESIAN_POINT('Ctrl Pts',(-1.1953456550714,-1.3591704559851,-8.55775248147335));
#149217=CARTESIAN_POINT('Ctrl Pts',(-1.18824747855661,-1.36087898843055,
-8.55701645997984));
#149218=CARTESIAN_POINT('Ctrl Pts',(-1.17380734060151,-1.36317274229665,
-8.55669399913736));
#149219=CARTESIAN_POINT('Ctrl Pts',(-1.1665134487113,-1.36375173586643,
-8.55710721380306));
#149220=CARTESIAN_POINT('Ctrl Pts',(-1.1592718085262,-1.36375173586556,
-8.55808816061781));
#149221=CARTESIAN_POINT('Ctrl Pts',(-1.14653447098409,-1.36375173586404,
-8.55981355022169));
#149222=CARTESIAN_POINT('Ctrl Pts',(-1.1341653432657,-1.36196031890374,
-8.5632668794042));
#149223=CARTESIAN_POINT('Ctrl Pts',(-1.11142720857434,-1.35499086520275,
-8.5732756690572));
#149224=CARTESIAN_POINT('Ctrl Pts',(-1.10130454455473,-1.34985996712054,
-8.57975147011711));
#149225=CARTESIAN_POINT('Ctrl Pts',(-1.08700753210465,-1.33873894480506,
-8.59278195993714));
#149226=CARTESIAN_POINT('Ctrl Pts',(-1.0820442345278,-1.33344492724318,
-8.59874280941312));
#149227=CARTESIAN_POINT('Ctrl Pts',(-1.07823576149093,-1.32768940211611,
-8.60502055540426));
#149228=CARTESIAN_POINT('Ctrl Pts',(-0.863564212198985,-0.999999999788605,
-8.95847402492269));
#149229=CARTESIAN_POINT('Ctrl Pts',(-0.934189657823289,-1.10901473803966,
-8.84214592630361));
#149230=CARTESIAN_POINT('Ctrl Pts',(-1.00588113150084,-1.2183440319341,
-8.72428725023411));
#149231=CARTESIAN_POINT('Ctrl Pts',(-1.07823576132974,-1.32768940217741,
-8.60502055536268));
#149232=CARTESIAN_POINT('',(-0.475577681,-1.32768940200002,-8.659260764));
#149233=CARTESIAN_POINT('Ctrl Pts',(-0.475577680456156,-1.32768940202431,
-8.65926076450709));
#149234=CARTESIAN_POINT('Ctrl Pts',(-0.568065599076002,-1.21834383457737,
-8.76369156484591));
#149235=CARTESIAN_POINT('Ctrl Pts',(-0.659649342801167,-1.10901465438963,
-8.8668550862539));
#149236=CARTESIAN_POINT('Ctrl Pts',(-0.749910923085495,-0.999999999972134,
-8.96870300589438));
#149237=CARTESIAN_POINT('',(-0.302547006,-1.32768940200002,-8.667031581));
#149238=CARTESIAN_POINT('Ctrl Pts',(-0.475577681121855,-1.32768940229424,
-8.6592607642002));
#149239=CARTESIAN_POINT('Ctrl Pts',(-0.471732066689365,-1.33223595165812,
-8.65491856908753));
#149240=CARTESIAN_POINT('Ctrl Pts',(-0.467206790057779,-1.33650155485448,
-8.65089287353958));
#149241=CARTESIAN_POINT('Ctrl Pts',(-0.452971455449954,-1.34730670111979,
-8.64083298092142));
#149242=CARTESIAN_POINT('Ctrl Pts',(-0.442127031285838,-1.35293307634352,
-8.63576457180455));
#149243=CARTESIAN_POINT('Ctrl Pts',(-0.423422528000185,-1.35917045606808,
-8.6304514441951));
#149244=CARTESIAN_POINT('Ctrl Pts',(-0.416418903115635,-1.36087898851643,
-8.62908211006861));
#149245=CARTESIAN_POINT('Ctrl Pts',(-0.402065802077877,-1.36317274238836,
-8.62746654336825));
#149246=CARTESIAN_POINT('Ctrl Pts',(-0.394764232974746,-1.36375173596106,
-8.62722427512314));
#149247=CARTESIAN_POINT('Ctrl Pts',(-0.387463814108887,-1.36375173596304,
-8.62755213731119));
#149248=CARTESIAN_POINT('Ctrl Pts',(-0.374623090611251,-1.36375173596654,
-8.62812881486618));
#149249=CARTESIAN_POINT('Ctrl Pts',(-0.361994203322079,-1.36196031901124,
-8.63045948189725));
#149250=CARTESIAN_POINT('Ctrl Pts',(-0.338450424685215,-1.35499086531967,
-8.6383897484205));
#149251=CARTESIAN_POINT('Ctrl Pts',(-0.327788025201018,-1.34985996724206,
-8.64393209119935));
#149252=CARTESIAN_POINT('Ctrl Pts',(-0.312380524047814,-1.33873894481487,
-8.65562854990331));
#149253=CARTESIAN_POINT('Ctrl Pts',(-0.306902880703472,-1.33344492710504,
-8.66112049633992));
#149254=CARTESIAN_POINT('Ctrl Pts',(-0.302547006590512,-1.32768940181038,
-8.6670315812505));
#149255=CARTESIAN_POINT('Ctrl Pts',(-0.0570563368422518,-1.00000000016179,
-8.99981914104468));
#149256=CARTESIAN_POINT('Ctrl Pts',(-0.137825035508058,-1.10901473824052,
-8.89029016145374));
#149257=CARTESIAN_POINT('Ctrl Pts',(-0.21979267061258,-1.21834403196143,
-8.77933232408725));
#149258=CARTESIAN_POINT('Ctrl Pts',(-0.302547006027247,-1.32768940203058,
-8.66703158104983));
#149259=CARTESIAN_POINT('',(0.302547007,-1.32768940200002,-8.667031581));
#149260=CARTESIAN_POINT('Ctrl Pts',(0.302547007479098,-1.32768940183626,
-8.66703158119359));
#149261=CARTESIAN_POINT('Ctrl Pts',(0.219792522734841,-1.21834383445799,
-8.77933252688754));
#149262=CARTESIAN_POINT('Ctrl Pts',(0.137824974935765,-1.10901465433772,
-8.89029024572902));
#149263=CARTESIAN_POINT('Ctrl Pts',(0.0570563383027792,-0.999999999986948,
-8.99981914121027));
#149264=CARTESIAN_POINT('',(0.475577681,-1.32768940200002,-8.659260764));
#149265=CARTESIAN_POINT('Ctrl Pts',(0.302547006808484,-1.32768940209839,
-8.66703158095471));
#149266=CARTESIAN_POINT('Ctrl Pts',(0.305987908599573,-1.33223595155284,
-8.66236214793029));
#149267=CARTESIAN_POINT('Ctrl Pts',(0.310134107298286,-1.33650155483069,
-8.65794701589455));
#149268=CARTESIAN_POINT('Ctrl Pts',(0.323410372907643,-1.34730670115791,
-8.64665157582217));
#149269=CARTESIAN_POINT('Ctrl Pts',(0.333756811921418,-1.35293307637481,
-8.64063148394741));
#149270=CARTESIAN_POINT('Ctrl Pts',(0.351909751292211,-1.35917045608827,
-8.63366308668712));
#149271=CARTESIAN_POINT('Ctrl Pts',(0.358762435478143,-1.36087898853258,
-8.63167146500543));
#149272=CARTESIAN_POINT('Ctrl Pts',(0.372912936869227,-1.3631727423964,
-8.62877580004926));
#149273=CARTESIAN_POINT('Ctrl Pts',(0.380163395243691,-1.36375173596503,
-8.6278799994992));
#149274=CARTESIAN_POINT('Ctrl Pts',(0.38746381410889,-1.36375173596304,
-8.62755213731119));
#149275=CARTESIAN_POINT('Ctrl Pts',(0.400304537606769,-1.36375173595955,
-8.62697545975618));
#149276=CARTESIAN_POINT('Ctrl Pts',(0.413091504089368,-1.36196031899726,
-8.6281646994827));
#149277=CARTESIAN_POINT('Ctrl Pts',(0.437251366001841,-1.35499086529249,
-8.63395259304714));
#149278=CARTESIAN_POINT('Ctrl Pts',(0.448367653573957,-1.34985996720843,
-8.63851685386684));
#149279=CARTESIAN_POINT('Ctrl Pts',(0.46476159091214,-1.33873894491584,
-8.64878510818524));
#149280=CARTESIAN_POINT('Ctrl Pts',(0.470709476999128,-1.33344492738548,
-8.65376393332434));
#149281=CARTESIAN_POINT('Ctrl Pts',(0.475577681121842,-1.32768940229425,
-8.65926076420018));
#149282=CARTESIAN_POINT('Ctrl Pts',(0.749910923381227,-1.00000000008659,
-8.9687030057548));
#149283=CARTESIAN_POINT('Ctrl Pts',(0.659649273775833,-1.10901473822727,
-8.86685500789799));
#149284=CARTESIAN_POINT('Ctrl Pts',(0.56806543247335,-1.21834403201054,
-8.76369137626223));
#149285=CARTESIAN_POINT('Ctrl Pts',(0.475577680748767,-1.32768940214297,
-8.65926076437218));
#149286=CARTESIAN_POINT('',(1.07823576159075,-1.32768940191118,-8.60502055527693));
#149287=CARTESIAN_POINT('Ctrl Pts',(1.07823576225904,-1.32768940182398,
-8.60502055560242));
#149288=CARTESIAN_POINT('Ctrl Pts',(1.00588100192119,-1.21834383435451,
-8.72428746560445));
#149289=CARTESIAN_POINT('Ctrl Pts',(0.934189604625298,-1.10901465414413,
-8.84214601570619));
#149290=CARTESIAN_POINT('Ctrl Pts',(0.86356421329429,-0.999999999704432,
-8.95847402490167));
#149291=CARTESIAN_POINT('',(1.249873295,-1.32768940200002,-8.581770672));
#149292=CARTESIAN_POINT('Ctrl Pts',(1.07823576149091,-1.32768940211609,
-8.60502055540428));
#149293=CARTESIAN_POINT('Ctrl Pts',(1.08124424645351,-1.33223595151502,
-8.60006148014485));
#149294=CARTESIAN_POINT('Ctrl Pts',(1.08497798435395,-1.33650155474298,
-8.59529245980226));
#149295=CARTESIAN_POINT('Ctrl Pts',(1.09718828812373,-1.34730670103304,
-8.58285241662335));
#149296=CARTESIAN_POINT('Ctrl Pts',(1.10695343853787,-1.35293307625488,
-8.5759291122228));
#149297=CARTESIAN_POINT('Ctrl Pts',(1.12440865719429,-1.35917045597632,
-8.56736155073659));
#149298=CARTESIAN_POINT('Ctrl Pts',(1.13105522689639,-1.36087898842353,
-8.56476367686195));
#149299=CARTESIAN_POINT('Ctrl Pts',(1.14488919712257,-1.36317274229315,
-8.56061122783272));
#149300=CARTESIAN_POINT('Ctrl Pts',(1.15203016834082,-1.3637517358647,-8.5590691074326));
#149301=CARTESIAN_POINT('Ctrl Pts',(1.15927180852621,-1.36375173586557,
-8.55808816061781));
#149302=CARTESIAN_POINT('Ctrl Pts',(1.17200914606822,-1.36375173586709,
-8.55636277101395));
#149303=CARTESIAN_POINT('Ctrl Pts',(1.18485123861068,-1.36196031890982,
-8.55640100836933));
#149304=CARTESIAN_POINT('Ctrl Pts',(1.20943266280315,-1.35499086521458,
-8.55999992824462));
#149305=CARTESIAN_POINT('Ctrl Pts',(1.22091333665683,-1.34985996713517,
-8.56354935835334));
#149306=CARTESIAN_POINT('Ctrl Pts',(1.23816171620794,-1.3387389447467,-8.57230673456117));
#149307=CARTESIAN_POINT('Ctrl Pts',(1.24453195642251,-1.33344492708842,
-8.57673235212774));
#149308=CARTESIAN_POINT('Ctrl Pts',(1.2498732947827,-1.32768940185218,-8.58177067206148));
#149309=CARTESIAN_POINT('Ctrl Pts',(1.55084034118531,-1.00000000030594,
-8.86537614716069));
#149310=CARTESIAN_POINT('Ctrl Pts',(1.4518124743483,-1.10901473831009,-8.77202915141814));
#149311=CARTESIAN_POINT('Ctrl Pts',(1.35134980606936,-1.21834403195577,
-8.6774903386024));
#149312=CARTESIAN_POINT('Ctrl Pts',(1.24987329501287,-1.32768940194995,
-8.58177067192916));
#149313=CARTESIAN_POINT('',(1.845243197,-1.32768940200002,-8.473726964));
#149314=CARTESIAN_POINT('Ctrl Pts',(1.84524319784117,-1.32768940174229,
-8.47372696418715));
#149315=CARTESIAN_POINT('Ctrl Pts',(1.78387071989928,-1.21834383431894,
-8.59899957133592));
#149316=CARTESIAN_POINT('Ctrl Pts',(1.72303269008614,-1.1090146541547,-8.72281002482354));
#149317=CARTESIAN_POINT('Ctrl Pts',(1.66311917818115,-0.999999999760971,
-8.84500054287555));
#149318=CARTESIAN_POINT('',(2.014105665,-1.32768940200002,-8.435185207));
#149319=CARTESIAN_POINT('Ctrl Pts',(1.84524319731388,-1.32768940193905,
-8.4737269641006));
#149320=CARTESIAN_POINT('Ctrl Pts',(1.8477950429561,-1.33223595150089,-8.46851817393293));
#149321=CARTESIAN_POINT('Ctrl Pts',(1.85108625832112,-1.33650155487643,
-8.46343366240974));
#149322=CARTESIAN_POINT('Ctrl Pts',(1.86213229025263,-1.34730670128967,
-8.44994917584067));
#149323=CARTESIAN_POINT('Ctrl Pts',(1.87123752882059,-1.35293307651039,
-8.44217840129405));
#149324=CARTESIAN_POINT('Ctrl Pts',(1.88785448760806,-1.35917045623014,
-8.43208065655475));
#149325=CARTESIAN_POINT('Ctrl Pts',(1.89424142855602,-1.36087898867676,
-8.42889744704194));
#149326=CARTESIAN_POINT('Ctrl Pts',(1.9076474846242,-1.3631727425452,-8.42352164702133));
#149327=CARTESIAN_POINT('Ctrl Pts',(1.9146214737849,-1.36375173611614,-8.42134562301971));
#149328=CARTESIAN_POINT('Ctrl Pts',(1.92174602986137,-1.36375173611641,
-8.41971948958691));
#149329=CARTESIAN_POINT('Ctrl Pts',(1.9342774278958,-1.36375173611689,-8.41685927975983));
#149330=CARTESIAN_POINT('Ctrl Pts',(1.94707124951949,-1.36196031915855,
-8.41574620688258));
#149331=CARTESIAN_POINT('Ctrl Pts',(1.9718763208155,-1.35499086546122,-8.41712717668837));
#149332=CARTESIAN_POINT('Ctrl Pts',(1.98362894531339,-1.34985996738079,
-8.41963319816523));
#149333=CARTESIAN_POINT('Ctrl Pts',(2.00159289302696,-1.33873894504213,
-8.42680918689579));
#149334=CARTESIAN_POINT('Ctrl Pts',(2.00833419776163,-1.33344492744846,
-8.43064596424567));
#149335=CARTESIAN_POINT('Ctrl Pts',(2.01410566493822,-1.32768940228524,
-8.4351852074402));
#149336=CARTESIAN_POINT('Ctrl Pts',(2.33928330581808,-0.999999999832171,
-8.69067049301388));
#149337=CARTESIAN_POINT('Ctrl Pts',(2.23228653562601,-1.10901473810327,
-8.60657607417562));
#149338=CARTESIAN_POINT('Ctrl Pts',(2.12375390641409,-1.21834403201796,
-8.52142325077419));
#149339=CARTESIAN_POINT('Ctrl Pts',(2.01410566492906,-1.32768940228112,
-8.43518520744662));
#149340=CARTESIAN_POINT('',(2.59739382,-1.32768940200002,-8.274207905));
#149341=CARTESIAN_POINT('Ctrl Pts',(2.59739382005673,-1.32768940220199,
-8.27420790519125));
#149342=CARTESIAN_POINT('Ctrl Pts',(2.54749775952752,-1.21834383473538,
-8.40447758822955));
#149343=CARTESIAN_POINT('Ctrl Pts',(2.49800292915253,-1.10901465452695,
-8.53324309624464));
#149344=CARTESIAN_POINT('Ctrl Pts',(2.44928368495601,-1.00000000008883,
-8.66031231705933));
#149345=CARTESIAN_POINT('',(2.762121641,-1.32768940200002,-8.220684592));
#149346=CARTESIAN_POINT('Ctrl Pts',(2.59739381999827,-1.32768940222355,
-8.274207905187));
#149347=CARTESIAN_POINT('Ctrl Pts',(2.59946848029277,-1.33223595162173,
-8.26879133857389));
#149348=CARTESIAN_POINT('Ctrl Pts',(2.60229067402789,-1.33650155484869,
-8.26343227370456));
#149349=CARTESIAN_POINT('Ctrl Pts',(2.61208349771735,-1.34730670113423,
-8.24901191321329));
#149350=CARTESIAN_POINT('Ctrl Pts',(2.62045551441409,-1.35293307635233,
-8.24045623422956));
#149351=CARTESIAN_POINT('Ctrl Pts',(2.63610042335358,-1.35917045606773,
-8.22890960734339));
#149352=CARTESIAN_POINT('Ctrl Pts',(2.64217631165495,-1.36087898851275,
-8.22516669152493));
#149353=CARTESIAN_POINT('Ctrl Pts',(2.65504651588519,-1.36317274237799,
-8.21861082329637));
#149354=CARTESIAN_POINT('Ctrl Pts',(2.66179737252854,-1.36375173594733,
-8.21581841576039));
#149355=CARTESIAN_POINT('Ctrl Pts',(2.66874748175985,-1.36375173594603,
-8.21356018838122));
#149356=CARTESIAN_POINT('Ctrl Pts',(2.68097204483843,-1.36375173594376,
-8.209588187061));
#149357=CARTESIAN_POINT('Ctrl Pts',(2.69361458721409,-1.3619603189827,-8.20733276576193));
#149358=CARTESIAN_POINT('Ctrl Pts',(2.71844358976387,-1.35499086528025,
-8.20648466674613));
#149359=CARTESIAN_POINT('Ctrl Pts',(2.73037353968325,-1.34985996719732,
-8.20792710258216));
#149360=CARTESIAN_POINT('Ctrl Pts',(2.74890842063212,-1.33873894477132,
-8.2134639270796));
#149361=CARTESIAN_POINT('Ctrl Pts',(2.7559665130382,-1.33344492707015,-8.21668097286978));
#149362=CARTESIAN_POINT('Ctrl Pts',(2.76212164068402,-1.32768940178609,
-8.22068459217825));
#149363=CARTESIAN_POINT('Ctrl Pts',(3.10889173601996,-1.00000000022005,
-8.44599266929271));
#149364=CARTESIAN_POINT('Ctrl Pts',(2.99478753806051,-1.10901473827084,
-8.37182790653101));
#149365=CARTESIAN_POINT('Ctrl Pts',(2.87905878935271,-1.21834403196375,
-8.29674667337776));
#149366=CARTESIAN_POINT('Ctrl Pts',(2.76212164114016,-1.32768940200595,
-8.22068459179305));
#149367=CARTESIAN_POINT('',(3.328631754,-1.32768940200002,-8.00806979));
#149368=CARTESIAN_POINT('Ctrl Pts',(3.32863175341881,-1.32768940231455,
-8.00806979009162));
#149369=CARTESIAN_POINT('Ctrl Pts',(3.29061384423879,-1.21834383487424,
-8.14228769397692));
#149370=CARTESIAN_POINT('Ctrl Pts',(3.25286071676859,-1.10901465469334,
-8.27497151221575));
#149371=CARTESIAN_POINT('Ctrl Pts',(3.21572799918201,-1.00000000028271,
-8.40589634900338));
#149372=CARTESIAN_POINT('',(3.487898636,-1.32768940200002,-7.939995858));
#149373=CARTESIAN_POINT('Ctrl Pts',(3.32863175374707,-1.32768940219362,
-8.00806979008612));
#149374=CARTESIAN_POINT('Ctrl Pts',(3.3302125247748,-1.33223595146223,-8.00248905800613));
#149375=CARTESIAN_POINT('Ctrl Pts',(3.3325429742706,-1.33650155457232,-7.99689858780651));
#149376=CARTESIAN_POINT('Ctrl Pts',(3.34100374369261,-1.34730670076621,
-7.9816584576379));
#149377=CARTESIAN_POINT('Ctrl Pts',(3.3485751319546,-1.35293307599116,-7.97238675950792));
#149378=CARTESIAN_POINT('Ctrl Pts',(3.36312202742944,-1.35917045571755,
-7.95948421711507));
#149379=CARTESIAN_POINT('Ctrl Pts',(3.3688379436014,-1.36087898816654,-7.95521173074453));
#149380=CARTESIAN_POINT('Ctrl Pts',(3.38106867267251,-1.36317274203974,
-7.94752857829612));
#149381=CARTESIAN_POINT('Ctrl Pts',(3.38754204286877,-1.36375173561308,
-7.94414227004508));
#149382=CARTESIAN_POINT('Ctrl Pts',(3.39426174706129,-1.36375173561571,
-7.94127013063417));
#149383=CARTESIAN_POINT('Ctrl Pts',(3.40608105018694,-1.36375173562033,
-7.93621831803287));
#149384=CARTESIAN_POINT('Ctrl Pts',(3.4184705229962,-1.3619603186662,-7.9328387076302));
#149385=CARTESIAN_POINT('Ctrl Pts',(3.44312354827156,-1.35499086497692,
-7.9297683681713));
#149386=CARTESIAN_POINT('Ctrl Pts',(3.45513477067234,-1.34985996690042,
-7.93013560471274));
#149387=CARTESIAN_POINT('Ctrl Pts',(3.47409135267749,-1.33873894453579,
-7.9339886856354));
#149388=CARTESIAN_POINT('Ctrl Pts',(3.48140940496856,-1.33344492690381,
-7.93656009797619));
#149389=CARTESIAN_POINT('Ctrl Pts',(3.48789863549779,-1.32768940169679,
-7.93999585844057));
#149390=CARTESIAN_POINT('Ctrl Pts',(3.8534691968536,-1.00000000021841,-8.13331267965086));
#149391=CARTESIAN_POINT('Ctrl Pts',(3.73317627069964,-1.10901473822962,
-8.06967470393504));
#149392=CARTESIAN_POINT('Ctrl Pts',(3.61118318198707,-1.21834403188242,
-8.00526957087236));
#149393=CARTESIAN_POINT('Ctrl Pts',(3.48789863585382,-1.32768940188326,
-7.93999585808051));
#149394=CARTESIAN_POINT('',(4.033069504,-1.32768940200002,-7.677455405));
#149395=CARTESIAN_POINT('Ctrl Pts',(4.03306950415229,-1.327689401891,-7.67745540494174));
#149396=CARTESIAN_POINT('Ctrl Pts',(4.00723584390748,-1.2183438344254,-7.81454088623289));
#149397=CARTESIAN_POINT('Ctrl Pts',(3.98152838506235,-1.1090146542176,-7.9500747228005));
#149398=CARTESIAN_POINT('Ctrl Pts',(3.95628116463242,-0.999999999779801,
-8.08380104593988));
#149399=CARTESIAN_POINT('',(4.185593123,-1.32768940200002,-7.595378945));
#149400=CARTESIAN_POINT('Ctrl Pts',(4.03306950367076,-1.32768940206931,
-7.67745540499327));
#149401=CARTESIAN_POINT('Ctrl Pts',(4.03414365800827,-1.33223595145271,
-7.67175543994931));
#149402=CARTESIAN_POINT('Ctrl Pts',(4.03596359994506,-1.3365015546661,-7.66597857532337));
#149403=CARTESIAN_POINT('Ctrl Pts',(4.04302419413378,-1.34730670093839,
-7.65004137978483));
#149404=CARTESIAN_POINT('Ctrl Pts',(4.04973399360729,-1.35293307615463,
-7.64012831277831));
#149405=CARTESIAN_POINT('Ctrl Pts',(4.06306575258348,-1.3591704558669,-7.6259737385784));
#149406=CARTESIAN_POINT('Ctrl Pts',(4.0683756754347,-1.36087898831075,-7.62120608120941));
#149407=CARTESIAN_POINT('Ctrl Pts',(4.07986845471533,-1.36317274217366,
-7.61245750477902));
#149408=CARTESIAN_POINT('Ctrl Pts',(4.08601221869675,-1.36375173574184,
-7.60850456038225));
#149409=CARTESIAN_POINT('Ctrl Pts',(4.09244741474498,-1.36375173573942,
-7.60504163372406));
#149410=CARTESIAN_POINT('Ctrl Pts',(4.10376629584433,-1.36375173573516,
-7.59895068407685));
#149411=CARTESIAN_POINT('Ctrl Pts',(4.11580294633933,-1.36196031877213,
-7.59447409521846));
#149412=CARTESIAN_POINT('Ctrl Pts',(4.1400815026765,-1.35499086506602,-7.58920623590949));
#149413=CARTESIAN_POINT('Ctrl Pts',(4.15207729025624,-1.3498599669813,-7.5884953163971));
#149414=CARTESIAN_POINT('Ctrl Pts',(4.17130294590846,-1.33873894473932,
-7.59063363102621));
#149415=CARTESIAN_POINT('Ctrl Pts',(4.17882203729309,-1.33344492727405,
-7.59253870638845));
#149416=CARTESIAN_POINT('Ctrl Pts',(4.1855931231253,-1.32768940225633,-7.59537894522069));
#149417=CARTESIAN_POINT('Ctrl Pts',(4.5670207909907,-1.00000000006023,-7.75514803814697));
#149418=CARTESIAN_POINT('Ctrl Pts',(4.44150766456477,-1.10901473824446,
-7.7025492248208));
#149419=CARTESIAN_POINT('Ctrl Pts',(4.31423245247801,-1.21834403207158,
-7.64933874389548));
#149420=CARTESIAN_POINT('Ctrl Pts',(4.18559312311082,-1.32768940224795,
-7.59537894523824));
#149421=CARTESIAN_POINT('',(4.705035349,-1.32768940200002,-7.285026664));
#149422=CARTESIAN_POINT('Ctrl Pts',(4.70503534876328,-1.32768940166455,
-7.2850266637129));
#149423=CARTESIAN_POINT('Ctrl Pts',(4.6915939350508,-1.21834383431014,-7.42387599047203));
#149424=CARTESIAN_POINT('Ctrl Pts',(4.67813912632766,-1.10901465421366,
-7.56116860636961));
#149425=CARTESIAN_POINT('Ctrl Pts',(4.66498067897969,-0.999999999886531,
-7.69661972990669));
#149426=CARTESIAN_POINT('',(4.849587676,-1.32768940200002,-7.189608507));
#149427=CARTESIAN_POINT('Ctrl Pts',(4.70503534864306,-1.32768940170967,
-7.28502666373683));
#149428=CARTESIAN_POINT('Ctrl Pts',(4.70559423778768,-1.33223595129556,
-7.27925335840597));
#149429=CARTESIAN_POINT('Ctrl Pts',(4.70688901904333,-1.33650155469243,
-7.27333661116776));
#149430=CARTESIAN_POINT('Ctrl Pts',(4.71249259024252,-1.34730670111821,
-7.25683066707283));
#149431=CARTESIAN_POINT('Ctrl Pts',(4.71828677756059,-1.35293307633343,
-7.24635604537204));
#149432=CARTESIAN_POINT('Ctrl Pts',(4.73029606054557,-1.35917045604412,
-7.23106340366536));
#149433=CARTESIAN_POINT('Ctrl Pts',(4.7351572376969,-1.36087898848742,-7.22583896166848));
#149434=CARTESIAN_POINT('Ctrl Pts',(4.74581953408189,-1.3631727423492,-7.21609539964254));
#149435=CARTESIAN_POINT('Ctrl Pts',(4.75158422587189,-1.36375173591681,
-7.21160764588035));
#149436=CARTESIAN_POINT('Ctrl Pts',(4.75768310136027,-1.36375173591383,
-7.20758181342034));
#149437=CARTESIAN_POINT('Ctrl Pts',(4.76841042745519,-1.36375173590859,
-7.20050076746617));
#149438=CARTESIAN_POINT('Ctrl Pts',(4.77999734360255,-1.36196031894456,
-7.19496324300642));
#149439=CARTESIAN_POINT('Ctrl Pts',(4.80370595434181,-1.35499086523651,
-7.18754027753896));
#149440=CARTESIAN_POINT('Ctrl Pts',(4.81558972407363,-1.34985996715085,
-7.18575692587117));
#149441=CARTESIAN_POINT('Ctrl Pts',(4.83492966004747,-1.33873894484204,
-7.18616325779104));
#149442=CARTESIAN_POINT('Ctrl Pts',(4.84258925152042,-1.33344492729325,
-7.18738665775673));
#149443=CARTESIAN_POINT('Ctrl Pts',(4.84958767607709,-1.32768940218149,
-7.18960850722728));
#149444=CARTESIAN_POINT('Ctrl Pts',(5.24380141911386,-1.00000000018046,
-7.31454350411914));
#149445=CARTESIAN_POINT('Ctrl Pts',(5.11407865044419,-1.10901473830268,
-7.27340734808659));
#149446=CARTESIAN_POINT('Ctrl Pts',(4.98254606029434,-1.21834403206745,
-7.23181993899048));
#149447=CARTESIAN_POINT('Ctrl Pts',(4.8495876760775,-1.32768940218176,-7.18960850722668));
#149448=CARTESIAN_POINT('',(5.339119013,-1.32768940200002,-6.833943172));
#149449=CARTESIAN_POINT('Ctrl Pts',(5.33911901336203,-1.3276894020463,-6.83394317203872));
#149450=CARTESIAN_POINT('Ctrl Pts',(5.33817806862294,-1.21834383468527,
-6.9734384111691));
#149451=CARTESIAN_POINT('Ctrl Pts',(5.33708424031203,-1.10901465458379,
-7.11138440702185));
#149452=CARTESIAN_POINT('Ctrl Pts',(5.33612051020986,-1.00000000025242,
-7.2474697581966));
#149453=CARTESIAN_POINT('',(5.474536199,-1.32768940200002,-6.725951571));
#149454=CARTESIAN_POINT('Ctrl Pts',(5.33911901311747,-1.32768940214016,
-6.83394317211068));
#149455=CARTESIAN_POINT('Ctrl Pts',(5.33915813729677,-1.33223595149941,
-6.82814301021648));
#149456=CARTESIAN_POINT('Ctrl Pts',(5.33991733300375,-1.33650155469162,
-6.82213401903261));
#149457=CARTESIAN_POINT('Ctrl Pts',(5.34401876437183,-1.34730670095398,
-6.80519222304139));
#149458=CARTESIAN_POINT('Ctrl Pts',(5.34885068813799,-1.35293307617826,
-6.79424038213927));
#149459=CARTESIAN_POINT('Ctrl Pts',(5.3594408034379,-1.35917045590364,-6.77793280028018));
#149460=CARTESIAN_POINT('Ctrl Pts',(5.3638140955464,-1.36087898835228,-6.77229363778862));
#149461=CARTESIAN_POINT('Ctrl Pts',(5.37356006248997,-1.36317274222478,
-6.76163353959512));
#149462=CARTESIAN_POINT('Ctrl Pts',(5.37889926817801,-1.36375173579776,
-6.75664710921954));
#149463=CARTESIAN_POINT('Ctrl Pts',(5.38461271854601,-1.36375173580003,
-6.75209078459071));
#149464=CARTESIAN_POINT('Ctrl Pts',(5.39466211951056,-1.36375173580403,
-6.74407665474437));
#149465=CARTESIAN_POINT('Ctrl Pts',(5.40570601027228,-1.36196031884925,
-6.73752277956918));
#149466=CARTESIAN_POINT('Ctrl Pts',(5.42865378761812,-1.35499086515872,
-6.7280044732854));
#149467=CARTESIAN_POINT('Ctrl Pts',(5.44032985837541,-1.3498599670816,-6.72516304795477));
#149468=CARTESIAN_POINT('Ctrl Pts',(5.4596283610753,-1.33873894460838,-6.72383412557344));
#149469=CARTESIAN_POINT('Ctrl Pts',(5.46736678229439,-1.33344492683944,
-6.72436600006062));
#149470=CARTESIAN_POINT('Ctrl Pts',(5.47453619853397,-1.32768940147805,
-6.72595157121251));
#149471=CARTESIAN_POINT('Ctrl Pts',(5.87836203986568,-0.99999999994125,
-6.81504656838998));
#149472=CARTESIAN_POINT('Ctrl Pts',(5.74547408034092,-1.10901473795678,
-6.78570427387046));
#149473=CARTESIAN_POINT('Ctrl Pts',(5.61074313513168,-1.21834403161385,
-6.75607477404509));
#149474=CARTESIAN_POINT('Ctrl Pts',(5.47453619872126,-1.32768940161921,
-6.72595157087805));
#149475=CARTESIAN_POINT('',(5.93021523354241,-1.32768940189191,-6.32783678686984));
#149476=CARTESIAN_POINT('Ctrl Pts',(5.93021523412515,-1.32768940176286,
-6.32783678671984));
#149477=CARTESIAN_POINT('Ctrl Pts',(5.94178233414468,-1.21834383430549,
-6.46685480485237));
#149478=CARTESIAN_POINT('Ctrl Pts',(5.95305829295893,-1.10901465410688,
-6.60434352087773));
#149479=CARTESIAN_POINT('Ctrl Pts',(5.96429703934163,-0.999999999678913,
-6.73996742071358));
#149480=CARTESIAN_POINT('',(6.055406976,-1.32768940200002,-6.208141225));
#149481=CARTESIAN_POINT('Ctrl Pts',(5.93021523353202,-1.32768940199765,
-6.32783678695391));
#149482=CARTESIAN_POINT('Ctrl Pts',(5.92973427764573,-1.33223595152411,
-6.32205646756782));
#149483=CARTESIAN_POINT('Ctrl Pts',(5.92995177522348,-1.33650155486745,
-6.31600361284212));
#149484=CARTESIAN_POINT('Ctrl Pts',(5.93251804458815,-1.34730670125214,
-6.29876236986104));
#149485=CARTESIAN_POINT('Ctrl Pts',(5.93634880100404,-1.3529330764714,-6.28742148754437));
#149486=CARTESIAN_POINT('Ctrl Pts',(5.94543448325041,-1.35917045618876,
-6.27023026460103));
#149487=CARTESIAN_POINT('Ctrl Pts',(5.94928467914374,-1.3608789886345,-6.26422178483839));
#149488=CARTESIAN_POINT('Ctrl Pts',(5.95803584785762,-1.36317274250118,
-6.25273097932687));
#149489=CARTESIAN_POINT('Ctrl Pts',(5.9629065793017,-1.36375173607124,-6.24728602014728));
#149490=CARTESIAN_POINT('Ctrl Pts',(5.96818860320827,-1.36375173607065,
-6.24223588820087));
#149491=CARTESIAN_POINT('Ctrl Pts',(5.97747916718049,-1.36375173606962,
-6.23335319952962));
#149492=CARTESIAN_POINT('Ctrl Pts',(5.98789111364513,-1.36196031910978,
-6.22583574159617));
#149493=CARTESIAN_POINT('Ctrl Pts',(6.00989329559082,-1.3549908654096,-6.21429873031895));
#149494=CARTESIAN_POINT('Ctrl Pts',(6.02126765851761,-1.34985996732779,
-6.21042210882142));
#149495=CARTESIAN_POINT('Ctrl Pts',(6.0403693472299,-1.33873894496681,-6.20736863188564));
#149496=CARTESIAN_POINT('Ctrl Pts',(6.04812429250932,-1.33344492734667,
-6.20720469845112));
#149497=CARTESIAN_POINT('Ctrl Pts',(6.05540697612596,-1.32768940215382,
-6.20814122496572));
#149498=CARTESIAN_POINT('Ctrl Pts',(6.46559354791635,-0.999999999885752,
-6.26067888293268));
#149499=CARTESIAN_POINT('Ctrl Pts',(6.33061033303081,-1.10901473812568,
-6.24336669663294));
#149500=CARTESIAN_POINT('Ctrl Pts',(6.19376580688884,-1.21834403200888,
-6.22593366519494));
#149501=CARTESIAN_POINT('Ctrl Pts',(6.05540697622248,-1.32768940224085,
-6.20814122474999));
#149502=CARTESIAN_POINT('',(6.473564847,-1.32768940200002,-5.770782381));
#149503=CARTESIAN_POINT('Ctrl Pts',(6.47356484705234,-1.32768940202094,
-5.77078238100751));
#149504=CARTESIAN_POINT('Ctrl Pts',(6.49754686040969,-1.21834383453442,
-5.90820388664413));
#149505=CARTESIAN_POINT('Ctrl Pts',(6.52110181902666,-1.10901465430654,
-6.04412834439049));
#149506=CARTESIAN_POINT('Ctrl Pts',(6.54445255418411,-0.999999999849283,
-6.17819882884537));
#149507=CARTESIAN_POINT('',(6.587523177,-1.32768940200002,-5.640346578));
#149508=CARTESIAN_POINT('Ctrl Pts',(6.47356484669524,-1.32768940216809,
-5.77078238118696));
#149509=CARTESIAN_POINT('Ctrl Pts',(6.47256768322408,-1.33223595155632,
-5.76506844435757));
#149510=CARTESIAN_POINT('Ctrl Pts',(6.47224173153327,-1.33650155477443,
-5.75902046047074));
#149511=CARTESIAN_POINT('Ctrl Pts',(6.47325217673578,-1.34730670105451,
-5.74161858722322));
#149512=CARTESIAN_POINT('Ctrl Pts',(6.47605092279891,-1.35293307627464,
-5.7299799736068));
#149513=CARTESIAN_POINT('Ctrl Pts',(6.48355901941539,-1.3591704559933,-5.71204352319526));
#149514=CARTESIAN_POINT('Ctrl Pts',(6.48685511957833,-1.3608789884395,-5.70571410290666));
#149515=CARTESIAN_POINT('Ctrl Pts',(6.49454103079465,-1.36317274230711,
-5.69348510728424));
#149516=CARTESIAN_POINT('Ctrl Pts',(6.49890407172791,-1.36375173587764,
-5.68762545890897));
#149517=CARTESIAN_POINT('Ctrl Pts',(6.50371214142148,-1.36375173587751,
-5.6821221803364));
#149518=CARTESIAN_POINT('Ctrl Pts',(6.51216906624052,-1.36375173587729,
-5.67244245102451));
#149519=CARTESIAN_POINT('Ctrl Pts',(6.52186523753564,-1.36196031891828,
-5.6640219364811));
#149520=CARTESIAN_POINT('Ctrl Pts',(6.54274467544732,-1.35499086521973,
-5.65055910943509));
#149521=CARTESIAN_POINT('Ctrl Pts',(6.55372575086094,-1.3498599671387,-5.64567850404373));
#149522=CARTESIAN_POINT('Ctrl Pts',(6.57247683027915,-1.33873894474861,
-5.64092505731962));
#149523=CARTESIAN_POINT('Ctrl Pts',(6.58018586159814,-1.33344492709045,
-5.64006663589892));
#149524=CARTESIAN_POINT('Ctrl Pts',(6.58752317690413,-1.3276894018546,-5.64034657752293));
#149525=CARTESIAN_POINT('Ctrl Pts',(7.00076789692398,-0.999999999893325,
-5.65590389374846));
#149526=CARTESIAN_POINT('Ctrl Pts',(6.86477623251869,-1.10901473799573,
-5.65076120332882));
#149527=CARTESIAN_POINT('Ctrl Pts',(6.72691991747828,-1.21834403174059,
-5.64566500091207));
#149528=CARTESIAN_POINT('Ctrl Pts',(6.58752317688628,-1.32768940183436,
-5.64034657757489));
#149529=CARTESIAN_POINT('',(6.964793123,-1.32768940200002,-5.167265029));
#149530=CARTESIAN_POINT('Ctrl Pts',(6.9647931225424,-1.32768940189471,-5.1672650290375));
#149531=CARTESIAN_POINT('Ctrl Pts',(7.00099696010947,-1.21834383456653,
-5.3019835847847));
#149532=CARTESIAN_POINT('Ctrl Pts',(7.03664126779649,-1.10901465449722,
-5.43524940021246));
#149533=CARTESIAN_POINT('Ctrl Pts',(7.07191598528383,-1.00000000019748,
-5.56668701235598));
#149534=CARTESIAN_POINT('',(7.066600514,-1.32768940200002,-5.027139175));
#149535=CARTESIAN_POINT('Ctrl Pts',(6.96479312275204,-1.32768940180384,
-5.16726502890744));
#149536=CARTESIAN_POINT('Ctrl Pts',(6.96328778019254,-1.3322359512407,-5.1616634797066));
#149537=CARTESIAN_POINT('Ctrl Pts',(6.96242100357658,-1.33650155450292,
-5.155669061255));
#149538=CARTESIAN_POINT('Ctrl Pts',(6.9618674891292,-1.34730670082041,-5.13824666716368));
#149539=CARTESIAN_POINT('Ctrl Pts',(6.96361169098159,-1.35293307604079,
-5.12640402952091));
#149540=CARTESIAN_POINT('Ctrl Pts',(6.96948175118831,-1.35917045575974,
-5.10786676539326));
#149541=CARTESIAN_POINT('Ctrl Pts',(6.97219721736018,-1.36087898820603,
-5.10126736534917));
#149542=CARTESIAN_POINT('Ctrl Pts',(6.97875598864058,-1.3631727420738,-5.08839864029793));
#149543=CARTESIAN_POINT('Ctrl Pts',(6.98257621042259,-1.36375173564443,
-5.08217148117021));
#149544=CARTESIAN_POINT('Ctrl Pts',(6.9868716141528,-1.36375173564439,-5.07625936513457));
#149545=CARTESIAN_POINT('Ctrl Pts',(6.9944268096322,-1.36375173564433,-5.06586053067067));
#149546=CARTESIAN_POINT('Ctrl Pts',(7.00332913788735,-1.36196031868552,
-5.05660475654901));
#149547=CARTESIAN_POINT('Ctrl Pts',(7.02291772280707,-1.35499086498739,
-5.04132450850107));
#149548=CARTESIAN_POINT('Ctrl Pts',(7.03341709754474,-1.34985996690657,
-5.0354792149805));
#149549=CARTESIAN_POINT('Ctrl Pts',(7.05166659470129,-1.33873894466852,
-5.02906407052158));
#149550=CARTESIAN_POINT('Ctrl Pts',(7.05926764317834,-1.33344492720299,
-5.02751807262591));
#149551=CARTESIAN_POINT('Ctrl Pts',(7.06660051416279,-1.32768940218439,
-5.0271391753499));
#149552=CARTESIAN_POINT('Ctrl Pts',(7.47957617995657,-0.999999999937531,
-5.00559089112874));
#149553=CARTESIAN_POINT('Ctrl Pts',(7.34367099065878,-1.1090147381492,-5.0126591024965));
#149554=CARTESIAN_POINT('Ctrl Pts',(7.20591282440991,-1.2183440320037,-5.01994076071516));
#149555=CARTESIAN_POINT('Ctrl Pts',(7.06660051417724,-1.32768940220666,
-5.02713917529117));
#149556=CARTESIAN_POINT('',(7.399944979,-1.32768940200002,-4.522143897));
#149557=CARTESIAN_POINT('Ctrl Pts',(7.39994497873908,-1.32768940215641,
-4.52214389722653));
#149558=CARTESIAN_POINT('Ctrl Pts',(7.44807914856806,-1.21834383484025,
-4.65307482860847));
#149559=CARTESIAN_POINT('Ctrl Pts',(7.495525818383,-1.1090146547835,-4.78260902385036));
#149560=CARTESIAN_POINT('Ctrl Pts',(7.5424405069824,-1.00000000049598,-4.9103555054297));
#149561=CARTESIAN_POINT('',(7.488781739,-1.32768940200002,-4.373456206));
#149562=CARTESIAN_POINT('Ctrl Pts',(7.39994497860661,-1.32768940221744,
-4.52214389732625));
#149563=CARTESIAN_POINT('Ctrl Pts',(7.39794357718913,-1.33223595153308,
-4.5166998362934));
#149564=CARTESIAN_POINT('Ctrl Pts',(7.39654295448025,-1.33650155468582,
-4.51080724699965));
#149565=CARTESIAN_POINT('Ctrl Pts',(7.39442993696486,-1.34730670091578,
-4.49350460715019));
#149566=CARTESIAN_POINT('Ctrl Pts',(7.39510555131524,-1.35293307614091,
-4.48155329543663));
#149567=CARTESIAN_POINT('Ctrl Pts',(7.39929031283406,-1.35917045586763,
-4.46256446874343));
#149568=CARTESIAN_POINT('Ctrl Pts',(7.40140328167635,-1.36087898831677,
-4.45574822343214));
#149569=CARTESIAN_POINT('Ctrl Pts',(7.40678210564818,-1.36317274219025,
-4.44234338035808));
#149570=CARTESIAN_POINT('Ctrl Pts',(7.41002875009816,-1.36375173576373,
-4.43579884790072));
#149571=CARTESIAN_POINT('Ctrl Pts',(7.41377690379883,-1.36375173576648,
-4.42952549528285));
#149572=CARTESIAN_POINT('Ctrl Pts',(7.42036953994479,-1.36375173577133,
-4.41849128096622));
#149573=CARTESIAN_POINT('Ctrl Pts',(7.42840634884571,-1.36196031881741,
-4.40847476931493));
#149574=CARTESIAN_POINT('Ctrl Pts',(7.44654636500287,-1.3549908651285,-4.39150012783264));
#149575=CARTESIAN_POINT('Ctrl Pts',(7.45647950427152,-1.34985996705217,
-4.3847372090463));
#149576=CARTESIAN_POINT('Ctrl Pts',(7.47408048527613,-1.33873894477316,
-4.37671201771834));
#149577=CARTESIAN_POINT('Ctrl Pts',(7.48151235206002,-1.3334449272496,-4.37449089080897));
#149578=CARTESIAN_POINT('Ctrl Pts',(7.48878173904294,-1.32768940216483,
-4.37345620538491));
#149579=CARTESIAN_POINT('Ctrl Pts',(7.89816331290478,-0.999999999857504,
-4.31497581514083));
#149580=CARTESIAN_POINT('Ctrl Pts',(7.76343882751087,-1.10901473804168,
-4.3341980192771));
#149581=CARTESIAN_POINT('Ctrl Pts',(7.62688795793262,-1.21834403186849,
-4.35379891056257));
#149582=CARTESIAN_POINT('Ctrl Pts',(7.48878173899302,-1.32768940204296,
-4.37345620571204));
#149583=CARTESIAN_POINT('',(7.77551683,-1.32768940200002,-3.840613121));
#149584=CARTESIAN_POINT('Ctrl Pts',(7.77551682982721,-1.32768940206457,
-3.84061312113776));
#149585=CARTESIAN_POINT('Ctrl Pts',(7.83519378383851,-1.21834383471285,
-3.96670224946581));
#149586=CARTESIAN_POINT('Ctrl Pts',(7.89406080304461,-1.10901465462005,
-4.09146189152694));
#149587=CARTESIAN_POINT('Ctrl Pts',(7.952237733216,-1.00000000029693,-4.21448870316095));
#149588=CARTESIAN_POINT('',(7.85066769791133,-1.32768940203921,-3.68456073648916));
#149589=CARTESIAN_POINT('Ctrl Pts',(7.77551682988423,-1.32768940203625,
-3.84061312108626));
#149590=CARTESIAN_POINT('Ctrl Pts',(7.77303548357002,-1.33223595146919,
-3.83537038038258));
#149591=CARTESIAN_POINT('Ctrl Pts',(7.77111229166754,-1.33650155472793,
-3.82962706364747));
#149592=CARTESIAN_POINT('Ctrl Pts',(7.76745678383559,-1.34730670104337,
-3.81258348842368));
#149593=CARTESIAN_POINT('Ctrl Pts',(7.76705837104186,-1.35293307626466,
-3.80061972757348));
#149594=CARTESIAN_POINT('Ctrl Pts',(7.76952414064379,-1.3591704559852,-3.78133222518373));
#149595=CARTESIAN_POINT('Ctrl Pts',(7.77101759977719,-1.36087898843209,
-3.77435401500558));
#149596=CARTESIAN_POINT('Ctrl Pts',(7.77517316931867,-1.36317274230107,
-3.76052098182607));
#149597=CARTESIAN_POINT('Ctrl Pts',(7.77782009636727,-1.36375173587229,
-3.75371176876821));
#149598=CARTESIAN_POINT('Ctrl Pts',(7.78099082211098,-1.36375173587283,
-3.74712768891714));
#149599=CARTESIAN_POINT('Ctrl Pts',(7.78656781889864,-1.36375173587379,
-3.73554693575616));
#149600=CARTESIAN_POINT('Ctrl Pts',(7.79367440078957,-1.36196031891597,
-3.7248503336419));
#149601=CARTESIAN_POINT('Ctrl Pts',(7.8102197954466,-1.35499086521966,-3.70631796856791));
#149602=CARTESIAN_POINT('Ctrl Pts',(7.81950672345209,-1.34985996713973,
-3.69869187556752));
#149603=CARTESIAN_POINT('Ctrl Pts',(7.83631747555383,-1.33873894480565,
-3.68912125148975));
#149604=CARTESIAN_POINT('Ctrl Pts',(7.8435203236244,-1.33344492721707,-3.6862428787659));
#149605=CARTESIAN_POINT('Ctrl Pts',(7.85066769778106,-1.32768940205954,
-3.68456073586607));
#149606=CARTESIAN_POINT('Ctrl Pts',(8.25315907915067,-1.0000000002333,-3.58961908982468));
#149607=CARTESIAN_POINT('Ctrl Pts',(8.12070002029395,-1.10901473821362,
-3.62084052066841));
#149608=CARTESIAN_POINT('Ctrl Pts',(7.98645587500192,-1.21834403183509,
-3.65260282999209));
#149609=CARTESIAN_POINT('Ctrl Pts',(7.85066769773846,-1.327689401805,-3.68456073655596));
#149610=CARTESIAN_POINT('',(8.088484791,-1.32768940200002,-3.128159987));
#149611=CARTESIAN_POINT('Ctrl Pts',(8.08848479089928,-1.32768940204577,
-3.12815998710087));
#149612=CARTESIAN_POINT('Ctrl Pts',(8.15922404537986,-1.21834383466874,
-3.2483921167694));
#149613=CARTESIAN_POINT('Ctrl Pts',(8.2290374513845,-1.10901465455067,-3.3673727142875));
#149614=CARTESIAN_POINT('Ctrl Pts',(8.29800821672838,-1.00000000020229,
-3.48468931634764));
#149615=CARTESIAN_POINT('',(8.14934469545831,-1.32768940190648,-2.96599935139841));
#149616=CARTESIAN_POINT('Ctrl Pts',(8.08848479065033,-1.32768940218081,
-3.12815998737019));
#149617=CARTESIAN_POINT('Ctrl Pts',(8.08554347786003,-1.33223595160539,
-3.1231607785749));
#149618=CARTESIAN_POINT('Ctrl Pts',(8.08311320122475,-1.33650155485665,
-3.11761297634637));
#149619=CARTESIAN_POINT('Ctrl Pts',(8.07794463509115,-1.3473067011667,-3.10096569075218));
#149620=CARTESIAN_POINT('Ctrl Pts',(8.07647540293555,-1.35293307638893,
-3.08908580593355));
#149621=CARTESIAN_POINT('Ctrl Pts',(8.07720232768916,-1.35917045611106,
-3.06965491947504));
#149622=CARTESIAN_POINT('Ctrl Pts',(8.07806425265739,-1.36087898855854,
-3.06257092887487));
#149623=CARTESIAN_POINT('Ctrl Pts',(8.08096310956339,-1.3631727424287,-3.04842108103817));
#149624=CARTESIAN_POINT('Ctrl Pts',(8.08298900770923,-1.36375173600051,
-3.04140201115875));
#149625=CARTESIAN_POINT('Ctrl Pts',(8.08555677667574,-1.36375173600163,
-3.03456021521294));
#149626=CARTESIAN_POINT('Ctrl Pts',(8.09007323140408,-1.3637517360036,-3.02252616462162));
#149627=CARTESIAN_POINT('Ctrl Pts',(8.09619236826459,-1.36196031904678,
-3.01123559479314));
#149628=CARTESIAN_POINT('Ctrl Pts',(8.11100992762966,-1.35499086535231,
-2.99129471782952));
#149629=CARTESIAN_POINT('Ctrl Pts',(8.11957587148718,-1.34985996727328,
-2.98286685142905));
#149630=CARTESIAN_POINT('Ctrl Pts',(8.13546104438257,-1.33873894489342,
-2.97182785162225));
#149631=CARTESIAN_POINT('Ctrl Pts',(8.14237688063509,-1.33344492724556,
-2.96831540803315));
#149632=CARTESIAN_POINT('Ctrl Pts',(8.14934469550913,-1.327689402021,-2.96599935126671));
#149633=CARTESIAN_POINT('Ctrl Pts',(8.54170526199855,-0.99999999983659,
-2.83536086241028));
#149634=CARTESIAN_POINT('Ctrl Pts',(8.41257811164622,-1.10901473799347,
-2.87833014352137));
#149635=CARTESIAN_POINT('Ctrl Pts',(8.28172154505887,-1.21834403179278,
-2.92199813961197));
#149636=CARTESIAN_POINT('Ctrl Pts',(8.14934469551528,-1.32768940194035,
-2.96599935148564));
#149637=CARTESIAN_POINT('',(8.336329029,-1.32768940200002,-2.390520747));
#149638=CARTESIAN_POINT('Ctrl Pts',(8.33632902896119,-1.32768940187385,
-2.39052074690614));
#149639=CARTESIAN_POINT('Ctrl Pts',(8.41756103301672,-1.21834383447248,
-2.50392783959535));
#149640=CARTESIAN_POINT('Ctrl Pts',(8.49775872931061,-1.10901465432932,
-2.61617143085006));
#149641=CARTESIAN_POINT('Ctrl Pts',(8.57696801776182,-0.999999999956055,
-2.72683325912718));
#149642=CARTESIAN_POINT('',(8.382407962,-1.32768940200002,-2.223557482));
#149643=CARTESIAN_POINT('Ctrl Pts',(8.33632902867258,-1.32768940204799,
-2.39052074728083));
#149644=CARTESIAN_POINT('Ctrl Pts',(8.33295143111257,-1.33223595148368,
-2.3858053210651));
#149645=CARTESIAN_POINT('Ctrl Pts',(8.33003363689228,-1.33650155474458,
-2.38049770096133));
#149646=CARTESIAN_POINT('Ctrl Pts',(8.32339362671072,-1.34730670105808,
-2.36438073912203));
#149647=CARTESIAN_POINT('Ctrl Pts',(8.32086540459087,-1.35293307627555,
-2.3526803801806));
#149648=CARTESIAN_POINT('Ctrl Pts',(8.31984763173159,-1.35917045598987,
-2.33326255572515));
#149649=CARTESIAN_POINT('Ctrl Pts',(8.3200710828237,-1.3608789884345,-2.32612982083004));
#149650=CARTESIAN_POINT('Ctrl Pts',(8.32168988720682,-1.36317274229893,
-2.31177708459178));
#149651=CARTESIAN_POINT('Ctrl Pts',(8.32307844511106,-1.36375173586787,
-2.30460467131509));
#149652=CARTESIAN_POINT('Ctrl Pts',(8.32502258313608,-1.36375173586619,
-2.29756024539374));
#149653=CARTESIAN_POINT('Ctrl Pts',(8.32844213197043,-1.36375173586324,
-2.28516978847247));
#149654=CARTESIAN_POINT('Ctrl Pts',(8.33352455611133,-1.3619603189015,-2.27337615596146));
#149655=CARTESIAN_POINT('Ctrl Pts',(8.34649497791398,-1.3549908651978,-2.25218731932978));
#149656=CARTESIAN_POINT('Ctrl Pts',(8.3542709696827,-1.34985996711426,-2.24302553575725));
#149657=CARTESIAN_POINT('Ctrl Pts',(8.36910266521966,-1.33873894473671,
-2.23060703981489));
#149658=CARTESIAN_POINT('Ctrl Pts',(8.37567580732036,-1.33344492709784,
-2.2264888055179));
#149659=CARTESIAN_POINT('Ctrl Pts',(8.38240796207933,-1.32768940188415,
-2.2235574824097));
#149660=CARTESIAN_POINT('Ctrl Pts',(8.76147865594041,-1.00000000018314,
-2.05827397549611));
#149661=CARTESIAN_POINT('Ctrl Pts',(8.63672307032885,-1.10901473824796,
-2.11264514330979));
#149662=CARTESIAN_POINT('Ctrl Pts',(8.51030766293714,-1.21834403195478,
-2.16786723695558));
#149663=CARTESIAN_POINT('Ctrl Pts',(8.38240796203887,-1.32768940201087,
-2.22355748206797));
#149664=CARTESIAN_POINT('',(8.517054046,-1.32768940200002,-1.633634441));
#149665=CARTESIAN_POINT('Ctrl Pts',(8.51705404654846,-1.32768940205777,
-1.63363444058707));
#149666=CARTESIAN_POINT('Ctrl Pts',(8.60812476791986,-1.21834383457677,
-1.73930340900002));
#149667=CARTESIAN_POINT('Ctrl Pts',(8.69806104988347,-1.10901465435411,
-1.8439062745251));
#149668=CARTESIAN_POINT('Ctrl Pts',(8.78687111490328,-0.999999999901665,
-1.94702234497933));
#149669=CARTESIAN_POINT('',(8.547981008,-1.32768940200002,-1.463212837));
#149670=CARTESIAN_POINT('Ctrl Pts',(8.51705404632891,-1.32768940220838,
-1.6336344409322));
#149671=CARTESIAN_POINT('Ctrl Pts',(8.5132673585444,-1.33223595152413,-1.62924076322205));
#149672=CARTESIAN_POINT('Ctrl Pts',(8.50988553919814,-1.33650155467649,
-1.62421605920029));
#149673=CARTESIAN_POINT('Ctrl Pts',(8.50182754649101,-1.34730670090065,
-1.6087591855685));
#149674=CARTESIAN_POINT('Ctrl Pts',(8.49826069015919,-1.3529330761202,-1.59733255691655));
#149675=CARTESIAN_POINT('Ctrl Pts',(8.49550641418745,-1.35917045583786,
-1.57808413536979));
#149676=CARTESIAN_POINT('Ctrl Pts',(8.49508959230381,-1.36087898828368,
-1.57096008476704));
#149677=CARTESIAN_POINT('Ctrl Pts',(8.49541531049769,-1.36317274215052,
-1.55652001991912));
#149678=CARTESIAN_POINT('Ctrl Pts',(8.49615534830605,-1.36375173572067,
-1.54925201129861));
#149679=CARTESIAN_POINT('Ctrl Pts',(8.4974602023311,-1.36375173572018,-1.54206167297575));
#149680=CARTESIAN_POINT('Ctrl Pts',(8.49975531307054,-1.3637517357193,-1.52941457039706));
#149681=CARTESIAN_POINT('Ctrl Pts',(8.50376010379714,-1.36196031875968,
-1.51721283059529));
#149682=CARTESIAN_POINT('Ctrl Pts',(8.51477895782059,-1.35499086505998,
-1.49494663434248));
#149683=CARTESIAN_POINT('Ctrl Pts',(8.52170238978374,-1.34985996697839,
-1.48512469888792));
#149684=CARTESIAN_POINT('Ctrl Pts',(8.53536119188796,-1.33873894459695,
-1.4714266932106));
#149685=CARTESIAN_POINT('Ctrl Pts',(8.54153871678395,-1.33344492695049,
-1.46673582579239));
#149686=CARTESIAN_POINT('Ctrl Pts',(8.54798100809932,-1.32768940172794,
-1.46321283762611));
#149687=CARTESIAN_POINT('Ctrl Pts',(8.9107097751411,-1.00000000032794,-1.26461507871065));
#149688=CARTESIAN_POINT('Ctrl Pts',(8.79133021285898,-1.10901473827851,
-1.32995036863204));
#149689=CARTESIAN_POINT('Ctrl Pts',(8.6703737871565,-1.21834403187058,-1.39628194408301));
#149690=CARTESIAN_POINT('Ctrl Pts',(8.54798100805239,-1.32768940181178,
-1.46321283740333));
#149691=CARTESIAN_POINT('',(8.629204753,-1.32768940200002,-0.863595069999998));
#149692=CARTESIAN_POINT('Ctrl Pts',(8.6292047530183,-1.32768940220178,-0.863595070208368));
#149693=CARTESIAN_POINT('Ctrl Pts',(8.72938094365667,-1.21834383481036,
-0.960675129813628));
#149694=CARTESIAN_POINT('Ctrl Pts',(8.82833169708264,-1.10901465467741,
-1.05679506871452));
#149695=CARTESIAN_POINT('Ctrl Pts',(8.92602749210211,-1.00000000031437,
-1.15153515125643));
#149696=CARTESIAN_POINT('',(8.644730737,-1.32768940200002,-0.691087262999999));
#149697=CARTESIAN_POINT('Ctrl Pts',(8.62920475309882,-1.32768940213718,
-0.86359507005258));
#149698=CARTESIAN_POINT('Ctrl Pts',(8.62503946318526,-1.33223595143947,
-0.85955851608047));
#149699=CARTESIAN_POINT('Ctrl Pts',(8.62122084706452,-1.33650155457962,
-0.854857183999841));
#149700=CARTESIAN_POINT('Ctrl Pts',(8.6118097500053,-1.34730670079354,-0.840184848108705));
#149701=CARTESIAN_POINT('Ctrl Pts',(8.60723297769259,-1.35293307601313,
-0.829123950240993));
#149702=CARTESIAN_POINT('Ctrl Pts',(8.60276437442064,-1.3591704557308,-0.810199908575189));
#149703=CARTESIAN_POINT('Ctrl Pts',(8.60171063556652,-1.3608789881766,-0.803141900931394));
#149704=CARTESIAN_POINT('Ctrl Pts',(8.60074064508077,-1.36317274204343,
-0.788730770385562));
#149705=CARTESIAN_POINT('Ctrl Pts',(8.60082620444441,-1.36375173561358,
-0.781425684153338));
#149706=CARTESIAN_POINT('Ctrl Pts',(8.6014812685525,-1.36375173561308,-0.77414732580565));
#149707=CARTESIAN_POINT('Ctrl Pts',(8.60263346231566,-1.3637517356122,-0.761345404603284));
#149708=CARTESIAN_POINT('Ctrl Pts',(8.60552837540853,-1.36196031865258,
-0.748833798745698));
#149709=CARTESIAN_POINT('Ctrl Pts',(8.61450694432037,-1.35499086495292,
-0.72566951719315));
#149710=CARTESIAN_POINT('Ctrl Pts',(8.6205220730753,-1.34985996687135,-0.715266510306567));
#149711=CARTESIAN_POINT('Ctrl Pts',(8.63289800898064,-1.33873894459279,
-0.700399283329013));
#149712=CARTESIAN_POINT('Ctrl Pts',(8.63863017872564,-1.33344492707686,
-0.695173550994194));
#149713=CARTESIAN_POINT('Ctrl Pts',(8.64473073689484,-1.32768940200152,
-0.691087262840885));
#149714=CARTESIAN_POINT('Ctrl Pts',(8.98819709909128,-1.00000000022959,
-0.460774243805896));
#149715=CARTESIAN_POINT('Ctrl Pts',(8.87515473393588,-1.10901473830769,
-0.536547614610087));
#149716=CARTESIAN_POINT('Ctrl Pts',(8.76063115969153,-1.21834403202809,
-0.613454609141287));
#149717=CARTESIAN_POINT('Ctrl Pts',(8.64473073681857,-1.32768940209739,
-0.691087262591988));
#149718=CARTESIAN_POINT('Ctrl Pts',(8.67187817713732,-1.32768940195935,
-0.0866025397794751));
#149719=CARTESIAN_POINT('Ctrl Pts',(8.78035327729649,-1.21834383460799,
-0.174312059059673));
#149720=CARTESIAN_POINT('Ctrl Pts',(8.88752180893808,-1.10901465451525,
-0.261175170144172));
#149721=CARTESIAN_POINT('Ctrl Pts',(8.99331674489802,-1.00000000019189,
-0.346776473370393));
#149722=CARTESIAN_POINT('Origin',(1.11022302462516E-15,2.49999999999998,
2.22044604925031E-15));
#149723=CARTESIAN_POINT('',(-9.,1.75940739586291,2.77153710886662E-15));
#149724=CARTESIAN_POINT('',(-9.,2.49999999999998,3.32262816848293E-15));
#149725=CARTESIAN_POINT('',(-8.999583324,1.69247211199998,0.0866025400000026));
#149726=CARTESIAN_POINT('Ctrl Pts',(-9.,1.75940739586291,2.22044604925031E-15));
#149727=CARTESIAN_POINT('Ctrl Pts',(-9.,1.75940739586291,0.00982275238874841));
#149728=CARTESIAN_POINT('Ctrl Pts',(-8.99998359035555,1.75748289664218,
0.0195489494290313));
#149729=CARTESIAN_POINT('Ctrl Pts',(-8.99992093207107,1.74964163101758,
0.0390855278294033));
#149730=CARTESIAN_POINT('Ctrl Pts',(-8.999873350116,1.74349822247422,0.0484604739130678));
#149731=CARTESIAN_POINT('Ctrl Pts',(-8.9997556224668,1.7263063716269,0.0671302358527082));
#149732=CARTESIAN_POINT('Ctrl Pts',(-8.99968442188485,1.71456563907317,
0.0756568956210235));
#149733=CARTESIAN_POINT('Ctrl Pts',(-8.99960986283583,1.69868853660841,
0.0838135890526348));
#149734=CARTESIAN_POINT('Ctrl Pts',(-8.99959624897225,1.69560796569572,
0.0852593676028396));
#149735=CARTESIAN_POINT('Ctrl Pts',(-8.9995833236904,1.69247211204886,0.0866025401111445));
#149736=CARTESIAN_POINT('Ctrl Pts',(-8.99331674508598,1.00000000014682,
0.346776473475385));
#149737=CARTESIAN_POINT('Ctrl Pts',(-8.99381097525863,1.04120750313464,
0.333959085827753));
#149738=CARTESIAN_POINT('Ctrl Pts',(-8.99429823665098,1.08227801725674,
0.320609565855717));
#149739=CARTESIAN_POINT('Ctrl Pts',(-8.99697437540542,1.31475831842863,
0.242147345620229));
#149740=CARTESIAN_POINT('Ctrl Pts',(-8.99880589307605,1.50385659888367,
0.167391759544172));
#149741=CARTESIAN_POINT('Ctrl Pts',(-8.99958332369329,1.69247211191984,
0.0866025398099413));
#149742=CARTESIAN_POINT('',(-8.971116639,1.69247211199998,0.720462526000001));
#149743=CARTESIAN_POINT('Ctrl Pts',(-8.9711166389309,1.69247211219709,0.7204625255328));
#149744=CARTESIAN_POINT('Ctrl Pts',(-8.97758422784487,1.50385659904378,
0.639928851033998));
#149745=CARTESIAN_POINT('Ctrl Pts',(-8.98246112239683,1.31475831847271,
0.565310032927709));
#149746=CARTESIAN_POINT('Ctrl Pts',(-8.98682905618331,1.08227801719273,
0.486923791245082));
#149747=CARTESIAN_POINT('Ctrl Pts',(-8.98754039810537,1.0412075030817,0.473584334742427));
#149748=CARTESIAN_POINT('Ctrl Pts',(-8.98819709932765,1.000000000105,0.460774243678978));
#149749=CARTESIAN_POINT('',(-8.955590655,1.69247211199998,0.892970333000003));
#149750=CARTESIAN_POINT('Ctrl Pts',(-8.97111663891427,1.69247211210811,
0.720462525739921));
#149751=CARTESIAN_POINT('Ctrl Pts',(-8.97094631389628,1.6974393326074,0.722583393305224));
#149752=CARTESIAN_POINT('Ctrl Pts',(-8.97075555028734,1.70224131070956,
0.724949445788221));
#149753=CARTESIAN_POINT('Ctrl Pts',(-8.96991022372285,1.72064855663712,
0.735372056421202));
#149754=CARTESIAN_POINT('Ctrl Pts',(-8.96910800608783,1.73230722803945,
0.745137489624774));
#149755=CARTESIAN_POINT('Ctrl Pts',(-8.96754183055015,1.7468654653495,0.763706039604066));
#149756=CARTESIAN_POINT('Ctrl Pts',(-8.96684856957967,1.75155833642529,
0.771819838253853));
#149757=CARTESIAN_POINT('Ctrl Pts',(-8.96534621752964,1.75781013611547,
0.789074245141224));
#149758=CARTESIAN_POINT('Ctrl Pts',(-8.96457104154341,1.75940739573185,
0.797838434983111));
#149759=CARTESIAN_POINT('Ctrl Pts',(-8.96376864597118,1.75940739573272,
0.806753779975071));
#149760=CARTESIAN_POINT('Ctrl Pts',(-8.96288814123577,1.75940739573368,
0.816536988849674));
#149761=CARTESIAN_POINT('Ctrl Pts',(-8.96199994807101,1.7574828965141,0.826222560130248));
#149762=CARTESIAN_POINT('Ctrl Pts',(-8.96018629664472,1.74964163089218,
0.845674873362572));
#149763=CARTESIAN_POINT('Ctrl Pts',(-8.95929854255293,1.74349822235063,
0.855007813454931));
#149764=CARTESIAN_POINT('Ctrl Pts',(-8.95750774428347,1.72630637150765,
0.873591863395142));
#149765=CARTESIAN_POINT('Ctrl Pts',(-8.95667250644544,1.71456563895655,
0.882077814966626));
#149766=CARTESIAN_POINT('Ctrl Pts',(-8.95586708718875,1.69868853652541,
0.890194988511478));
#149767=CARTESIAN_POINT('Ctrl Pts',(-8.95572392954188,1.69560796564499,
0.891633726431578));
#149768=CARTESIAN_POINT('Ctrl Pts',(-8.95559065523919,1.69247211203143,
0.892970333097604));
#149769=CARTESIAN_POINT('Ctrl Pts',(-8.92602749238919,1.00000000013511,
1.1515351514879));
#149770=CARTESIAN_POINT('Ctrl Pts',(-8.92766867470473,1.04120750303497,
1.13881366534867));
#149771=CARTESIAN_POINT('Ctrl Pts',(-8.92935061626786,1.0822780170697,1.12556156441892));
#149772=CARTESIAN_POINT('Ctrl Pts',(-8.93904928087935,1.31475831830307,
1.04765509721038));
#149773=CARTESIAN_POINT('Ctrl Pts',(-8.94757446448273,1.50385659890226,
0.973364631047322));
#149774=CARTESIAN_POINT('Ctrl Pts',(-8.95559065522704,1.69247211208388,
0.892970333219481));
#149775=CARTESIAN_POINT('',(-8.870419798,1.69247211199998,1.521726851));
#149776=CARTESIAN_POINT('Ctrl Pts',(-8.87041979790224,1.69247211200266,
1.52172685097689));
#149777=CARTESIAN_POINT('Ctrl Pts',(-8.88408033312625,1.50385659891321,
1.44209713160695));
#149778=CARTESIAN_POINT('Ctrl Pts',(-8.89562637401809,1.31475831840579,
1.36821586841046));
#149779=CARTESIAN_POINT('Ctrl Pts',(-8.90700321231731,1.08227801720866,
1.2905367252853));
#149780=CARTESIAN_POINT('Ctrl Pts',(-8.90890743024755,1.04120750311532,
1.27731473371655));
#149781=CARTESIAN_POINT('Ctrl Pts',(-8.91070977549335,1.00000000015644,
1.26461507856234));
#149782=CARTESIAN_POINT('',(-8.83949283668534,1.69247211210181,1.69214845452143));
#149783=CARTESIAN_POINT('Ctrl Pts',(-8.87041979787082,1.69247211192305,
1.52172685116002));
#149784=CARTESIAN_POINT('Ctrl Pts',(-8.87006004542175,1.69743933254887,
1.52382391295804));
#149785=CARTESIAN_POINT('Ctrl Pts',(-8.86965795845286,1.70224131077037,
1.52616334054193));
#149786=CARTESIAN_POINT('Ctrl Pts',(-8.86788175929939,1.72064855680533,
1.53646821838201));
#149787=CARTESIAN_POINT('Ctrl Pts',(-8.86620740447287,1.73230722820551,
1.54612242858823));
#149788=CARTESIAN_POINT('Ctrl Pts',(-8.86298306190944,1.74686546551234,
1.56447583615115));
#149789=CARTESIAN_POINT('Ctrl Pts',(-8.86156527650011,1.7515583365868,1.57249482759808));
#149790=CARTESIAN_POINT('Ctrl Pts',(-8.85852229936856,1.75781013627524,
1.5895451035149));
#149791=CARTESIAN_POINT('Ctrl Pts',(-8.85696462809229,1.75940739589114,
1.59820452506459));
#149792=CARTESIAN_POINT('Ctrl Pts',(-8.8553662973649,1.75940739589201,1.60701205331319));
#149793=CARTESIAN_POINT('Ctrl Pts',(-8.85361237719985,1.75940739589296,
1.61667695002995));
#149794=CARTESIAN_POINT('Ctrl Pts',(-8.85185955172326,1.75748289667319,
1.62624391302741));
#149795=CARTESIAN_POINT('Ctrl Pts',(-8.84830950960882,1.74964163105064,
1.6454553425064));
#149796=CARTESIAN_POINT('Ctrl Pts',(-8.84658873105369,1.74349822250871,
1.65467113326302));
#149797=CARTESIAN_POINT('Ctrl Pts',(-8.84313928061765,1.72630637166508,
1.6730198433628));
#149798=CARTESIAN_POINT('Ctrl Pts',(-8.8415467303671,1.71456563911397,1.68139676284533));
#149799=CARTESIAN_POINT('Ctrl Pts',(-8.84001693566233,1.69868853665975,
1.68940906182158));
#149800=CARTESIAN_POINT('Ctrl Pts',(-8.83974538685126,1.69560796575533,
1.69082917526325));
#149801=CARTESIAN_POINT('Ctrl Pts',(-8.83949283657224,1.69247211211698,
1.69214845453584));
#149802=CARTESIAN_POINT('Ctrl Pts',(-8.78687111482176,0.999999999979337,
1.94702234489257));
#149803=CARTESIAN_POINT('Ctrl Pts',(-8.78964603545235,1.04120750300605,
1.93449918613234));
#149804=CARTESIAN_POINT('Ctrl Pts',(-8.79250911518946,1.08227801716676,
1.92145120230824));
#149805=CARTESIAN_POINT('Ctrl Pts',(-8.80915221770156,1.31475831840232,
1.84472774523967));
#149806=CARTESIAN_POINT('Ctrl Pts',(-8.82430242745039,1.5038565988819,1.77150054228567));
#149807=CARTESIAN_POINT('Ctrl Pts',(-8.8394928366488,1.69247211194256,1.6921484541359));
#149808=CARTESIAN_POINT('',(-8.698303553,1.69247211199998,2.310739126));
#149809=CARTESIAN_POINT('Ctrl Pts',(-8.69830355259779,1.69247211209572,
2.31073912566189));
#149810=CARTESIAN_POINT('Ctrl Pts',(-8.71904704750919,1.5038565991313,2.23265449314007));
#149811=CARTESIAN_POINT('Ctrl Pts',(-8.7371692727865,1.31475831874758,2.16010563338117));
#149812=CARTESIAN_POINT('Ctrl Pts',(-8.75546341597935,1.08227801752857,
2.08375901557486));
#149813=CARTESIAN_POINT('Ctrl Pts',(-8.75854517828406,1.04120750328463,
2.07076094459201));
#149814=CARTESIAN_POINT('Ctrl Pts',(-8.76147865613757,1.00000000017415,
2.05827397545756));
#149815=CARTESIAN_POINT('',(-8.652224619,1.69247211199998,2.477702391));
#149816=CARTESIAN_POINT('Ctrl Pts',(-8.69830355250322,1.69247211193793,
2.31073912601786));
#149817=CARTESIAN_POINT('Ctrl Pts',(-8.69775726913674,1.69743933262653,
2.31279549771896));
#149818=CARTESIAN_POINT('Ctrl Pts',(-8.69714709617372,1.70224131090743,
2.31508946468109));
#149819=CARTESIAN_POINT('Ctrl Pts',(-8.69445432534047,1.72064855700242,
2.3251936408784));
#149820=CARTESIAN_POINT('Ctrl Pts',(-8.69192131424338,1.73230722840749,
2.33465889806517));
#149821=CARTESIAN_POINT('Ctrl Pts',(-8.6870647651655,1.74686546571993,2.35264939236907));
#149822=CARTESIAN_POINT('Ctrl Pts',(-8.68493387049238,1.75155833679612,
2.36050901241014));
#149823=CARTESIAN_POINT('Ctrl Pts',(-8.6803747685432,1.75781013648825,2.37721787856242));
#149824=CARTESIAN_POINT('Ctrl Pts',(-8.67804714343072,1.75940739610623,
2.38570281125057));
#149825=CARTESIAN_POINT('Ctrl Pts',(-8.67566574636791,1.75940739610916,
2.3943316097188));
#149826=CARTESIAN_POINT('Ctrl Pts',(-8.6730525323078,1.75940739611239,2.40380037821234));
#149827=CARTESIAN_POINT('Ctrl Pts',(-8.67044918724009,1.75748289689478,
2.41317170536637));
#149828=CARTESIAN_POINT('Ctrl Pts',(-8.6651913372909,1.74964163127651,2.43198757195745));
#149829=CARTESIAN_POINT('Ctrl Pts',(-8.66265138897058,1.7434982227376,2.44101201324904));
#149830=CARTESIAN_POINT('Ctrl Pts',(-8.65757105931702,1.72630637190226,
2.45897765048096));
#149831=CARTESIAN_POINT('Ctrl Pts',(-8.65523401893332,1.71456563935741,
2.46717809184323));
#149832=CARTESIAN_POINT('Ctrl Pts',(-8.65299216577076,1.6986885367743,2.47502100598598));
#149833=CARTESIAN_POINT('Ctrl Pts',(-8.65259441213127,1.69560796572895,
2.47641106107899));
#149834=CARTESIAN_POINT('Ctrl Pts',(-8.65222461924908,1.6924721119451,2.47770239093806));
#149835=CARTESIAN_POINT('Ctrl Pts',(-8.57696801773418,1.00000000004553,
2.72683325906904));
#149836=CARTESIAN_POINT('Ctrl Pts',(-8.58085433463339,1.0412075029207,2.71460925687145));
#149837=CARTESIAN_POINT('Ctrl Pts',(-8.58487550069146,1.08227801693089,
2.70187044492656));
#149838=CARTESIAN_POINT('Ctrl Pts',(-8.60832904062519,1.31475831807767,
2.62694773016632));
#149839=CARTESIAN_POINT('Ctrl Pts',(-8.62998229595736,1.50385659861581,
2.55537337269809));
#149840=CARTESIAN_POINT('Ctrl Pts',(-8.65222461938352,1.69247211173591,
2.47770239046857));
#149841=CARTESIAN_POINT('',(-8.456153681,1.69247211199998,3.081146689));
#149842=CARTESIAN_POINT('Ctrl Pts',(-8.45615368104301,1.69247211178115,
3.0811466895594));
#149843=CARTESIAN_POINT('Ctrl Pts',(-8.48381312126247,1.50385659874206,
3.00523583532452));
#149844=CARTESIAN_POINT('Ctrl Pts',(-8.50836562146029,1.31475831828408,
2.93460349966487));
#149845=CARTESIAN_POINT('Ctrl Pts',(-8.53342977587719,1.08227801706105,
2.86020410525441));
#149846=CARTESIAN_POINT('Ctrl Pts',(-8.53766427000695,1.04120750289092,
2.84753460775047));
#149847=CARTESIAN_POINT('Ctrl Pts',(-8.54170526181922,0.999999999854698,
2.83536086243177));
#149848=CARTESIAN_POINT('',(-8.395293776,1.69247211199998,3.243307326));
#149849=CARTESIAN_POINT('Ctrl Pts',(-8.45615368110477,1.6924721118584,3.08114668938989));
#149850=CARTESIAN_POINT('Ctrl Pts',(-8.45542526516038,1.69743933268664,
3.08314581432305));
#149851=CARTESIAN_POINT('Ctrl Pts',(-8.45461191894058,1.70224131109879,
3.08537585102182));
#149852=CARTESIAN_POINT('Ctrl Pts',(-8.45102425701389,1.7206485572912,3.09519797272739));
#149853=CARTESIAN_POINT('Ctrl Pts',(-8.44765298396237,1.7323072286751,3.10439806820338));
#149854=CARTESIAN_POINT('Ctrl Pts',(-8.44120333044821,1.74686546595974,
3.12188080035488));
#149855=CARTESIAN_POINT('Ctrl Pts',(-8.43837648322229,1.75155833702593,
3.12951776794704));
#149856=CARTESIAN_POINT('Ctrl Pts',(-8.432337963664,1.75781013670153,3.14575069436043));
#149857=CARTESIAN_POINT('Ctrl Pts',(-8.42925912538441,1.75940739631255,
3.15399282249319));
#149858=CARTESIAN_POINT('Ctrl Pts',(-8.42611383559583,1.75940739631059,
3.16237341716321));
#149859=CARTESIAN_POINT('Ctrl Pts',(-8.42266236770178,1.75940739630844,
3.17156982047769));
#149860=CARTESIAN_POINT('Ctrl Pts',(-8.41922946364508,1.75748289708497,
3.18067005937171));
#149861=CARTESIAN_POINT('Ctrl Pts',(-8.41230613897276,1.74964163145378,
3.19893886878414));
#149862=CARTESIAN_POINT('Ctrl Pts',(-8.40896747105482,1.74349822290597,
3.20769930111942));
#149863=CARTESIAN_POINT('Ctrl Pts',(-8.4022971660049,1.72630637204837,3.22513721674514));
#149864=CARTESIAN_POINT('Ctrl Pts',(-8.39923445196042,1.71456563948876,
3.23309515485905));
#149865=CARTESIAN_POINT('Ctrl Pts',(-8.39629859042414,1.69868853682826,
3.24070553759573));
#149866=CARTESIAN_POINT('Ctrl Pts',(-8.39577783443639,1.69560796571781,
3.24205434239871));
#149867=CARTESIAN_POINT('Ctrl Pts',(-8.39529377630737,1.69247211186687,
3.24330732578562));
#149868=CARTESIAN_POINT('Ctrl Pts',(-8.29800821684455,0.999999999902031,
3.48468931659343));
#149869=CARTESIAN_POINT('Ctrl Pts',(-8.30297463971393,1.04120750304222,
3.47286289132727));
#149870=CARTESIAN_POINT('Ctrl Pts',(-8.30812151607148,1.08227801731563,
3.4605358165655));
#149871=CARTESIAN_POINT('Ctrl Pts',(-8.33819665933031,1.3147583184983,3.38801707773433));
#149872=CARTESIAN_POINT('Ctrl Pts',(-8.36617862092732,1.50385659881755,
3.31867184053366));
#149873=CARTESIAN_POINT('Ctrl Pts',(-8.39529377643312,1.6924721117174,3.24330732546012));
#149874=CARTESIAN_POINT('',(-8.145919833,1.69247211199998,3.82674667));
#149875=CARTESIAN_POINT('Ctrl Pts',(-8.14591983253155,1.69247211163032,
3.82674667073341));
#149876=CARTESIAN_POINT('Ctrl Pts',(-8.18027252047733,1.50385659864394,
3.75362078440848));
#149877=CARTESIAN_POINT('Ctrl Pts',(-8.21105761327326,1.3147583182386,3.68547366293637));
#149878=CARTESIAN_POINT('Ctrl Pts',(-8.24268997705341,1.08227801715203,
3.61362051213516));
#149879=CARTESIAN_POINT('Ctrl Pts',(-8.24804310934497,1.04120750306483,
3.6013815954542));
#149880=CARTESIAN_POINT('Ctrl Pts',(-8.2531590794202,1.00000000011213,3.58961908978988));
#149881=CARTESIAN_POINT('',(-8.070768965,1.69247211199998,3.982799055));
#149882=CARTESIAN_POINT('Ctrl Pts',(-8.14591983282591,1.69247211192685,
3.82674667010681));
#149883=CARTESIAN_POINT('Ctrl Pts',(-8.14501514910682,1.69743933265066,
3.8286724524188));
#149884=CARTESIAN_POINT('Ctrl Pts',(-8.14400517824978,1.70224131096443,
3.8308206038134));
#149885=CARTESIAN_POINT('Ctrl Pts',(-8.1395515110169,1.72064855707352,3.84028158896135));
#149886=CARTESIAN_POINT('Ctrl Pts',(-8.13536911951964,1.73230722846371,
3.84914244897217));
#149887=CARTESIAN_POINT('Ctrl Pts',(-8.12737829038704,1.74686546575702,
3.86597665830253));
#149888=CARTESIAN_POINT('Ctrl Pts',(-8.12387825071991,1.75155833682648,
3.87332948507808));
#149889=CARTESIAN_POINT('Ctrl Pts',(-8.11640893216073,1.75781013650711,
3.88895577378552));
#149890=CARTESIAN_POINT('Ctrl Pts',(-8.11260366970907,1.75940739611999,
3.89688873659974));
#149891=CARTESIAN_POINT('Ctrl Pts',(-8.10871981121782,1.75940739611904,
3.90495365185858));
#149892=CARTESIAN_POINT('Ctrl Pts',(-8.10445787868249,1.75940739611799,
3.9138036459595));
#149893=CARTESIAN_POINT('Ctrl Pts',(-8.10022305536408,1.75748289689589,
3.92255952681936));
#149894=CARTESIAN_POINT('Ctrl Pts',(-8.09168999851364,1.74964163126793,
3.94013418933557));
#149895=CARTESIAN_POINT('Ctrl Pts',(-8.08757949199218,1.7434982227223,3.94856007886009));
#149896=CARTESIAN_POINT('Ctrl Pts',(-8.07937291692608,1.72630637186984,
3.96532987302821));
#149897=CARTESIAN_POINT('Ctrl Pts',(-8.0756091883959,1.71456563931326,3.97298123525238));
#149898=CARTESIAN_POINT('Ctrl Pts',(-8.07200295636026,1.69868853680513,
3.98029781215842));
#149899=CARTESIAN_POINT('Ctrl Pts',(-8.07136339088196,1.69560796585033,
3.98159450680377));
#149900=CARTESIAN_POINT('Ctrl Pts',(-8.07076896488867,1.69247211216003,
3.98279905536168));
#149901=CARTESIAN_POINT('Ctrl Pts',(-7.95223773338532,1.0000000000746,4.2144887034755));
#149902=CARTESIAN_POINT('Ctrl Pts',(-7.95824427546704,1.04120750308548,
4.20315507466545));
#149903=CARTESIAN_POINT('Ctrl Pts',(-7.96447542245755,1.08227801723047,
4.19133898755649));
#149904=CARTESIAN_POINT('Ctrl Pts',(-8.00093002168167,1.31475831851661,
4.12180810286586));
#149905=CARTESIAN_POINT('Ctrl Pts',(-8.03501539531451,1.50385659906093,
4.05525031280323));
#149906=CARTESIAN_POINT('Ctrl Pts',(-8.07076896486063,1.69247211218716,
3.9827990554185));
#149907=CARTESIAN_POINT('',(-7.770099827,1.69247211199998,4.541535938));
#149908=CARTESIAN_POINT('Ctrl Pts',(-7.77009982692731,1.69247211184426,
4.54153593837858));
#149909=CARTESIAN_POINT('Ctrl Pts',(-7.81086917503205,1.50385659862522,
4.47178378647429));
#149910=CARTESIAN_POINT('Ctrl Pts',(-7.84763899702609,1.31475831798858,
4.40667055962397));
#149911=CARTESIAN_POINT('Ctrl Pts',(-7.88558488501719,1.08227801676248,
4.33794217166716));
#149912=CARTESIAN_POINT('Ctrl Pts',(-7.89201355519076,1.04120750277453,
4.32623237637253));
#149913=CARTESIAN_POINT('Ctrl Pts',(-7.89816331274033,0.999999999921736,
4.31497581514458));
#149914=CARTESIAN_POINT('',(-7.681263067,1.69247211199998,4.69022363));
#149915=CARTESIAN_POINT('Ctrl Pts',(-7.77009982710407,1.69247211199432,
4.54153593807615));
#149916=CARTESIAN_POINT('Ctrl Pts',(-7.76902615958796,1.69743933266121,
4.54337287251751));
#149917=CARTESIAN_POINT('Ctrl Pts',(-7.7678276957807,1.70224131092097,4.54542184297812));
#149918=CARTESIAN_POINT('Ctrl Pts',(-7.76254388154537,1.72064855696673,
4.55444551730453));
#149919=CARTESIAN_POINT('Ctrl Pts',(-7.75758404575988,1.73230722834443,
4.56289579941125));
#149920=CARTESIAN_POINT('Ctrl Pts',(-7.74811637846733,1.74686546562209,
4.57894594675684));
#149921=CARTESIAN_POINT('Ctrl Pts',(-7.74397132662034,1.75155833668633,
4.58595543207489));
#149922=CARTESIAN_POINT('Ctrl Pts',(-7.73513134762144,1.7578101363574,4.60084926938084));
#149923=CARTESIAN_POINT('Ctrl Pts',(-7.73063029873371,1.75940739596569,
4.60840919532058));
#149924=CARTESIAN_POINT('Ctrl Pts',(-7.72603914208534,1.75940739596087,
4.61609349720791));
#149925=CARTESIAN_POINT('Ctrl Pts',(-7.72100105948176,1.75940739595559,
4.62452582714662));
#149926=CARTESIAN_POINT('Ctrl Pts',(-7.71599841320754,1.75748289672923,
4.63286685276749));
#149927=CARTESIAN_POINT('Ctrl Pts',(-7.70592432733087,1.7496416310923,4.6496058675405));
#149928=CARTESIAN_POINT('Ctrl Pts',(-7.70107507758455,1.74349822254042,
4.65762937394832));
#149929=CARTESIAN_POINT('Ctrl Pts',(-7.69139830701293,1.7263063716716,4.67359602614167));
#149930=CARTESIAN_POINT('Ctrl Pts',(-7.68696386732324,1.71456563910337,
4.68087920820852));
#149931=CARTESIAN_POINT('Ctrl Pts',(-7.68271630004147,1.6986885366654,4.68784307054307));
#149932=CARTESIAN_POINT('Ctrl Pts',(-7.68196307447331,1.69560796579605,
4.68907721483747));
#149933=CARTESIAN_POINT('Ctrl Pts',(-7.68126306658054,1.692472112194,4.69022363027454));
#149934=CARTESIAN_POINT('Ctrl Pts',(-7.54244050719113,0.999999999972252,
4.91035550601812));
#149935=CARTESIAN_POINT('Ctrl Pts',(-7.54943880738768,1.0412075031992,4.89960592529647));
#149936=CARTESIAN_POINT('Ctrl Pts',(-7.55670405553103,1.08227801755879,
4.88839596193518));
#149937=CARTESIAN_POINT('Ctrl Pts',(-7.59924459970585,1.31475831885198,
4.82241275323143));
#149938=CARTESIAN_POINT('Ctrl Pts',(-7.63915894989652,1.50385659919618,
4.75917829468802));
#149939=CARTESIAN_POINT('Ctrl Pts',(-7.6812630666695,1.69247211212086,4.69022363012885));
#149940=CARTESIAN_POINT('',(-7.331719547,1.69247211199998,5.219759428));
#149941=CARTESIAN_POINT('Ctrl Pts',(-7.33171954715669,1.69247211218445,
5.2197594275829));
#149942=CARTESIAN_POINT('Ctrl Pts',(-7.37857730449581,1.5038565990772,5.15394261357347));
#149943=CARTESIAN_POINT('Ctrl Pts',(-7.42103580661076,1.31475831855127,
5.09238753490903));
#149944=CARTESIAN_POINT('Ctrl Pts',(-7.46498970082048,1.08227801722486,
5.0273372703834));
#149945=CARTESIAN_POINT('Ctrl Pts',(-7.47244214905171,1.04120750302034,
5.01625087677696));
#149946=CARTESIAN_POINT('Ctrl Pts',(-7.47957617988741,0.999999999949514,
5.00559089111974));
#149947=CARTESIAN_POINT('',(-7.229912155,1.69247211199998,5.359885281));
#149948=CARTESIAN_POINT('Ctrl Pts',(-7.33171954712374,1.69247211216016,
5.21975942762917));
#149949=CARTESIAN_POINT('Ctrl Pts',(-7.33048554037461,1.69743933266442,
5.22149272425506));
#149950=CARTESIAN_POINT('Ctrl Pts',(-7.32910823297432,1.7022413107712,5.22342601663964));
#149951=CARTESIAN_POINT('Ctrl Pts',(-7.32303681394078,1.72064855669881,
5.23193972678211));
#149952=CARTESIAN_POINT('Ctrl Pts',(-7.31733946754655,1.73230722809749,
5.23991139428892));
#149953=CARTESIAN_POINT('Ctrl Pts',(-7.30647119017968,1.74686546540271,
5.25504825331498));
#149954=CARTESIAN_POINT('Ctrl Pts',(-7.30171449967183,1.75155833647675,
5.26165796092615));
#149955=CARTESIAN_POINT('Ctrl Pts',(-7.29157503454324,1.75781013616407,
5.27569943042096));
#149956=CARTESIAN_POINT('Ctrl Pts',(-7.2864144390166,1.75940739577924,5.2828254514138));
#149957=CARTESIAN_POINT('Ctrl Pts',(-7.28115294950206,1.7594073957793,5.29006727045672));
#149958=CARTESIAN_POINT('Ctrl Pts',(-7.27537928051152,1.75940739577936,
5.29801404407048));
#149959=CARTESIAN_POINT('Ctrl Pts',(-7.26964908964959,1.75748289655881,
5.30587305741947));
#149960=CARTESIAN_POINT('Ctrl Pts',(-7.25811508536945,1.74964163093469,
5.32164165174141));
#149961=CARTESIAN_POINT('Ctrl Pts',(-7.25256613571054,1.74349822239162,
5.32919817447285));
#149962=CARTESIAN_POINT('Ctrl Pts',(-7.24149708131024,1.72630637154491,
5.344233130587));
#149963=CARTESIAN_POINT('Ctrl Pts',(-7.23642763396645,1.71456563899138,
5.35108949259295));
#149964=CARTESIAN_POINT('Ctrl Pts',(-7.23157293031562,1.69868853650539,
5.3576445714967));
#149965=CARTESIAN_POINT('Ctrl Pts',(-7.23071210915307,1.69560796557039,
5.3588062288934));
#149966=CARTESIAN_POINT('Ctrl Pts',(-7.2299121553839,1.69247211190049,5.3598852809955));
#149967=CARTESIAN_POINT('Ctrl Pts',(-7.07191598531854,0.999999999848428,
5.56668701263113));
#149968=CARTESIAN_POINT('Ctrl Pts',(-7.0798496973723,1.04120750290071,5.55660802939234));
#149969=CARTESIAN_POINT('Ctrl Pts',(-7.08809055109799,1.08227801708678,
5.54609444591211));
#149970=CARTESIAN_POINT('Ctrl Pts',(-7.13637452878035,1.31475831838269,
5.48419017118036));
#149971=CARTESIAN_POINT('Ctrl Pts',(-7.18179648874699,1.50385659889642,
5.42478817067091));
#149972=CARTESIAN_POINT('Ctrl Pts',(-7.22991215525667,1.69247211199201,
5.35988528116712));
#149973=CARTESIAN_POINT('',(-6.834308572,1.69247211199998,5.855956484));
#149974=CARTESIAN_POINT('Ctrl Pts',(-6.83430857185789,1.69247211190127,
5.85595648418171));
#149975=CARTESIAN_POINT('Ctrl Pts',(-6.88687746734898,1.50385659885685,
5.79460492632121));
#149976=CARTESIAN_POINT('Ctrl Pts',(-6.93468279871554,1.31475831839393,
5.73710360111202));
#149977=CARTESIAN_POINT('Ctrl Pts',(-6.98429080820646,1.08227801718584,
5.67625520655512));
#149978=CARTESIAN_POINT('Ctrl Pts',(-6.99270703172362,1.04120750303555,
5.66588147583171));
#149979=CARTESIAN_POINT('Ctrl Pts',(-7.0007678967871,1.00000000001932,5.65590389374812));
#149980=CARTESIAN_POINT('',(-6.720350242,1.69247211199998,5.986392288));
#149981=CARTESIAN_POINT('Ctrl Pts',(-6.83430857189648,1.69247211192666,
5.85595648413667));
#149982=CARTESIAN_POINT('Ctrl Pts',(-6.83292416134052,1.69743933264486,
5.85757218755852));
#149983=CARTESIAN_POINT('Ctrl Pts',(-6.83137909952495,1.70224131095344,
5.85937423625886));
#149984=CARTESIAN_POINT('Ctrl Pts',(-6.8245689590756,1.72064855706262,5.86730943498249));
#149985=CARTESIAN_POINT('Ctrl Pts',(-6.81817997375611,1.73230722845714,
5.87473830470638));
#149986=CARTESIAN_POINT('Ctrl Pts',(-6.80599859129646,1.74686546575595,
5.88884000231499));
#149987=CARTESIAN_POINT('Ctrl Pts',(-6.80066856020434,1.75155833682738,
5.89499671473559));
#149988=CARTESIAN_POINT('Ctrl Pts',(-6.78931124596147,1.75781013651137,
5.90807276275261));
#149989=CARTESIAN_POINT('Ctrl Pts',(-6.78353265387896,1.75940739612577,
5.91470750426196));
#149990=CARTESIAN_POINT('Ctrl Pts',(-6.77764319392101,1.75940739612599,
5.92144853358502));
#149991=CARTESIAN_POINT('Ctrl Pts',(-6.77118042472805,1.75940739612624,
5.92884576812757));
#149992=CARTESIAN_POINT('Ctrl Pts',(-6.76476882540304,1.75748289690549,
5.93615949305174));
#149993=CARTESIAN_POINT('Ctrl Pts',(-6.75186776773317,1.74964163128042,
5.95083070747797));
#149994=CARTESIAN_POINT('Ctrl Pts',(-6.74566379503781,1.7434982227368,5.95785940585847));
#149995=CARTESIAN_POINT('Ctrl Pts',(-6.73329157831984,1.72630637188949,
5.97184161327271));
#149996=CARTESIAN_POINT('Ctrl Pts',(-6.72762793952884,1.71456563933646,
5.97821595182398));
#149997=CARTESIAN_POINT('Ctrl Pts',(-6.72220518672269,1.69868853678518,
5.98430946965148));
#149998=CARTESIAN_POINT('Ctrl Pts',(-6.72124370078741,1.69560796578166,
5.98538928716463));
#149999=CARTESIAN_POINT('Ctrl Pts',(-6.72035024189579,1.69247211204104,
5.98639228803552));
#150000=CARTESIAN_POINT('Ctrl Pts',(-6.54445255413051,0.999999999900246,
6.17819882868257));
#150001=CARTESIAN_POINT('Ctrl Pts',(-6.553257800479,1.04120750293032,6.16887159293748));
#150002=CARTESIAN_POINT('Ctrl Pts',(-6.56240790930224,1.08227801709433,
6.15913903849141));
#150003=CARTESIAN_POINT('Ctrl Pts',(-6.6160465662733,1.31475831833009,6.1018121145769));
#150004=CARTESIAN_POINT('Ctrl Pts',(-6.66661042504181,1.5038565988065,6.04672084217141));
#150005=CARTESIAN_POINT('Ctrl Pts',(-6.72035024216997,1.69247211186447,
5.98639228772773));
#150006=CARTESIAN_POINT('',(-6.281871763,1.69247211199998,6.445004822));
#150007=CARTESIAN_POINT('Ctrl Pts',(-6.28187176315731,1.69247211214928,
6.44500482166204));
#150008=CARTESIAN_POINT('Ctrl Pts',(-6.33972854297823,1.50385659908023,
6.38861248658687));
#150009=CARTESIAN_POINT('Ctrl Pts',(-6.39249580318892,1.31475831859254,
6.33562788166308));
#150010=CARTESIAN_POINT('Ctrl Pts',(-6.44735851345535,1.08227801735199,
6.27947127252895));
#150011=CARTESIAN_POINT('Ctrl Pts',(-6.45667074978434,1.04120750319416,
6.26989372785291));
#150012=CARTESIAN_POINT('Ctrl Pts',(-6.46559354773797,1.00000000017037,
6.26067888295264));
#150013=CARTESIAN_POINT('',(-6.15668002,1.69247211199998,6.564700384));
#150014=CARTESIAN_POINT('Ctrl Pts',(-6.28187176296278,1.69247211203293,
6.44500482185164));
#150015=CARTESIAN_POINT('Ctrl Pts',(-6.28034809508384,1.6974393328171,6.44648992333557));
#150016=CARTESIAN_POINT('Ctrl Pts',(-6.27864771881356,1.70224131118792,
6.44814621926317));
#150017=CARTESIAN_POINT('Ctrl Pts',(-6.27115368823422,1.7206485573528,6.4554390169499));
#150018=CARTESIAN_POINT('Ctrl Pts',(-6.26412450434296,1.73230722874671,
6.46226527600062));
#150019=CARTESIAN_POINT('Ctrl Pts',(-6.25072809411952,1.74686546604397,
6.47521827361669));
#150020=CARTESIAN_POINT('Ctrl Pts',(-6.24486763671978,1.75155833711437,
6.4808724206194));
#150021=CARTESIAN_POINT('Ctrl Pts',(-6.23238391577944,1.7578101367976,6.49287776651093));
#150022=CARTESIAN_POINT('Ctrl Pts',(-6.22603385296701,1.75940739641221,
6.4989678095005));
#150023=CARTESIAN_POINT('Ctrl Pts',(-6.21956384103444,1.75940739641324,
6.50515377430057));
#150024=CARTESIAN_POINT('Ctrl Pts',(-6.21246400605726,1.75940739641437,
6.51194191158887));
#150025=CARTESIAN_POINT('Ctrl Pts',(-6.20542262069756,1.75748289719422,
6.51865146227563));
#150026=CARTESIAN_POINT('Ctrl Pts',(-6.19125838137018,1.74964163157005,
6.53210717281416));
#150027=CARTESIAN_POINT('Ctrl Pts',(-6.18444933637955,1.74349822302714,
6.53855145589715));
#150028=CARTESIAN_POINT('Ctrl Pts',(-6.17087357116009,1.72630637218225,
6.55136833809903));
#150029=CARTESIAN_POINT('Ctrl Pts',(-6.16466134121213,1.71456563963167,
6.55720933076995));
#150030=CARTESIAN_POINT('Ctrl Pts',(-6.15871420003383,1.69868853693743,
6.56279222612325));
#150031=CARTESIAN_POINT('Ctrl Pts',(-6.15765979061543,1.69560796578235,
6.56378150971813));
#150032=CARTESIAN_POINT('Ctrl Pts',(-6.15668002018172,1.69247211188529,
6.56470038380239));
#150033=CARTESIAN_POINT('Ctrl Pts',(-5.96429703930701,0.999999999993485,
6.73996742031544));
#150034=CARTESIAN_POINT('Ctrl Pts',(-5.97390292527018,1.0412075029378,6.73146702949199));
#150035=CARTESIAN_POINT('Ctrl Pts',(-5.98388861787978,1.08227801701665,
6.72259386489691));
#150036=CARTESIAN_POINT('Ctrl Pts',(-6.04245008719923,1.31475831813608,
6.67030585448667));
#150037=CARTESIAN_POINT('Ctrl Pts',(-6.09774873431316,1.50385659858127,
6.61996887270678));
#150038=CARTESIAN_POINT('Ctrl Pts',(-6.15668002065362,1.69247211160818,
6.56470038335982));
#150039=CARTESIAN_POINT('',(-5.678857015,1.69247211199998,6.982161771));
#150040=CARTESIAN_POINT('Ctrl Pts',(-5.67885701527804,1.69247211202244,
6.98216177125877));
#150041=CARTESIAN_POINT('Ctrl Pts',(-5.74153585071579,1.50385659882619,
6.93118269686947));
#150042=CARTESIAN_POINT('Ctrl Pts',(-5.79884018886956,1.31475831821191,
6.88314141309412));
#150043=CARTESIAN_POINT('Ctrl Pts',(-5.85851587764468,1.08227801691581,
6.83212872938778));
#150044=CARTESIAN_POINT('Ctrl Pts',(-5.86864915011615,1.04120750283384,
6.82342448353686));
#150045=CARTESIAN_POINT('Ctrl Pts',(-5.87836203982082,0.999999999886375,
6.81504656835106));
#150046=CARTESIAN_POINT('',(-5.54343983025804,1.69247211212479,7.09015337246985));
#150047=CARTESIAN_POINT('Ctrl Pts',(-5.678857014964,1.69247211184902,6.98216177151419));
#150048=CARTESIAN_POINT('Ctrl Pts',(-5.67720635746448,1.69743933258059,
6.98350431387102));
#150049=CARTESIAN_POINT('Ctrl Pts',(-5.67536435720179,1.70224131090145,
6.98500152147185));
#150050=CARTESIAN_POINT('Ctrl Pts',(-5.66724677406058,1.72064855700654,
6.99159320075996));
#150051=CARTESIAN_POINT('Ctrl Pts',(-5.65963398645598,1.73230722838665,
6.99776188810862));
#150052=CARTESIAN_POINT('Ctrl Pts',(-5.64513040849174,1.74686546566723,
7.00946189580316));
#150053=CARTESIAN_POINT('Ctrl Pts',(-5.63878670974102,1.75155833673249,
7.01456795351953));
#150054=CARTESIAN_POINT('Ctrl Pts',(-5.62527709368239,1.75781013640549,
7.02540593729718));
#150055=CARTESIAN_POINT('Ctrl Pts',(-5.61840668711161,1.75940739601474,
7.03090224832023));
#150056=CARTESIAN_POINT('Ctrl Pts',(-5.61140821593638,1.75940739601077,
7.03648334284404));
#150057=CARTESIAN_POINT('Ctrl Pts',(-5.60372847887256,1.75940739600641,
7.04260772878464));
#150058=CARTESIAN_POINT('Ctrl Pts',(-5.5961140005745,1.75748289678097,7.04865908387313));
#150059=CARTESIAN_POINT('Ctrl Pts',(-5.58080062171541,1.74964163114594,
7.06079095305035));
#150060=CARTESIAN_POINT('Ctrl Pts',(-5.57344132685396,1.7434982225954,7.06659893525709));
#150061=CARTESIAN_POINT('Ctrl Pts',(-5.55877131720445,1.7263063717301,7.0781472982493));
#150062=CARTESIAN_POINT('Ctrl Pts',(-5.55206051331798,1.71456563916442,
7.08340791680299));
#150063=CARTESIAN_POINT('Ctrl Pts',(-5.54563686680511,1.69868853671578,
7.08843523935246));
#150064=CARTESIAN_POINT('Ctrl Pts',(-5.54449802352356,1.69560796583262,
7.08932602377848));
#150065=CARTESIAN_POINT('Ctrl Pts',(-5.54343983019798,1.69247211221631,
7.09015337273988));
#150066=CARTESIAN_POINT('Ctrl Pts',(-5.33612051021732,1.00000000003863,
7.24746975850456));
#150067=CARTESIAN_POINT('Ctrl Pts',(-5.34644969490053,1.04120750312078,
7.23986465271198));
#150068=CARTESIAN_POINT('Ctrl Pts',(-5.35719057242631,1.08227801733654,
7.23192231942854));
#150069=CARTESIAN_POINT('Ctrl Pts',(-5.42020335165464,1.3147583185972,7.18509421478981));
#150070=CARTESIAN_POINT('Ctrl Pts',(-5.47979155494116,1.50385659904842,
7.13991680741592));
#150071=CARTESIAN_POINT('Ctrl Pts',(-5.54343983044598,1.69247211208145,
7.09015337254597));
#150072=CARTESIAN_POINT('',(-5.030119452,1.69247211199998,7.463102458));
#150073=CARTESIAN_POINT('Ctrl Pts',(-5.03011945219446,1.69247211210034,
7.46310245786931));
#150074=CARTESIAN_POINT('Ctrl Pts',(-5.09711568993067,1.50385659918751,
7.41794709780784));
#150075=CARTESIAN_POINT('Ctrl Pts',(-5.15849572502523,1.31475831885526,
7.3752359354521));
#150076=CARTESIAN_POINT('Ctrl Pts',(-5.22250391870522,1.08227801764803,
7.3297779013181));
#150077=CARTESIAN_POINT('Ctrl Pts',(-5.23337664023476,1.04120750336251,
7.32201703570376));
#150078=CARTESIAN_POINT('Ctrl Pts',(-5.24380141927541,1.00000000021015,
7.31454350422535));
#150079=CARTESIAN_POINT('',(-4.885567124,1.69247211199998,7.558520614));
#150080=CARTESIAN_POINT('Ctrl Pts',(-5.03011945218954,1.69247211209782,
7.46310245787263));
#150081=CARTESIAN_POINT('Ctrl Pts',(-5.02835509520953,1.69743933274048,
7.46429163173374));
#150082=CARTESIAN_POINT('Ctrl Pts',(-5.0263863016777,1.70224131097822,7.46561769636424));
#150083=CARTESIAN_POINT('Ctrl Pts',(-5.01771052400477,1.72064855704174,
7.47145518492245));
#150084=CARTESIAN_POINT('Ctrl Pts',(-5.00957542636928,1.73230722845448,
7.4769166339361));
#150085=CARTESIAN_POINT('Ctrl Pts',(-4.99408145493217,1.74686546577658,
7.4872694501465));
#150086=CARTESIAN_POINT('Ctrl Pts',(-4.98730559056024,1.75155833685606,
7.49178630760795));
#150087=CARTESIAN_POINT('Ctrl Pts',(-4.97287885086278,1.75781013655407,
7.50136966821127));
#150088=CARTESIAN_POINT('Ctrl Pts',(-4.96554341700394,1.7594073961748,7.50622799421013));
#150089=CARTESIAN_POINT('Ctrl Pts',(-4.95807283415526,1.75940739618001,
7.51115928277464));
#150090=CARTESIAN_POINT('Ctrl Pts',(-4.94987502773368,1.75940739618573,
7.51657060741686));
#150091=CARTESIAN_POINT('Ctrl Pts',(-4.94174876379914,1.75748289697065,
7.52191504495915));
#150092=CARTESIAN_POINT('Ctrl Pts',(-4.92540953973939,1.74964163135777,
7.53262539410137));
#150093=CARTESIAN_POINT('Ctrl Pts',(-4.91755924773008,1.74349822282263,
7.53775031297301));
#150094=CARTESIAN_POINT('Ctrl Pts',(-4.90191310796274,1.72630637199696,
7.54793717612114));
#150095=CARTESIAN_POINT('Ctrl Pts',(-4.89475776159462,1.71456563945895,
7.55257506514706));
#150096=CARTESIAN_POINT('Ctrl Pts',(-4.88790932897337,1.69868853680129,
7.55700633800827));
#150097=CARTESIAN_POINT('Ctrl Pts',(-4.88669522094921,1.69560796567097,
7.55779145133232));
#150098=CARTESIAN_POINT('Ctrl Pts',(-4.88556712453283,1.69247211179938,
7.55852061396171));
#150099=CARTESIAN_POINT('Ctrl Pts',(-4.66498067898464,0.999999999967121,
7.69661972977099));
#150100=CARTESIAN_POINT('Ctrl Pts',(-4.67594999777918,1.04120750284047,
7.68997114090538));
#150101=CARTESIAN_POINT('Ctrl Pts',(-4.6873595808967,1.08227801684883,7.68302358599243));
#150102=CARTESIAN_POINT('Ctrl Pts',(-4.75431632809316,1.31475831803052,
7.6420324195285));
#150103=CARTESIAN_POINT('Ctrl Pts',(-4.81771431840041,1.50385659860426,
7.60237832843866));
#150104=CARTESIAN_POINT('Ctrl Pts',(-4.88556712461049,1.69247211175979,
7.55852061391151));
#150105=CARTESIAN_POINT('',(-4.340882323,1.69247211199998,7.883954633));
#150106=CARTESIAN_POINT('Ctrl Pts',(-4.34088232282825,1.69247211188109,
7.88395463326351));
#150107=CARTESIAN_POINT('Ctrl Pts',(-4.41165654866182,1.50385659901075,
7.84498655187241));
#150108=CARTESIAN_POINT('Ctrl Pts',(-4.47661808484275,1.31475831872082,
7.80794939604147));
#150109=CARTESIAN_POINT('Ctrl Pts',(-4.54444342707815,1.08227801765357,
7.76841201286517));
#150110=CARTESIAN_POINT('Ctrl Pts',(-4.55596805683155,1.04120750346539,
7.76165701347468));
#150111=CARTESIAN_POINT('Ctrl Pts',(-4.56702079094976,1.00000000041108,
7.75514803824096));
#150112=CARTESIAN_POINT('',(-4.188358703,1.69247211199998,7.966031093));
#150113=CARTESIAN_POINT('Ctrl Pts',(-4.34088232285577,1.69247211189453,
7.88395463324836));
#150114=CARTESIAN_POINT('Ctrl Pts',(-4.33901847194055,1.69743933251756,
7.88498086410162));
#150115=CARTESIAN_POINT('Ctrl Pts',(-4.33693873668265,1.70224131073674,
7.88612510909012));
#150116=CARTESIAN_POINT('Ctrl Pts',(-4.32777461670888,1.72064855678309,
7.89116140691491));
#150117=CARTESIAN_POINT('Ctrl Pts',(-4.3191827080702,1.73230722819562,7.89587164520933));
#150118=CARTESIAN_POINT('Ctrl Pts',(-4.30282309151686,1.74686546551824,
7.90479391513174));
#150119=CARTESIAN_POINT('Ctrl Pts',(-4.29566961680086,1.7515583365982,7.9086852052531));
#150120=CARTESIAN_POINT('Ctrl Pts',(-4.28044190909274,1.75781013629619,
7.91693678308731));
#150121=CARTESIAN_POINT('Ctrl Pts',(-4.27270050854822,1.75940739591639,
7.92111800767207));
#150122=CARTESIAN_POINT('Ctrl Pts',(-4.26481796277002,1.75940739592062,
7.92535978643457));
#150123=CARTESIAN_POINT('Ctrl Pts',(-4.25616809090657,1.75940739592527,
7.93001448097122));
#150124=CARTESIAN_POINT('Ctrl Pts',(-4.24759546923469,1.75748289670936,
7.93460897069478));
#150125=CARTESIAN_POINT('Ctrl Pts',(-4.23036195379282,1.74964163109505,
7.94381156636528));
#150126=CARTESIAN_POINT('Ctrl Pts',(-4.22208387056523,1.74349822255881,
7.94821215906904));
#150127=CARTESIAN_POINT('Ctrl Pts',(-4.20558757418278,1.72630637172989,
7.95695550374437));
#150128=CARTESIAN_POINT('Ctrl Pts',(-4.19804529596738,1.71456563918893,
7.96093332168898));
#150129=CARTESIAN_POINT('Ctrl Pts',(-4.19082721695447,1.69868853668133,
7.96473286674421));
#150130=CARTESIAN_POINT('Ctrl Pts',(-4.18954761961682,1.69560796571051,
7.96540598759677));
#150131=CARTESIAN_POINT('Ctrl Pts',(-4.18835870300193,1.69247211200357,
7.96603109302167));
#150132=CARTESIAN_POINT('Ctrl Pts',(-3.95628116469446,1.00000000003948,
8.08380104566434));
#150133=CARTESIAN_POINT('Ctrl Pts',(-3.96780229915045,1.04120750292555,
8.07816250421748));
#150134=CARTESIAN_POINT('Ctrl Pts',(-3.97978872466481,1.08227801694657,
8.07226566526221));
#150135=CARTESIAN_POINT('Ctrl Pts',(-4.05015034350906,1.31475831811704,
8.03744147373218));
#150136=CARTESIAN_POINT('Ctrl Pts',(-4.11684767745441,1.50385659866781,
8.00362997039905));
#150137=CARTESIAN_POINT('Ctrl Pts',(-4.18835870342248,1.69247211180005,
7.96603109280055));
#150138=CARTESIAN_POINT('',(-3.61669496163465,1.69247211178013,8.24132984144472));
#150139=CARTESIAN_POINT('Ctrl Pts',(-3.61669496156912,1.69247211175992,
8.24132984141277));
#150140=CARTESIAN_POINT('Ctrl Pts',(-3.69067734322808,1.5038565985687,8.20886278668499));
#150141=CARTESIAN_POINT('Ctrl Pts',(-3.75869734856277,1.3147583179601,8.17779783869765));
#150142=CARTESIAN_POINT('Ctrl Pts',(-3.82979374964924,1.08227801680555,
8.14449943819061));
#150143=CARTESIAN_POINT('Ctrl Pts',(-3.84187749804066,1.04120750286064,
8.13880469232044));
#150144=CARTESIAN_POINT('Ctrl Pts',(-3.85346919708018,1.00000000005117,
8.13331267978517));
#150145=CARTESIAN_POINT('',(-3.45742808,1.69247211199998,8.309403774));
#150146=CARTESIAN_POINT('Ctrl Pts',(-3.61669496113721,1.69247211155784,
8.24132984160231));
#150147=CARTESIAN_POINT('Ctrl Pts',(-3.61474662287773,1.69743933229287,
8.24218486685928));
#150148=CARTESIAN_POINT('Ctrl Pts',(-3.61257269064703,1.702241310617,8.24313807944231));
#150149=CARTESIAN_POINT('Ctrl Pts',(-3.60299401241552,1.72064855672633,
8.24733263725374));
#150150=CARTESIAN_POINT('Ctrl Pts',(-3.59401446977586,1.73230722810795,
8.25125374075691));
#150151=CARTESIAN_POINT('Ctrl Pts',(-3.57692092613147,1.74686546539135,
8.25867362751413));
#150152=CARTESIAN_POINT('Ctrl Pts',(-3.56944743664773,1.75155833645782,
8.26190801991309));
#150153=CARTESIAN_POINT('Ctrl Pts',(-3.55354136548706,1.75781013613199,
8.2687613781201));
#150154=CARTESIAN_POINT('Ctrl Pts',(-3.54545632746744,1.75940739574123,
8.2722318365261));
#150155=CARTESIAN_POINT('Ctrl Pts',(-3.53722528439024,1.75940739573665,
8.27574995317466));
#150156=CARTESIAN_POINT('Ctrl Pts',(-3.52819299076565,1.75940739573161,
8.27961054074264));
#150157=CARTESIAN_POINT('Ctrl Pts',(-3.51924303306519,1.75748289650574,
8.28341809051765));
#150158=CARTESIAN_POINT('Ctrl Pts',(-3.50125398036883,1.74964163087026,
8.29103883882883));
#150159=CARTESIAN_POINT('Ctrl Pts',(-3.49261475617683,1.74349822231932,
8.29467967438141));
#150160=CARTESIAN_POINT('Ctrl Pts',(-3.47540112164682,1.72630637145233,
8.3019091043172));
#150161=CARTESIAN_POINT('Ctrl Pts',(-3.46753263756868,1.71456563888475,
8.30519482413073));
#150162=CARTESIAN_POINT('Ctrl Pts',(-3.46000302790207,1.69868853650819,
8.30833204968783));
#150163=CARTESIAN_POINT('Ctrl Pts',(-3.45866824382614,1.69560796570203,
8.30888775850462));
#150164=CARTESIAN_POINT('Ctrl Pts',(-3.45742807947873,1.69247211216521,
8.30940377375128));
#150165=CARTESIAN_POINT('Ctrl Pts',(-3.21572799916628,1.00000000027708,
8.40589634931207));
#150166=CARTESIAN_POINT('Ctrl Pts',(-3.22770818794205,1.04120750338201,
8.40131325348498));
#150167=CARTESIAN_POINT('Ctrl Pts',(-3.24017494826639,1.08227801762046,
8.39651460834608));
#150168=CARTESIAN_POINT('Ctrl Pts',(-3.31337492842116,1.31475831887219,
8.36813777565844));
#150169=CARTESIAN_POINT('Ctrl Pts',(-3.3828345982506,1.50385659929336,8.34044109045195));
#150170=CARTESIAN_POINT('Ctrl Pts',(-3.45742807919782,1.69247211229553,
8.30940377386816));
#150171=CARTESIAN_POINT('',(-2.8633881,1.69247211199998,8.532350707));
#150172=CARTESIAN_POINT('Ctrl Pts',(-2.86338810042523,1.69247211217985,
8.53235070694725));
#150173=CARTESIAN_POINT('Ctrl Pts',(-2.93998297503229,1.50385659913088,
8.50664608461793));
#150174=CARTESIAN_POINT('Ctrl Pts',(-3.01051379221962,1.31475831866339,
8.48180346126633));
#150175=CARTESIAN_POINT('Ctrl Pts',(-3.08430882573711,1.08227801739708,
8.45501214257094));
#150176=CARTESIAN_POINT('Ctrl Pts',(-3.09685440167008,1.04120750319233,
8.45042350089905));
#150177=CARTESIAN_POINT('Ctrl Pts',(-3.10889173621482,1.00000000012129,
8.44599266945545));
#150178=CARTESIAN_POINT('',(-2.698660279,1.69247211199998,8.585874021));
#150179=CARTESIAN_POINT('Ctrl Pts',(-2.86338809984566,1.69247211191797,
8.53235070714175));
#150180=CARTESIAN_POINT('Ctrl Pts',(-2.86137096114923,1.6974393326637,8.53302764262381));
#150181=CARTESIAN_POINT('Ctrl Pts',(-2.85912033521171,1.70224131099841,
8.53378214807124));
#150182=CARTESIAN_POINT('Ctrl Pts',(-2.84920422065495,1.72064855713849,
8.53710119373168));
#150183=CARTESIAN_POINT('Ctrl Pts',(-2.83990934200021,1.73230722853934,
8.54020159203125));
#150184=CARTESIAN_POINT('Ctrl Pts',(-2.82221949840695,1.746865465846,8.54605935507156));
#150185=CARTESIAN_POINT('Ctrl Pts',(-2.81448616629377,1.75155833692005,
8.54861080832648));
#150186=CARTESIAN_POINT('Ctrl Pts',(-2.79802979800297,1.75781013660889,
8.55401076770457));
#150187=CARTESIAN_POINT('Ctrl Pts',(-2.78966621847436,1.75940739622565,
8.55674251784626));
#150188=CARTESIAN_POINT('Ctrl Pts',(-2.78115294960864,1.7594073962279,8.55950864658032));
#150189=CARTESIAN_POINT('Ctrl Pts',(-2.77181095693984,1.75940739623038,
8.56254404400076));
#150190=CARTESIAN_POINT('Ctrl Pts',(-2.76255572300507,1.75748289701186,
8.56553399767844));
#150191=CARTESIAN_POINT('Ctrl Pts',(-2.74395597033505,1.74964163139145,
8.57151154084736));
#150192=CARTESIAN_POINT('Ctrl Pts',(-2.73502516313974,1.74349822285107,
8.57436330538032));
#150193=CARTESIAN_POINT('Ctrl Pts',(-2.71723278454767,1.7263063720123,8.58002061345238));
#150194=CARTESIAN_POINT('Ctrl Pts',(-2.70910144702474,1.71456563946539,
8.58258778044829));
#150195=CARTESIAN_POINT('Ctrl Pts',(-2.7013209304805,1.69868853681972,8.58503742749617));
#150196=CARTESIAN_POINT('Ctrl Pts',(-2.69994170637387,1.69560796571128,
8.58547125010984));
#150197=CARTESIAN_POINT('Ctrl Pts',(-2.69866027920764,1.69247211186234,
8.58587402058911));
#150198=CARTESIAN_POINT('Ctrl Pts',(-2.44928368492693,1.00000000003541,
8.66031231715986));
#150199=CARTESIAN_POINT('Ctrl Pts',(-2.46162647047221,1.04120750294047,
8.65682156738601));
#150200=CARTESIAN_POINT('Ctrl Pts',(-2.47447319045865,1.08227801698034,
8.65315975197741));
#150201=CARTESIAN_POINT('Ctrl Pts',(-2.54992216866384,1.31475831816348,
8.63145875170902));
#150202=CARTESIAN_POINT('Ctrl Pts',(-2.62158492606628,1.50385659870848,
8.61009988199061));
#150203=CARTESIAN_POINT('Ctrl Pts',(-2.69866027926731,1.69247211183557,
8.58587402057035));
#150204=CARTESIAN_POINT('',(-2.08702692,1.69247211199998,8.754674102));
#150205=CARTESIAN_POINT('Ctrl Pts',(-2.08702692043405,1.69247211217429,
8.75467410206591));
#150206=CARTESIAN_POINT('Ctrl Pts',(-2.1656175912421,1.50385659900165,8.73593887060451));
#150207=CARTESIAN_POINT('Ctrl Pts',(-2.2380913477429,1.31475831841118,8.71751859004947));
#150208=CARTESIAN_POINT('Ctrl Pts',(-2.31399085943843,1.08227801716552,
8.69745006113723));
#150209=CARTESIAN_POINT('Ctrl Pts',(-2.32689725319462,1.04120750310917,
8.69400446875687));
#150210=CARTESIAN_POINT('Ctrl Pts',(-2.33928330559696,1.00000000018754,
8.69067049289958));
#150211=CARTESIAN_POINT('',(-1.918164453,1.69247211199998,8.793215858));
#150212=CARTESIAN_POINT('Ctrl Pts',(-2.08702692043181,1.69247211217334,
8.75467410206645));
#150213=CARTESIAN_POINT('Ctrl Pts',(-2.08495722210436,1.69743933294414,
8.75516749748885));
#150214=CARTESIAN_POINT('Ctrl Pts',(-2.08264802316623,1.70224131130219,
8.75571722096838));
#150215=CARTESIAN_POINT('Ctrl Pts',(-2.0724743109975,1.72064855744848,8.7581340314743));
#150216=CARTESIAN_POINT('Ctrl Pts',(-2.06293893323256,1.73230722883563,
8.76038876198234));
#150217=CARTESIAN_POINT('Ctrl Pts',(-2.044795217923,1.74686546612392,8.76463723803522));
#150218=CARTESIAN_POINT('Ctrl Pts',(-2.03686430742723,1.75155833719122,
8.76648520934269));
#150219=CARTESIAN_POINT('Ctrl Pts',(-2.01999013901601,1.75781013686931,
8.77038829258981));
#150220=CARTESIAN_POINT('Ctrl Pts',(-2.01141535660801,1.75940739648177,
8.77235934001888));
#150221=CARTESIAN_POINT('Ctrl Pts',(-2.00268840579558,1.75940739648129,
8.77435120959334));
#150222=CARTESIAN_POINT('Ctrl Pts',(-1.99311193031393,1.75940739648077,
8.7765369776299));
#150223=CARTESIAN_POINT('Ctrl Pts',(-1.98362593784728,1.75748289725882,
8.7786852618597));
#150224=CARTESIAN_POINT('Ctrl Pts',(-1.96456523947057,1.74964163163066,
8.78297147222287));
#150225=CARTESIAN_POINT('Ctrl Pts',(-1.95541475487495,1.743498223085,8.7850112050058));
#150226=CARTESIAN_POINT('Ctrl Pts',(-1.93718688597779,1.72630637223327,
8.78905084189893));
#150227=CARTESIAN_POINT('Ctrl Pts',(-1.92885816375222,1.71456563967816,
8.79087878675951));
#150228=CARTESIAN_POINT('Ctrl Pts',(-1.92088938462464,1.69868853704812,
8.79262113211973));
#150229=CARTESIAN_POINT('Ctrl Pts',(-1.91947682532086,1.69560796596479,
8.79292957559287));
#150230=CARTESIAN_POINT('Ctrl Pts',(-1.91816445274598,1.69247211214182,
8.79321585838888));
#150231=CARTESIAN_POINT('Ctrl Pts',(-1.66311917827957,0.999999999892244,
8.84500054261382));
#150232=CARTESIAN_POINT('Ctrl Pts',(-1.67572518383153,1.04120750292225,
8.84263024433131));
#150233=CARTESIAN_POINT('Ctrl Pts',(-1.6888484293412,1.0822780170862,8.84013474140826));
#150234=CARTESIAN_POINT('Ctrl Pts',(-1.76593893483276,1.31475831833986,
8.82528429724149));
#150235=CARTESIAN_POINT('Ctrl Pts',(-1.83922779333879,1.50385659883379,
8.81043521210152));
#150236=CARTESIAN_POINT('Ctrl Pts',(-1.91816445327559,1.6924721119096,8.79321585827335));
#150237=CARTESIAN_POINT('',(-1.293862227,1.69247211199998,8.906510009));
#150238=CARTESIAN_POINT('Ctrl Pts',(-1.29386222704835,1.69247211203085,
8.9065100088316));
#150239=CARTESIAN_POINT('Ctrl Pts',(-1.37381592810969,1.50385659888228,
8.89489501332681));
#150240=CARTESIAN_POINT('Ctrl Pts',(-1.44764910778166,1.31475831831576,
8.88304538485746));
#150241=CARTESIAN_POINT('Ctrl Pts',(-1.52504199941119,1.08227801709192,
8.86986122572234));
#150242=CARTESIAN_POINT('Ctrl Pts',(-1.53820529634083,1.04120750303301,
8.86758642450121));
#150243=CARTESIAN_POINT('Ctrl Pts',(-1.55084034142984,1.0000000001088,8.86537614742848));
#150244=CARTESIAN_POINT('',(-1.12222469370069,1.69247211186443,8.92975989245309));
#150245=CARTESIAN_POINT('Ctrl Pts',(-1.29386222678592,1.69247211191724,
8.90651000886973));
#150246=CARTESIAN_POINT('Ctrl Pts',(-1.29175663284455,1.69743933264429,
8.90681589169734));
#150247=CARTESIAN_POINT('Ctrl Pts',(-1.28940745324758,1.70224131096107,
8.90715640715207));
#150248=CARTESIAN_POINT('Ctrl Pts',(-1.27905805625228,1.72064855707096,
8.90865152375763));
#150249=CARTESIAN_POINT('Ctrl Pts',(-1.26935895263151,1.73230722845912,
8.9100424327097));
#150250=CARTESIAN_POINT('Ctrl Pts',(-1.25090744812926,1.74686546574981,
8.91264741554435));
#150251=CARTESIAN_POINT('Ctrl Pts',(-1.24284281427572,1.75155833681844,
8.91377702612638));
#150252=CARTESIAN_POINT('Ctrl Pts',(-1.22568670661819,1.75781013649756,
8.9161518079123));
#150253=CARTESIAN_POINT('Ctrl Pts',(-1.21696976043267,1.75940739610974,
8.91734628291441));
#150254=CARTESIAN_POINT('Ctrl Pts',(-1.20809939194526,1.75940739610823,
8.91854785596744));
#150255=CARTESIAN_POINT('Ctrl Pts',(-1.19836553780408,1.75940739610657,
8.91986639609967));
#150256=CARTESIAN_POINT('Ctrl Pts',(-1.18872516244254,1.75748289688385,
8.92115571415885));
#150257=CARTESIAN_POINT('Ctrl Pts',(-1.1693569839014,1.74964163125455,8.92371608166787));
#150258=CARTESIAN_POINT('Ctrl Pts',(-1.1600604962301,1.743498222708,8.92492735997031));
#150259=CARTESIAN_POINT('Ctrl Pts',(-1.14154389711404,1.72630637185313,
8.92731680090106));
#150260=CARTESIAN_POINT('Ctrl Pts',(-1.13308484816047,1.71456563929489,
8.92839080608825));
#150261=CARTESIAN_POINT('Ctrl Pts',(-1.12499196639287,1.69868853672591,
8.92941182141991));
#150262=CARTESIAN_POINT('Ctrl Pts',(-1.12355744500622,1.69560796570946,
8.92959240234686));
#150263=CARTESIAN_POINT('Ctrl Pts',(-1.12222469348958,1.69247211195553,
8.92975989247876));
#150264=CARTESIAN_POINT('Ctrl Pts',(-0.863564213439779,0.999999999851497,
8.95847402459069));
#150265=CARTESIAN_POINT('Ctrl Pts',(-0.87633194283773,1.04120750294903,
8.95724326205628));
#150266=CARTESIAN_POINT('Ctrl Pts',(-0.889626053196569,1.08227801718005,
8.95593416395052));
#150267=CARTESIAN_POINT('Ctrl Pts',(-0.967737398493407,1.31475831834263,
8.94805384294514));
#150268=CARTESIAN_POINT('Ctrl Pts',(-1.04206227925682,1.503856598683,8.93983409849227));
#150269=CARTESIAN_POINT('Ctrl Pts',(-1.12222469430304,1.69247211160434,
8.92975989237653));
#150270=CARTESIAN_POINT('',(-0.490280117,1.69247211199998,8.986635934));
#150271=CARTESIAN_POINT('Ctrl Pts',(-0.490280116634963,1.69247211184778,
8.98663593383155));
#150272=CARTESIAN_POINT('Ctrl Pts',(-0.570953107639294,1.50385659894552,
8.98223469139443));
#150273=CARTESIAN_POINT('Ctrl Pts',(-0.645551249023955,1.31475831862389,
8.97705112125193));
#150274=CARTESIAN_POINT('Ctrl Pts',(-0.723814398508996,1.08227801747435,
8.97085748298641));
#150275=CARTESIAN_POINT('Ctrl Pts',(-0.737128615539831,1.04120750323641,
8.96977178828106));
#150276=CARTESIAN_POINT('Ctrl Pts',(-0.749910923411969,1.00000000013195,
8.96870300583911));
#150277=CARTESIAN_POINT('',(-0.317249442999998,1.69247211199998,8.99440675));
#150278=CARTESIAN_POINT('Ctrl Pts',(-0.490280117042471,1.6924721120226,
8.98663593380932));
#150279=CARTESIAN_POINT('Ctrl Pts',(-0.488155580485669,1.69743933273219,
8.98675184125671));
#150280=CARTESIAN_POINT('Ctrl Pts',(-0.485785334434531,1.70224131103289,
8.98688040706055));
#150281=CARTESIAN_POINT('Ctrl Pts',(-0.475343579860209,1.72064855714573,
8.98744179197277));
#150282=CARTESIAN_POINT('Ctrl Pts',(-0.465558841857883,1.73230722855105,
8.98795768059026));
#150283=CARTESIAN_POINT('Ctrl Pts',(-0.446948108818774,1.74686546586347,
8.98889819642085));
#150284=CARTESIAN_POINT('Ctrl Pts',(-0.438814683296168,1.75155833693935,
8.98930035131872));
#150285=CARTESIAN_POINT('Ctrl Pts',(-0.421514767281583,1.75781013663146,
8.99012771129987));
#150286=CARTESIAN_POINT('Ctrl Pts',(-0.412725841042246,1.75940739624973,
8.99053599666622));
#150287=CARTESIAN_POINT('Ctrl Pts',(-0.4037834738688,1.7594073962532,8.99093759883976));
#150288=CARTESIAN_POINT('Ctrl Pts',(-0.393970612336493,1.75940739625701,
8.99137829496011));
#150289=CARTESIAN_POINT('Ctrl Pts',(-0.384253472711392,1.75748289703985,
8.99179826602012));
#150290=CARTESIAN_POINT('Ctrl Pts',(-0.364733755191153,1.74964163142237,
8.9926121761055));
#150291=CARTESIAN_POINT('Ctrl Pts',(-0.355366114298903,1.74349822288404,
8.99298524742859));
#150292=CARTESIAN_POINT('Ctrl Pts',(-0.33670986974061,1.72630637205049,
8.99370525402672));
#150293=CARTESIAN_POINT('Ctrl Pts',(-0.328188601351913,1.71456563950727,
8.99401667228356));
#150294=CARTESIAN_POINT('Ctrl Pts',(-0.320036776042561,1.69868853696225,
8.99430813697986));
#150295=CARTESIAN_POINT('Ctrl Pts',(-0.318591842470321,1.69560796595495,
8.99435940143549));
#150296=CARTESIAN_POINT('Ctrl Pts',(-0.31724944252187,1.69247211221038,
8.99440675037657));
#150297=CARTESIAN_POINT('Ctrl Pts',(-0.0570563382849726,0.999999999911669,
8.99981914119731));
#150298=CARTESIAN_POINT('Ctrl Pts',(-0.0698829932121865,1.04120750284218,
8.99973782378958));
#150299=CARTESIAN_POINT('Ctrl Pts',(-0.0832409319874672,1.08227801690732,
8.99962567059222));
#150300=CARTESIAN_POINT('Ctrl Pts',(-0.161744210525077,1.31475831815756,
8.99877892044582));
#150301=CARTESIAN_POINT('Ctrl Pts',(-0.236506693492214,1.50385659874335,
8.9972546972045));
#150302=CARTESIAN_POINT('Ctrl Pts',(-0.317249443220438,1.69247211191093,
8.99440675035193));
#150303=CARTESIAN_POINT('',(0.317249442,1.69247211199998,8.99440675));
#150304=CARTESIAN_POINT('Ctrl Pts',(0.3172494417691,1.69247211210491,8.99440675040312));
#150305=CARTESIAN_POINT('Ctrl Pts',(0.236506691980429,1.50385659883905,
8.99725469724477));
#150306=CARTESIAN_POINT('Ctrl Pts',(0.161744208956719,1.3147583181561,8.99877892047435));
#150307=CARTESIAN_POINT('Ctrl Pts',(0.0832409304009244,1.08227801689511,
8.99962567060685));
#150308=CARTESIAN_POINT('Ctrl Pts',(0.0698829916511325,1.0412075029195,
8.99973782380167));
#150309=CARTESIAN_POINT('Ctrl Pts',(0.0570563367470327,1.00000000007913,
8.99981914120706));
#150310=CARTESIAN_POINT('',(0.490280117,1.69247211199998,8.986635934));
#150311=CARTESIAN_POINT('Ctrl Pts',(0.317249442367011,1.69247211184862,
8.99440675038203));
#150312=CARTESIAN_POINT('Ctrl Pts',(0.319375816065644,1.69743933266916,
8.99433174922977));
#150313=CARTESIAN_POINT('Ctrl Pts',(0.321748044801427,1.70224131107395,
8.99424733024544));
#150314=CARTESIAN_POINT('Ctrl Pts',(0.33219808615543,1.72064855725431,8.99387046351945));
#150315=CARTESIAN_POINT('Ctrl Pts',(0.34198967757272,1.73230722863321,8.99350717816731));
#150316=CARTESIAN_POINT('Ctrl Pts',(0.360609796449283,1.74686546591159,
8.99277565450731));
#150317=CARTESIAN_POINT('Ctrl Pts',(0.368746528075233,1.75155833697567,
8.99244711580377));
#150318=CARTESIAN_POINT('Ctrl Pts',(0.386050963682271,1.75781013664747,
8.99172039255882));
#150319=CARTESIAN_POINT('Ctrl Pts',(0.394841106701611,1.75940739625667,
8.99133920101302));
#150320=CARTESIAN_POINT('Ctrl Pts',(0.403783473868802,1.7594073962532,8.99093759883976));
#150321=CARTESIAN_POINT('Ctrl Pts',(0.413596335402248,1.75940739624939,
8.99049690271936));
#150322=CARTESIAN_POINT('Ctrl Pts',(0.423312002595504,1.75748289702423,
8.99004414541729));
#150323=CARTESIAN_POINT('Ctrl Pts',(0.44282609781397,1.74964163138951,8.98910504494812));
#150324=CARTESIAN_POINT('Ctrl Pts',(0.452189469197952,1.74349822283924,
8.98863690553838));
#150325=CARTESIAN_POINT('Ctrl Pts',(0.470835150104622,1.72630637197519,
8.98768168072916));
#150326=CARTESIAN_POINT('Ctrl Pts',(0.479350029693807,1.71456563941102,
8.98722800469669));
#150327=CARTESIAN_POINT('Ctrl Pts',(0.487495164855629,1.69868853682224,
8.98678757205289));
#150328=CARTESIAN_POINT('Ctrl Pts',(0.488938876868529,1.69560796579137,
8.98670910728539));
#150329=CARTESIAN_POINT('Ctrl Pts',(0.490280117042474,1.6924721120226,8.98663593380932));
#150330=CARTESIAN_POINT('Ctrl Pts',(0.749910923055971,1.00000000002074,
8.96870300586887));
#150331=CARTESIAN_POINT('Ctrl Pts',(0.737128615170063,1.04120750317642,
8.96977178831147));
#150332=CARTESIAN_POINT('Ctrl Pts',(0.723814398124095,1.08227801746521,
8.97085748301749));
#150333=CARTESIAN_POINT('Ctrl Pts',(0.645551248646327,1.31475831860558,
8.97705112127892));
#150334=CARTESIAN_POINT('Ctrl Pts',(0.570953107291636,1.503856598869,8.98223469141624));
#150335=CARTESIAN_POINT('Ctrl Pts',(0.490280116319866,1.69247211171261,
8.98663593384874));
#150336=CARTESIAN_POINT('',(1.122224693,1.69247211199998,8.929759892));
#150337=CARTESIAN_POINT('Ctrl Pts',(1.12222469326036,1.69247211191644,8.92975989250757));
#150338=CARTESIAN_POINT('Ctrl Pts',(1.04206227819181,1.50385659894457,8.9398340986166));
#150339=CARTESIAN_POINT('Ctrl Pts',(0.967737397408283,1.31475831855362,
8.94805384306261));
#150340=CARTESIAN_POINT('Ctrl Pts',(0.889626052114518,1.08227801739532,
8.95593416405797));
#150341=CARTESIAN_POINT('Ctrl Pts',(0.876331941773366,1.04120750322035,
8.95724326216039));
#150342=CARTESIAN_POINT('Ctrl Pts',(0.863564212391513,1.00000000017931,
8.95847402469174));
#150343=CARTESIAN_POINT('',(1.293862227,1.69247211199998,8.906510009));
#150344=CARTESIAN_POINT('Ctrl Pts',(1.12222469343999,1.69247211183887,8.92975989248499));
#150345=CARTESIAN_POINT('Ctrl Pts',(1.12433578390216,1.69743933257241,8.92949458660048));
#150346=CARTESIAN_POINT('Ctrl Pts',(1.12669089544509,1.70224131089559,8.9291978625228));
#150347=CARTESIAN_POINT('Ctrl Pts',(1.13706508588633,1.72064855702352,8.92788577847361));
#150348=CARTESIAN_POINT('Ctrl Pts',(1.14678469459136,1.73230722842326,8.92664624411455));
#150349=CARTESIAN_POINT('Ctrl Pts',(1.16526428107704,1.74686546572888,8.92424857076722));
#150350=CARTESIAN_POINT('Ctrl Pts',(1.17333880663464,1.75155833680264,8.92319198366484));
#150351=CARTESIAN_POINT('Ctrl Pts',(1.19050843670975,1.75781013649061,8.92091702834642));
#150352=CARTESIAN_POINT('Ctrl Pts',(1.19922902345515,1.75940739610672,8.91974942902085));
#150353=CARTESIAN_POINT('Ctrl Pts',(1.20809939194526,1.75940739610823,8.91854785596745));
#150354=CARTESIAN_POINT('Ctrl Pts',(1.21783324608598,1.75940739610989,8.91722931583528));
#150355=CARTESIAN_POINT('Ctrl Pts',(1.2274692160072,1.75748289689063,8.91590747550959));
#150356=CARTESIAN_POINT('Ctrl Pts',(1.24682057289392,1.74964163126884,8.91322292557665));
#150357=CARTESIAN_POINT('Ctrl Pts',(1.25610428640085,1.74349822272749,8.91191734462038));
#150358=CARTESIAN_POINT('Ctrl Pts',(1.27458927957878,1.72630637188588,8.90929457931835));
#150359=CARTESIAN_POINT('Ctrl Pts',(1.2830292135571,1.71456563933674,8.90807946173197));
#150360=CARTESIAN_POINT('Ctrl Pts',(1.29110207873021,1.69868853674836,8.90691067785349));
#150361=CARTESIAN_POINT('Ctrl Pts',(1.29253294526349,1.69560796570205,8.906703115614));
#150362=CARTESIAN_POINT('Ctrl Pts',(1.29386222678592,1.69247211191724,8.90651000886973));
#150363=CARTESIAN_POINT('Ctrl Pts',(1.5508403410948,1.00000000000293,8.86537614748709));
#150364=CARTESIAN_POINT('Ctrl Pts',(1.53820529599185,1.04120750297962,8.86758642456177));
#150365=CARTESIAN_POINT('Ctrl Pts',(1.52504199904688,1.08227801709064,8.869861225785));
#150366=CARTESIAN_POINT('Ctrl Pts',(1.44764910742439,1.31475831830606,8.88304538491551));
#150367=CARTESIAN_POINT('Ctrl Pts',(1.37381592778245,1.50385659881392,8.89489501337705));
#150368=CARTESIAN_POINT('Ctrl Pts',(1.29386222675378,1.69247211190334,8.9065100088744));
#150369=CARTESIAN_POINT('',(1.918164453,1.69247211199998,8.793215858));
#150370=CARTESIAN_POINT('Ctrl Pts',(1.91816445274452,1.69247211214243,8.7932158583892));
#150371=CARTESIAN_POINT('Ctrl Pts',(1.8392277928231,1.50385659907754,8.81043521220902));
#150372=CARTESIAN_POINT('Ctrl Pts',(1.76593893433233,1.31475831859373,8.82528429734154));
#150373=CARTESIAN_POINT('Ctrl Pts',(1.68884842884387,1.08227801731721,8.84013474150329));
#150374=CARTESIAN_POINT('Ctrl Pts',(1.67572518332552,1.04120750311924,8.84263024442721));
#150375=CARTESIAN_POINT('Ctrl Pts',(1.66311917776566,1.00000000005502,8.84500054271045));
#150376=CARTESIAN_POINT('',(2.08702692,1.69247211199998,8.754674102));
#150377=CARTESIAN_POINT('Ctrl Pts',(1.91816445274599,1.69247211214183,8.79321585838888));
#150378=CARTESIAN_POINT('Ctrl Pts',(1.92024326275655,1.69743933291712,8.79276238385459));
#150379=CARTESIAN_POINT('Ctrl Pts',(1.92256229518959,1.70224131127949,8.79225574372561));
#150380=CARTESIAN_POINT('Ctrl Pts',(1.93277710790527,1.72064855743365,8.79001900647378));
#150381=CARTESIAN_POINT('Ctrl Pts',(1.94234647731936,1.73230722882441,8.78791320310791));
#150382=CARTESIAN_POINT('Ctrl Pts',(1.96053674463815,1.74686546611737,8.78386868472646));
#150383=CARTESIAN_POINT('Ctrl Pts',(1.96848405279004,1.75155833718626,8.7820925562423));
#150384=CARTESIAN_POINT('Ctrl Pts',(1.9853806375546,1.75781013686712,8.77828768545105));
#150385=CARTESIAN_POINT('Ctrl Pts',(1.99396145498231,1.75940739648082,8.77634307916798));
#150386=CARTESIAN_POINT('Ctrl Pts',(2.00268840579558,1.75940739648129,8.77435120959334));
#150387=CARTESIAN_POINT('Ctrl Pts',(2.01226488127708,1.75940739648181,8.77216544155681));
#150388=CARTESIAN_POINT('Ctrl Pts',(2.0217435707649,1.75748289726097,8.7699851608862));
#150389=CARTESIAN_POINT('Ctrl Pts',(2.04077638358101,1.74964163163515,8.76557677590213));
#150390=CARTESIAN_POINT('Ctrl Pts',(2.04990569221387,1.7434982230911,8.76344426516706));
#150391=CARTESIAN_POINT('Ctrl Pts',(2.06808116737671,1.72630637224354,8.75917507633169));
#150392=CARTESIAN_POINT('Ctrl Pts',(2.07637820236166,1.71456563969128,8.75720830060181));
#150393=CARTESIAN_POINT('Ctrl Pts',(2.08431379958806,1.69868853706913,8.75532057584465));
#150394=CARTESIAN_POINT('Ctrl Pts',(2.08572030015038,1.69560796599098,8.7549855872994));
#150395=CARTESIAN_POINT('Ctrl Pts',(2.08702692043182,1.69247211217333,8.75467410206645));
#150396=CARTESIAN_POINT('Ctrl Pts',(2.33928330456152,0.999999999853761,
8.69067049317829));
#150397=CARTESIAN_POINT('Ctrl Pts',(2.32689725212173,1.04120750291753,8.69400446904408));
#150398=CARTESIAN_POINT('Ctrl Pts',(2.31399085832436,1.08227801711502,8.6974500614337));
#150399=CARTESIAN_POINT('Ctrl Pts',(2.23809134664659,1.31475831833215,8.71751859033044));
#150400=CARTESIAN_POINT('Ctrl Pts',(2.1656175902253,1.50385659875802,8.73593887085572));
#150401=CARTESIAN_POINT('Ctrl Pts',(2.08702691950425,1.69247211176485,8.75467410228757));
#150402=CARTESIAN_POINT('',(2.698660279,1.69247211199998,8.585874021));
#150403=CARTESIAN_POINT('Ctrl Pts',(2.69866027953189,1.69247211171677,8.58587402048719));
#150404=CARTESIAN_POINT('Ctrl Pts',(2.62158492637212,1.50385659866213,8.61009988189709));
#150405=CARTESIAN_POINT('Ctrl Pts',(2.54992216900827,1.3147583181889,8.63145875160704));
#150406=CARTESIAN_POINT('Ctrl Pts',(2.47447319081348,1.0822780170125,8.65315975187598));
#150407=CARTESIAN_POINT('Ctrl Pts',(2.46162647080814,1.04120750290523,8.65682156729051));
#150408=CARTESIAN_POINT('Ctrl Pts',(2.44928368524565,0.999999999932307,
8.66031231706972));
#150409=CARTESIAN_POINT('',(2.8633881,1.69247211199998,8.532350707));
#150410=CARTESIAN_POINT('Ctrl Pts',(2.69866027920764,1.69247211186232,8.58587402058911));
#150411=CARTESIAN_POINT('Ctrl Pts',(2.70069007140366,1.69743933265977,8.585236028515));
#150412=CARTESIAN_POINT('Ctrl Pts',(2.70295435323217,1.70224131104288,8.58452355150266));
#150413=CARTESIAN_POINT('Ctrl Pts',(2.7129275445438,1.7206485572087,8.58138016994169));
#150414=CARTESIAN_POINT('Ctrl Pts',(2.72226962772913,1.73230722859253,8.57842505226086));
#150415=CARTESIAN_POINT('Ctrl Pts',(2.74002411854311,1.74686546587729,8.57276625293123));
#150416=CARTESIAN_POINT('Ctrl Pts',(2.7477802222385,1.75155833694366,8.57028488340791));
#150417=CARTESIAN_POINT('Ctrl Pts',(2.76426772033127,1.7578101366193,8.56498073172689));
#150418=CARTESIAN_POINT('Ctrl Pts',(2.77263968074679,1.75940739623017,8.56227477531312));
#150419=CARTESIAN_POINT('Ctrl Pts',(2.78115294960864,1.75940739622791,8.55950864658032));
#150420=CARTESIAN_POINT('Ctrl Pts',(2.79049494227812,1.75940739622543,8.55647324915966));
#150421=CARTESIAN_POINT('Ctrl Pts',(2.79974003449488,1.7574828970017,8.5534520824834));
#150422=CARTESIAN_POINT('Ctrl Pts',(2.81830106221836,1.7496416313701,8.54735535617396));
#150423=CARTESIAN_POINT('Ctrl Pts',(2.82720246215092,1.74349822282198,8.54441308538322));
#150424=CARTESIAN_POINT('Ctrl Pts',(2.84492208106079,1.72630637196337,8.53853184601318));
#150425=CARTESIAN_POINT('Ctrl Pts',(2.85300941420689,1.71456563940287,8.53582924746147));
#150426=CARTESIAN_POINT('Ctrl Pts',(2.86074385070299,1.69868853678567,8.53323778068015));
#150427=CARTESIAN_POINT('Ctrl Pts',(2.86211466095963,1.69560796572133,8.53277806296399));
#150428=CARTESIAN_POINT('Ctrl Pts',(2.86338809984566,1.69247211191798,8.53235070714175));
#150429=CARTESIAN_POINT('Ctrl Pts',(3.1088917354371,1.00000000015544,8.44599266974173));
#150430=CARTESIAN_POINT('Ctrl Pts',(3.09685440089955,1.04120750319919,8.45042350118141));
#150431=CARTESIAN_POINT('Ctrl Pts',(3.08430882497446,1.08227801737684,8.45501214284914));
#150432=CARTESIAN_POINT('Ctrl Pts',(3.01051379149163,1.31475831853189,8.4818034615245));
#150433=CARTESIAN_POINT('Ctrl Pts',(2.93998297433824,1.50385659891702,8.5066460848574));
#150434=CARTESIAN_POINT('Ctrl Pts',(2.86338809976884,1.69247211188328,8.53235070716753));
#150435=CARTESIAN_POINT('',(3.45742808,1.69247211199998,8.309403774));
#150436=CARTESIAN_POINT('Ctrl Pts',(3.45742807951293,1.69247211214934,8.30940377373705));
#150437=CARTESIAN_POINT('Ctrl Pts',(3.38283459860251,1.50385659921542,8.34044109030884));
#150438=CARTESIAN_POINT('Ctrl Pts',(3.31337492880746,1.31475831886194,8.36813777550527));
#150439=CARTESIAN_POINT('Ctrl Pts',(3.24017494866242,1.08227801761983,8.39651460819329));
#150440=CARTESIAN_POINT('Ctrl Pts',(3.22770818832162,1.04120750332116,8.40131325333918));
#150441=CARTESIAN_POINT('Ctrl Pts',(3.21572799953086,1.00000000015557,8.4058963491726));
#150442=CARTESIAN_POINT('',(3.616694961,1.69247211199998,8.241329842));
#150443=CARTESIAN_POINT('Ctrl Pts',(3.45742807947874,1.69247211216523,8.30940377375128));
#150444=CARTESIAN_POINT('Ctrl Pts',(3.45939251105716,1.69743933261944,8.30858640091872));
#150445=CARTESIAN_POINT('Ctrl Pts',(3.46158381147327,1.70224131067939,8.30767382352641));
#150446=CARTESIAN_POINT('Ctrl Pts',(3.47123508293627,1.72064855658321,8.30364910638722));
#150447=CARTESIAN_POINT('Ctrl Pts',(3.48027466293952,1.73230722799961,8.29986846725986));
#150448=CARTESIAN_POINT('Ctrl Pts',(3.49745042854423,1.74686546532776,8.29264094830292));
#150449=CARTESIAN_POINT('Ctrl Pts',(3.5049528802026,1.75155833640984,8.28947431626728));
#150450=CARTESIAN_POINT('Ctrl Pts',(3.52089854399714,1.75781013611086,8.28271358960318));
#150451=CARTESIAN_POINT('Ctrl Pts',(3.52899424130546,1.75940739573206,8.27926806982646));
#150452=CARTESIAN_POINT('Ctrl Pts',(3.53722528439024,1.75940739573665,8.27574995317466));
#150453=CARTESIAN_POINT('Ctrl Pts',(3.54625757801351,1.75940739574168,8.27188936560725));
#150454=CARTESIAN_POINT('Ctrl Pts',(3.55519463691193,1.75748289652636,8.26805163758463));
#150455=CARTESIAN_POINT('Ctrl Pts',(3.57313443705392,1.74964163091365,8.26031565721045));
#150456=CARTESIAN_POINT('Ctrl Pts',(3.58173625944175,1.74349822237847,8.25658731580187));
#150457=CARTESIAN_POINT('Ctrl Pts',(3.59885735413302,1.72630637155177,8.24914137818544));
#150458=CARTESIAN_POINT('Ctrl Pts',(3.60666987098365,1.71456563901184,8.24572471654921));
#150459=CARTESIAN_POINT('Ctrl Pts',(3.61414087354956,1.6986885365718,8.24245037274111));
#150460=CARTESIAN_POINT('Ctrl Pts',(3.61546495648722,1.69560796567022,8.24186962725645));
#150461=CARTESIAN_POINT('Ctrl Pts',(3.61669496095015,1.69247211203475,8.2413298416844));
#150462=CARTESIAN_POINT('Ctrl Pts',(3.85346919584842,0.999999999908194,
8.13331268036877));
#150463=CARTESIAN_POINT('Ctrl Pts',(3.84187749678661,1.04120750281033,8.13880469291244));
#150464=CARTESIAN_POINT('Ctrl Pts',(3.82979374837064,1.08227801684729,8.1444994387919));
#150465=CARTESIAN_POINT('Ctrl Pts',(3.75869734727944,1.31475831804487,8.17779783928727));
#150466=CARTESIAN_POINT('Ctrl Pts',(3.69067734197139,1.50385659860643,8.20886278724963));
#150467=CARTESIAN_POINT('Ctrl Pts',(3.61669496034055,1.69247211174959,8.24132984195192));
#150468=CARTESIAN_POINT('',(4.188358703,1.69247211199998,7.966031093));
#150469=CARTESIAN_POINT('Ctrl Pts',(4.18835870309452,1.69247211195877,7.96603109297299));
#150470=CARTESIAN_POINT('Ctrl Pts',(4.11684767709352,1.50385659876227,8.00362997058505));
#150471=CARTESIAN_POINT('Ctrl Pts',(4.05015034311738,1.31475831814771,8.03744147392976));
#150472=CARTESIAN_POINT('Ctrl Pts',(3.97978872423844,1.08227801688172,8.07226566547244));
#150473=CARTESIAN_POINT('Ctrl Pts',(3.96780229871458,1.04120750283049,8.07816250443158));
#150474=CARTESIAN_POINT('Ctrl Pts',(3.95628116424985,0.999999999913974,
8.08380104588194));
#150475=CARTESIAN_POINT('',(4.340882323,1.69247211199998,7.883954633));
#150476=CARTESIAN_POINT('Ctrl Pts',(4.18835870300193,1.69247211200357,7.96603109302167));
#150477=CARTESIAN_POINT('Ctrl Pts',(4.19024195767693,1.69743933264773,7.96504092037285));
#150478=CARTESIAN_POINT('Ctrl Pts',(4.19234263382752,1.7022413108861,7.96393559005549));
#150479=CARTESIAN_POINT('Ctrl Pts',(4.20159427933326,1.72064855691514,7.95906194189284));
#150480=CARTESIAN_POINT('Ctrl Pts',(4.21025857475967,1.7323072282956,7.95448622080495));
#150481=CARTESIAN_POINT('Ctrl Pts',(4.22671732596282,1.74686546557696,7.94574817396074));
#150482=CARTESIAN_POINT('Ctrl Pts',(4.23390572024393,1.7515583366425,7.94192177527461));
#150483=CARTESIAN_POINT('Ctrl Pts',(4.24918116460586,1.75781013631569,7.93375890702995));
#150484=CARTESIAN_POINT('Ctrl Pts',(4.25693541699853,1.75940739592486,7.92960156519345));
#150485=CARTESIAN_POINT('Ctrl Pts',(4.26481796277002,1.75940739592063,7.92535978643457));
#150486=CARTESIAN_POINT('Ctrl Pts',(4.27346783463467,1.75940739591598,7.92070509189727));
#150487=CARTESIAN_POINT('Ctrl Pts',(4.28202490427402,1.75748289669031,7.91608170165456));
#150488=CARTESIAN_POINT('Ctrl Pts',(4.29919903612614,1.74964163105498,7.90676875277056));
#150489=CARTESIAN_POINT('Ctrl Pts',(4.30743202416367,1.7434982225042,7.90228435915017));
#150490=CARTESIAN_POINT('Ctrl Pts',(4.32381674566998,1.72630637163806,7.8933336735851));
#150491=CARTESIAN_POINT('Ctrl Pts',(4.33129154444121,1.71456563907157,7.88923045780917));
#150492=CARTESIAN_POINT('Ctrl Pts',(4.33843896105432,1.69868853654903,7.88529960002584));
#150493=CARTESIAN_POINT('Ctrl Pts',(4.33970565601871,1.69560796558959,7.88460250256148));
#150494=CARTESIAN_POINT('Ctrl Pts',(4.34088232285577,1.69247211189454,7.88395463324836));
#150495=CARTESIAN_POINT('Ctrl Pts',(4.56702079088812,0.999999999926177,
7.75514803827727));
#150496=CARTESIAN_POINT('Ctrl Pts',(4.55596805673791,1.04120750310877,7.7616570135297));
#150497=CARTESIAN_POINT('Ctrl Pts',(4.54444342694939,1.08227801742429,7.76841201294058));
#150498=CARTESIAN_POINT('Ctrl Pts',(4.47661808467104,1.31475831862242,7.80794939613996));
#150499=CARTESIAN_POINT('Ctrl Pts',(4.41165654848376,1.50385659891625,7.84498655197261));
#150500=CARTESIAN_POINT('Ctrl Pts',(4.34088232264359,1.69247211179079,7.88395463336519));
#150501=CARTESIAN_POINT('',(4.885567124,1.69247211199998,7.558520614));
#150502=CARTESIAN_POINT('Ctrl Pts',(4.88556712448749,1.69247211182252,7.55852061399102));
#150503=CARTESIAN_POINT('Ctrl Pts',(4.81771431823801,1.50385659859261,7.60237832854207));
#150504=CARTESIAN_POINT('Ctrl Pts',(4.75431632789338,1.31475831794536,7.64203241965308));
#150505=CARTESIAN_POINT('Ctrl Pts',(4.68735958066341,1.08227801668198,7.68302358613477));
#150506=CARTESIAN_POINT('Ctrl Pts',(4.67594999754258,1.0412075026676,7.68997114104926));
#150507=CARTESIAN_POINT('Ctrl Pts',(4.66498067874495,0.999999999788169,
7.69661972991627));
#150508=CARTESIAN_POINT('',(5.030119452,1.69247211199998,7.463102458));
#150509=CARTESIAN_POINT('Ctrl Pts',(4.88556712453282,1.69247211179936,7.55852061396171));
#150510=CARTESIAN_POINT('Ctrl Pts',(4.8873540394334,1.69743933262184,7.55736561377867));
#150511=CARTESIAN_POINT('Ctrl Pts',(4.88934717789494,1.7022413110283,7.55607642999802));
#150512=CARTESIAN_POINT('Ctrl Pts',(4.89812470861776,1.72064855720425,7.55039309055106));
#150513=CARTESIAN_POINT('Ctrl Pts',(4.90634395966117,1.7323072285775,7.54505912851645));
#150514=CARTESIAN_POINT('Ctrl Pts',(4.9219531802878,1.7468654658488,7.53488090739657));
#150515=CARTESIAN_POINT('Ctrl Pts',(4.92876964047146,1.75155833691055,7.5304255499714));
#150516=CARTESIAN_POINT('Ctrl Pts',(4.94325187651329,1.75781013657807,7.52092626275953));
#150517=CARTESIAN_POINT('Ctrl Pts',(4.95060225131441,1.75940739618523,7.51609057133398));
#150518=CARTESIAN_POINT('Ctrl Pts',(4.95807283415526,1.75940739618001,7.51115928277464));
#150519=CARTESIAN_POINT('Ctrl Pts',(4.96627064057822,1.75940739617429,7.50574795813151));
#150520=CARTESIAN_POINT('Ctrl Pts',(4.97437882446554,1.75748289694724,7.50037613048852));
#150521=CARTESIAN_POINT('Ctrl Pts',(4.99064901201179,1.74964163130848,7.48956119548553));
#150522=CARTESIAN_POINT('Ctrl Pts',(4.99844687851582,1.7434982227554,7.48435685535609));
#150523=CARTESIAN_POINT('Ctrl Pts',(5.01396330668295,1.72630637188402,7.47397348750486));
#150524=CARTESIAN_POINT('Ctrl Pts',(5.02104020468542,1.71456563931462,7.46921675427246));
#150525=CARTESIAN_POINT('Ctrl Pts',(5.02780648852956,1.69868853677723,7.46466103147771));
#150526=CARTESIAN_POINT('Ctrl Pts',(5.02900559682142,1.69560796580551,7.4638531946588));
#150527=CARTESIAN_POINT('Ctrl Pts',(5.03011945218954,1.69247211209781,7.46310245787263));
#150528=CARTESIAN_POINT('Ctrl Pts',(5.24380141833698,1.00000000010371,7.31454350489811));
#150529=CARTESIAN_POINT('Ctrl Pts',(5.23337663930275,1.04120750322152,7.32201703636989));
#150530=CARTESIAN_POINT('Ctrl Pts',(5.2225039177803,1.08227801747271,7.3297779019771));
#150531=CARTESIAN_POINT('Ctrl Pts',(5.15849572412172,1.314758318566,7.37523593608385));
#150532=CARTESIAN_POINT('Ctrl Pts',(5.09711568904592,1.50385659881995,7.41794709841542));
#150533=CARTESIAN_POINT('Ctrl Pts',(5.03011945133157,1.69247211165461,7.4631024584509));
#150534=CARTESIAN_POINT('',(5.54343983057962,1.69247211214185,7.09015337246368));
#150535=CARTESIAN_POINT('Ctrl Pts',(5.54343983074268,1.69247211204734,7.090153372314));
#150536=CARTESIAN_POINT('Ctrl Pts',(5.47979155526345,1.50385659906037,7.13991680716823));
#150537=CARTESIAN_POINT('Ctrl Pts',(5.42020335200143,1.31475831865458,7.185094214528));
#150538=CARTESIAN_POINT('Ctrl Pts',(5.35719057279498,1.08227801744158,7.23192231915544));
#150539=CARTESIAN_POINT('Ctrl Pts',(5.34644969527096,1.0412075032267,7.23986465243843));
#150540=CARTESIAN_POINT('Ctrl Pts',(5.33612051058942,1.00000000014546,7.24746975823059));
#150541=CARTESIAN_POINT('',(5.678857015,1.69247211099998,6.982161771));
#150542=CARTESIAN_POINT('Ctrl Pts',(5.54343983023426,1.69247211232382,7.09015337271151));
#150543=CARTESIAN_POINT('Ctrl Pts',(5.54511601804186,1.69743933283044,7.08884284446661));
#150544=CARTESIAN_POINT('Ctrl Pts',(5.54698557106645,1.70224131093972,7.08738018708892));
#150545=CARTESIAN_POINT('Ctrl Pts',(5.55521831528553,1.72064855688244,7.08093291540946));
#150546=CARTESIAN_POINT('Ctrl Pts',(5.56292634537749,1.73230722829274,7.07488365835215));
#150547=CARTESIAN_POINT('Ctrl Pts',(5.5775603591791,1.74686546561221,7.06334721200285));
#150548=CARTESIAN_POINT('Ctrl Pts',(5.5839500031433,1.75155833669097,7.05829876775497));
#150549=CARTESIAN_POINT('Ctrl Pts',(5.59752242843278,1.7578101363872,7.04753954424594));
#150550=CARTESIAN_POINT('Ctrl Pts',(5.60440974475557,1.7594073960068,7.04206443737231));
#150551=CARTESIAN_POINT('Ctrl Pts',(5.61140821593639,1.75940739601077,7.03648334284404));
#150552=CARTESIAN_POINT('Ctrl Pts',(5.61908795299923,1.75940739601513,7.03035895690422));
#150553=CARTESIAN_POINT('Ctrl Pts',(5.62668196880537,1.75748289679882,7.02428194266244));
#150554=CARTESIAN_POINT('Ctrl Pts',(5.64191721405738,1.7496416311835,7.01205209704974));
#150555=CARTESIAN_POINT('Ctrl Pts',(5.64921717518739,1.7434982226466,7.00616971270523));
#150556=CARTESIAN_POINT('Ctrl Pts',(5.66374038085026,1.72630637181616,6.99443726335541));
#150557=CARTESIAN_POINT('Ctrl Pts',(5.67036239905917,1.71456563927441,6.98906531109188));
#150558=CARTESIAN_POINT('Ctrl Pts',(5.67669307213169,1.69868853641841,6.98392140317849));
#150559=CARTESIAN_POINT('Ctrl Pts',(5.67781493935397,1.69560796508514,6.98300933113573));
#150560=CARTESIAN_POINT('Ctrl Pts',(5.67885701524478,1.69247211100408,6.98216177128582));
#150561=CARTESIAN_POINT('Ctrl Pts',(5.87836203940153,1.00000000015303,6.81504656871273));
#150562=CARTESIAN_POINT('Ctrl Pts',(5.86864914972266,1.04120750297626,6.82342448387522));
#150563=CARTESIAN_POINT('Ctrl Pts',(5.85851587727959,1.08227801693488,6.83212872970076));
#150564=CARTESIAN_POINT('Ctrl Pts',(5.79884018861094,1.31475831779691,6.88314141331103));
#150565=CARTESIAN_POINT('Ctrl Pts',(5.74153585055806,1.50385659810718,6.93118269699841));
#150566=CARTESIAN_POINT('Ctrl Pts',(5.6788570152349,1.69247211099862,6.98216177129386));
#150567=CARTESIAN_POINT('',(6.15668002,1.69247211199998,6.564700384));
#150568=CARTESIAN_POINT('Ctrl Pts',(6.15668002040536,1.69247211175397,6.56470038359266));
#150569=CARTESIAN_POINT('Ctrl Pts',(6.09774873405703,1.50385659870572,6.6199688729428));
#150570=CARTESIAN_POINT('Ctrl Pts',(6.04245008693597,1.31475831823908,6.67030585472521));
#150571=CARTESIAN_POINT('Ctrl Pts',(5.9838886175974,1.08227801704481,6.7225938651483));
#150572=CARTESIAN_POINT('Ctrl Pts',(5.97390292497523,1.04120750291262,6.73146702975377));
#150573=CARTESIAN_POINT('Ctrl Pts',(5.96429703900053,0.999999999914594,
6.73996742058666));
#150574=CARTESIAN_POINT('',(6.281871763,1.69247211199998,6.445004822));
#150575=CARTESIAN_POINT('Ctrl Pts',(6.15668002018172,1.69247211188528,6.56470038380239));
#150576=CARTESIAN_POINT('Ctrl Pts',(6.15823198538401,1.69743933273646,6.56324487896678));
#150577=CARTESIAN_POINT('Ctrl Pts',(6.15996290064518,1.70224131117035,6.56162052427874));
#150578=CARTESIAN_POINT('Ctrl Pts',(6.16758457340532,1.72064855738561,6.55446122979652));
#150579=CARTESIAN_POINT('Ctrl Pts',(6.17471932200875,1.73230722877144,6.54774538278063));
#150580=CARTESIAN_POINT('Ctrl Pts',(6.18826030448659,1.74686546605821,6.53494359589355));
#150581=CARTESIAN_POINT('Ctrl Pts',(6.19417168656544,1.75155833712512,6.52934271193098));
#150582=CARTESIAN_POINT('Ctrl Pts',(6.20672502389222,1.75781013680233,6.51741017907484));
#150583=CARTESIAN_POINT('Ctrl Pts',(6.21309382910321,1.75940739641427,6.51133973909936));
#150584=CARTESIAN_POINT('Ctrl Pts',(6.21956384103445,1.75940739641324,6.50515377430057));
#150585=CARTESIAN_POINT('Ctrl Pts',(6.22666367601188,1.75940739641211,6.49836563701203));
#150586=CARTESIAN_POINT('Ctrl Pts',(6.23368238118684,1.75748289718959,6.4916323647118));
#150587=CARTESIAN_POINT('Ctrl Pts',(6.24776001891509,1.74964163156032,6.47808607599983));
#150588=CARTESIAN_POINT('Ctrl Pts',(6.25450329968281,1.74349822301388,6.47157300893045));
#150589=CARTESIAN_POINT('Ctrl Pts',(6.26791635054222,1.72630637215997,6.45858594084604));
#150590=CARTESIAN_POINT('Ctrl Pts',(6.27403017236558,1.71456563960318,6.45264202134429));
#150591=CARTESIAN_POINT('Ctrl Pts',(6.27987426357281,1.69868853696114,6.44695134421518));
#150592=CARTESIAN_POINT('Ctrl Pts',(6.28090985690551,1.69560796586702,6.44594238057608));
#150593=CARTESIAN_POINT('Ctrl Pts',(6.28187176296278,1.69247211203292,6.44500482185164));
#150594=CARTESIAN_POINT('Ctrl Pts',(6.4655935474153,1.00000000002598,6.26067888328588));
#150595=CARTESIAN_POINT('Ctrl Pts',(6.45667074945246,1.04120750309549,6.2698937281947));
#150596=CARTESIAN_POINT('Ctrl Pts',(6.44735851311335,1.0822780172987,6.27947127288013));
#150597=CARTESIAN_POINT('Ctrl Pts',(6.39249580284863,1.31475831852555,6.3356278820062));
#150598=CARTESIAN_POINT('Ctrl Pts',(6.3397285426547,1.5038565989558,6.38861248690754));
#150599=CARTESIAN_POINT('Ctrl Pts',(6.28187176285276,1.69247211196711,6.44500482195888));
#150600=CARTESIAN_POINT('',(6.720350242,1.69247211199998,5.986392288));
#150601=CARTESIAN_POINT('Ctrl Pts',(6.72035024195089,1.69247211200555,5.98639228797367));
#150602=CARTESIAN_POINT('Ctrl Pts',(6.66661042481084,1.50385659891639,6.04672084242626));
#150603=CARTESIAN_POINT('Ctrl Pts',(6.61604656603123,1.31475831840883,6.10181211483949));
#150604=CARTESIAN_POINT('Ctrl Pts',(6.56240790905556,1.0822780171616,6.15913903875424));
#150605=CARTESIAN_POINT('Ctrl Pts',(6.55325780023637,1.04120750301805,6.16887159319523));
#150606=CARTESIAN_POINT('Ctrl Pts',(6.54445255389156,1.0000000000086,6.17819882893568));
#150607=CARTESIAN_POINT('',(6.834308572,1.69247211199998,5.855956484));
#150608=CARTESIAN_POINT('Ctrl Pts',(6.72035024189579,1.69247211204104,5.98639228803552));
#150609=CARTESIAN_POINT('Ctrl Pts',(6.72176548885911,1.69743933272173,5.98480352558652));
#150610=CARTESIAN_POINT('Ctrl Pts',(6.72334382988621,1.70224131099489,5.98303055207738));
#150611=CARTESIAN_POINT('Ctrl Pts',(6.73029306576593,1.72064855706964,5.97521687739583));
#150612=CARTESIAN_POINT('Ctrl Pts',(6.73679708808436,1.73230722846244,5.96788851247167));
#150613=CARTESIAN_POINT('Ctrl Pts',(6.7491360152204,1.74686546575904,5.95392445750275));
#150614=CARTESIAN_POINT('Ctrl Pts',(6.75452154044654,1.75155833682971,5.94781622884727));
#150615=CARTESIAN_POINT('Ctrl Pts',(6.76595471773228,1.75781013651241,5.93480646037549));
#150616=CARTESIAN_POINT('Ctrl Pts',(6.77175373396333,1.75940739612622,5.92818956290777));
#150617=CARTESIAN_POINT('Ctrl Pts',(6.77764319392101,1.75940739612599,5.92144853358502));
#150618=CARTESIAN_POINT('Ctrl Pts',(6.78410596311401,1.75940739612575,5.91405129904243));
#150619=CARTESIAN_POINT('Ctrl Pts',(6.79049284716903,1.75748289690448,5.90671598103713));
#150620=CARTESIAN_POINT('Ctrl Pts',(6.80329953250676,1.74964163127831,5.89196231598693));
#150621=CARTESIAN_POINT('Ctrl Pts',(6.80943183997698,1.74349822273394,5.8848710055844));
#150622=CARTESIAN_POINT('Ctrl Pts',(6.82162674202862,1.72630637188466,5.87073388301059));
#150623=CARTESIAN_POINT('Ctrl Pts',(6.82718314256654,1.71456563933029,5.86426585321872));
#150624=CARTESIAN_POINT('Ctrl Pts',(6.8324935987988,1.69868853674338,5.85807422480592));
#150625=CARTESIAN_POINT('Ctrl Pts',(6.83343458031894,1.69560796570414,5.85697649310469));
#150626=CARTESIAN_POINT('Ctrl Pts',(6.83430857189648,1.69247211192667,5.85595648413667));
#150627=CARTESIAN_POINT('Ctrl Pts',(7.00076789655382,0.999999999903773,
5.65590389403687));
#150628=CARTESIAN_POINT('Ctrl Pts',(6.99270703148499,1.04120750294805,5.66588147612623));
#150629=CARTESIAN_POINT('Ctrl Pts',(6.98429080796197,1.08227801712618,5.67625520685598));
#150630=CARTESIAN_POINT('Ctrl Pts',(6.93468279847114,1.31475831832256,5.73710360140728));
#150631=CARTESIAN_POINT('Ctrl Pts',(6.8868774671133,1.50385659874697,5.79460492660105));
#150632=CARTESIAN_POINT('Ctrl Pts',(6.83430857163229,1.69247211175275,5.855956484445));
#150633=CARTESIAN_POINT('',(7.229912155,1.69247211199998,5.359885281));
#150634=CARTESIAN_POINT('Ctrl Pts',(7.22991215493042,1.69247211222666,5.35988528160719));
#150635=CARTESIAN_POINT('Ctrl Pts',(7.18179648839481,1.50385659905977,5.42478817113771));
#150636=CARTESIAN_POINT('Ctrl Pts',(7.13637452840358,1.31475831847509,5.48419017167095));
#150637=CARTESIAN_POINT('Ctrl Pts',(7.08809055071595,1.08227801718246,5.54609444640032));
#150638=CARTESIAN_POINT('Ctrl Pts',(7.07984969700402,1.04120750307276,5.55660802986153));
#150639=CARTESIAN_POINT('Ctrl Pts',(7.07191598496283,1.00000000009741,5.56668701308303));
#150640=CARTESIAN_POINT('',(7.331719547,1.69247211199998,5.219759428));
#150641=CARTESIAN_POINT('Ctrl Pts',(7.2299121553839,1.69247211190049,5.3598852809955));
#150642=CARTESIAN_POINT('Ctrl Pts',(7.23117928939508,1.69743933249793,5.35817605269869));
#150643=CARTESIAN_POINT('Ctrl Pts',(7.23259234834446,1.70224131069262,5.35626873528853));
#150644=CARTESIAN_POINT('Ctrl Pts',(7.238813196219,1.72064855670081,5.34786359149694));
#150645=CARTESIAN_POINT('Ctrl Pts',(7.244634125688,1.732307228099,5.33998171234978));
#150646=CARTESIAN_POINT('Ctrl Pts',(7.25567165169417,1.74686546540359,5.32496781965828));
#150647=CARTESIAN_POINT('Ctrl Pts',(7.2604879589843,1.75155833647739,5.31840142617491));
#150648=CARTESIAN_POINT('Ctrl Pts',(7.2707089230063,1.75781013616434,5.30441916909239));
#150649=CARTESIAN_POINT('Ctrl Pts',(7.27589145998758,1.75940739577936,5.29730908949957));
#150650=CARTESIAN_POINT('Ctrl Pts',(7.28115294950206,1.7594073957793,5.29006727045673));
#150651=CARTESIAN_POINT('Ctrl Pts',(7.28692661849263,1.75940739577923,5.28212049684292));
#150652=CARTESIAN_POINT('Ctrl Pts',(7.29263025799211,1.75748289655852,5.27424219279993));
#150653=CARTESIAN_POINT('Ctrl Pts',(7.30406287903832,1.7496416309341,5.25839993924684));
#150654=CARTESIAN_POINT('Ctrl Pts',(7.30953483947673,1.74349822239083,5.25078748057241));
#150655=CARTESIAN_POINT('Ctrl Pts',(7.32041340653934,1.72630637154356,5.23561412730614));
#150656=CARTESIAN_POINT('Ctrl Pts',(7.32536764892156,1.71456563898964,5.22867406399609));
#150657=CARTESIAN_POINT('Ctrl Pts',(7.33010171347168,1.69868853658724,5.22203133570847));
#150658=CARTESIAN_POINT('Ctrl Pts',(7.33094050691844,1.69560796573972,5.22085367428564));
#150659=CARTESIAN_POINT('Ctrl Pts',(7.33171954712375,1.69247211216014,5.21975942762917));
#150660=CARTESIAN_POINT('Ctrl Pts',(7.47957617958273,1.00000000003768,5.00559089157501));
#150661=CARTESIAN_POINT('Ctrl Pts',(7.47244214875601,1.0412075030462,5.01625087721741));
#150662=CARTESIAN_POINT('Ctrl Pts',(7.4649897005347,1.08227801718884,5.0273372708077));
#150663=CARTESIAN_POINT('Ctrl Pts',(7.42103580633787,1.3147583184205,5.09238753530659));
#150664=CARTESIAN_POINT('Ctrl Pts',(7.37857730422629,1.50385659891382,5.15394261395913));
#150665=CARTESIAN_POINT('Ctrl Pts',(7.33171954689145,1.69247211198855,5.21975942795546));
#150666=CARTESIAN_POINT('',(7.681263067,1.69247211199998,4.69022363));
#150667=CARTESIAN_POINT('Ctrl Pts',(7.68126306643363,1.69247211231474,4.69022363051514));
#150668=CARTESIAN_POINT('Ctrl Pts',(7.63915894961858,1.50385659926452,4.75917829513542));
#150669=CARTESIAN_POINT('Ctrl Pts',(7.59924459938714,1.31475831879601,4.8224127537344));
#150670=CARTESIAN_POINT('Ctrl Pts',(7.55670405519824,1.08227801749227,4.88839596244951));
#150671=CARTESIAN_POINT('Ctrl Pts',(7.54943880707296,1.0412075032506,4.89960592578131));
#150672=CARTESIAN_POINT('Ctrl Pts',(7.54244050689292,1.00000000014238,4.91035550647617));
#150673=CARTESIAN_POINT('',(7.770099827,1.69247211199998,4.541535938));
#150674=CARTESIAN_POINT('Ctrl Pts',(7.68126306658055,1.69247211219402,4.69022363027453));
#150675=CARTESIAN_POINT('Ctrl Pts',(7.68237188542729,1.69743933272178,4.68840769783156));
#150676=CARTESIAN_POINT('Ctrl Pts',(7.68360828518667,1.70224131085111,4.68638139311887));
#150677=CARTESIAN_POINT('Ctrl Pts',(7.68905065845815,1.72064855681647,4.67745245349188));
#150678=CARTESIAN_POINT('Ctrl Pts',(7.69414162837983,1.73230722823068,4.66908052037508));
#150679=CARTESIAN_POINT('Ctrl Pts',(7.70378888559199,1.74686546555535,4.65313767299271));
#150680=CARTESIAN_POINT('Ctrl Pts',(7.7079971968728,1.75155833663596,4.64616598342078));
#150681=CARTESIAN_POINT('Ctrl Pts',(7.71692365444042,1.7578101363352,4.63132381464051));
#150682=CARTESIAN_POINT('Ctrl Pts',(7.72144798543253,1.75940739595606,4.6237777991027));
#150683=CARTESIAN_POINT('Ctrl Pts',(7.72603914208535,1.75940739596088,4.61609349720791));
#150684=CARTESIAN_POINT('Ctrl Pts',(7.73107722468816,1.75940739596616,4.60766116727051));
#150685=CARTESIAN_POINT('Ctrl Pts',(7.73605169728343,1.75748289675087,4.59930330866005));
#150686=CARTESIAN_POINT('Ctrl Pts',(7.74601820529917,1.74964163113786,4.58250001911516));
#150687=CARTESIAN_POINT('Ctrl Pts',(7.75078576169848,1.74349822260255,4.57442770321188));
#150688=CARTESIAN_POINT('Ctrl Pts',(7.76026040594584,1.72630637177601,4.55834028617848));
#150689=CARTESIAN_POINT('Ctrl Pts',(7.76457260152491,1.71456563923682,4.550984066663));
#150690=CARTESIAN_POINT('Ctrl Pts',(7.76869215858641,1.69868853671208,4.54394372171134));
#150691=CARTESIAN_POINT('Ctrl Pts',(7.76942201057286,1.69560796572158,4.54269561228855));
#150692=CARTESIAN_POINT('Ctrl Pts',(7.77009982710408,1.69247211199432,4.54153593807615));
#150693=CARTESIAN_POINT('Ctrl Pts',(7.89816331283004,0.999999999979972,
4.31497581498039));
#150694=CARTESIAN_POINT('Ctrl Pts',(7.8920135552809,1.04120750283238,4.3262323762081));
#150695=CARTESIAN_POINT('Ctrl Pts',(7.88558488510779,1.08227801681994,4.33794217150246));
#150696=CARTESIAN_POINT('Ctrl Pts',(7.84763899711798,1.31475831805313,4.40667055946035));
#150697=CARTESIAN_POINT('Ctrl Pts',(7.81086917512474,1.50385659869719,4.47178378631242));
#150698=CARTESIAN_POINT('Ctrl Pts',(7.77009982702068,1.69247211192352,4.54153593821884));
#150699=CARTESIAN_POINT('',(8.070768965,1.69247211199998,3.982799055));
#150700=CARTESIAN_POINT('Ctrl Pts',(8.07076896483245,1.69247211221444,3.98279905547562));
#150701=CARTESIAN_POINT('Ctrl Pts',(8.03501539529516,1.50385659911875,4.05525031284117));
#150702=CARTESIAN_POINT('Ctrl Pts',(8.00093002167116,1.31475831860448,4.12180810288602));
#150703=CARTESIAN_POINT('Ctrl Pts',(7.96447542245618,1.08227801735784,4.19133898755909));
#150704=CARTESIAN_POINT('Ctrl Pts',(7.95824427546741,1.04120750322134,4.20315507466474));
#150705=CARTESIAN_POINT('Ctrl Pts',(7.95223773338732,1.00000000021904,4.21448870347175));
#150706=CARTESIAN_POINT('',(8.14591983279771,1.69247211207413,3.82674667047894));
#150707=CARTESIAN_POINT('Ctrl Pts',(8.07076896488867,1.69247211216004,3.98279905536167));
#150708=CARTESIAN_POINT('Ctrl Pts',(8.07171054104207,1.69743933278747,3.98089103954382));
#150709=CARTESIAN_POINT('Ctrl Pts',(8.07276032688418,1.70224131101044,3.97876206207974));
#150710=CARTESIAN_POINT('Ctrl Pts',(8.07738040680553,1.72064855704371,3.96938121711269));
#150711=CARTESIAN_POINT('Ctrl Pts',(8.08170042767807,1.73230722844115,3.9605866359141));
#150712=CARTESIAN_POINT('Ctrl Pts',(8.08987974204302,1.74686546574377,3.94384319628412));
#150713=CARTESIAN_POINT('Ctrl Pts',(8.09344617446283,1.7515583368165,3.93652234257196));
#150714=CARTESIAN_POINT('Ctrl Pts',(8.10100625498024,1.75781013650272,3.92093976251732));
#150715=CARTESIAN_POINT('Ctrl Pts',(8.10483595272583,1.75940739611808,3.91301856711897));
#150716=CARTESIAN_POINT('Ctrl Pts',(8.10871981121782,1.75940739611904,3.90495365185858));
#150717=CARTESIAN_POINT('Ctrl Pts',(8.11298174375302,1.75940739612009,3.89610365775794));
#150718=CARTESIAN_POINT('Ctrl Pts',(8.11718699791387,1.75748289690017,3.88733353714228));
#150719=CARTESIAN_POINT('Ctrl Pts',(8.1256071484364,1.74964163127696,3.86970450180578));
#150720=CARTESIAN_POINT('Ctrl Pts',(8.12963191523693,1.74349822273463,3.86123732220919));
#150721=CARTESIAN_POINT('Ctrl Pts',(8.13762635240813,1.72630637189053,3.84436536781836));
#150722=CARTESIAN_POINT('Ctrl Pts',(8.14126178192232,1.71456563933969,3.83665222004586));
#150723=CARTESIAN_POINT('Ctrl Pts',(8.14473366319477,1.69868853683267,3.8292709432193));
#150724=CARTESIAN_POINT('Ctrl Pts',(8.14534869733938,1.69560796587296,3.82796243490335));
#150725=CARTESIAN_POINT('Ctrl Pts',(8.14591983278025,1.69247211217755,3.826746670204));
#150726=CARTESIAN_POINT('Ctrl Pts',(8.25315907928445,1.00000000000618,3.589619090102));
#150727=CARTESIAN_POINT('Ctrl Pts',(8.24804310921235,1.04120750292175,3.60138159575791));
#150728=CARTESIAN_POINT('Ctrl Pts',(8.2426899769243,1.08227801697206,3.61362051242964));
#150729=CARTESIAN_POINT('Ctrl Pts',(8.21105761312824,1.31475831812731,3.68547366326025));
#150730=CARTESIAN_POINT('Ctrl Pts',(8.18027252030632,1.50385659863499,3.75362078478248));
#150731=CARTESIAN_POINT('Ctrl Pts',(8.14591983233074,1.6924721117247,3.82674667116087));
#150732=CARTESIAN_POINT('',(8.395293776,1.69247211199998,3.243307326));
#150733=CARTESIAN_POINT('Ctrl Pts',(8.39529377643544,1.69247211171466,3.24330732545414));
#150734=CARTESIAN_POINT('Ctrl Pts',(8.36617862092618,1.50385659880013,3.31867184053676));
#150735=CARTESIAN_POINT('Ctrl Pts',(8.33819665932569,1.31475831846641,3.38801707774585));
#150736=CARTESIAN_POINT('Ctrl Pts',(8.30812151607705,1.08227801737161,3.460535816552));
#150737=CARTESIAN_POINT('Ctrl Pts',(8.30297463973184,1.04120750320158,3.47286289128436));
#150738=CARTESIAN_POINT('Ctrl Pts',(8.29800821687382,1.0000000001655,3.48468931652372));
#150739=CARTESIAN_POINT('',(8.456153681,1.69247211199998,3.081146689));
#150740=CARTESIAN_POINT('Ctrl Pts',(8.39529377630737,1.69247211186685,3.24330732578563));
#150741=CARTESIAN_POINT('Ctrl Pts',(8.39606052875182,1.69743933266438,3.24132258879396));
#150742=CARTESIAN_POINT('Ctrl Pts',(8.39691524842106,1.70224131104791,3.23910807982609));
#150743=CARTESIAN_POINT('Ctrl Pts',(8.40067583683032,1.72064855723031,3.22935085853306));
#150744=CARTESIAN_POINT('Ctrl Pts',(8.40419012638923,1.73230722862897,3.22020443804662));
#150745=CARTESIAN_POINT('Ctrl Pts',(8.41083564288388,1.74686546593259,3.20279521449446));
#150746=CARTESIAN_POINT('Ctrl Pts',(8.41373148162846,1.75155833700544,3.19518413985007));
#150747=CARTESIAN_POINT('Ctrl Pts',(8.4198643157783,1.75781013669251,3.17898661028975));
#150748=CARTESIAN_POINT('Ctrl Pts',(8.42296854580602,1.75940739630863,3.17075401183653));
#150749=CARTESIAN_POINT('Ctrl Pts',(8.42611383559583,1.75940739631059,3.16237341716321));
#150750=CARTESIAN_POINT('Ctrl Pts',(8.42956530348966,1.75940739631274,3.15317701384933));
#150751=CARTESIAN_POINT('Ctrl Pts',(8.43296748098366,1.75748289709378,3.14406524308343));
#150752=CARTESIAN_POINT('Ctrl Pts',(8.43977347991322,1.74964163147232,3.12575240058617));
#150753=CARTESIAN_POINT('Ctrl Pts',(8.44302305205915,1.74349822293125,3.11695853005104));
#150754=CARTESIAN_POINT('Ctrl Pts',(8.44947291564613,1.72630637209084,3.09943788136672));
#150755=CARTESIAN_POINT('Ctrl Pts',(8.45240230875442,1.71456563954306,3.0914299070713));
#150756=CARTESIAN_POINT('Ctrl Pts',(8.45519856073018,1.69868853687056,3.08376712797649));
#150757=CARTESIAN_POINT('Ctrl Pts',(8.45569382517283,1.69560796573518,3.08240875602405));
#150758=CARTESIAN_POINT('Ctrl Pts',(8.45615368110477,1.69247211185842,3.0811466893899));
#150759=CARTESIAN_POINT('Ctrl Pts',(8.54170526185697,0.999999999891995,
2.83536086231805));
#150760=CARTESIAN_POINT('Ctrl Pts',(8.53766427004687,1.04120750290419,2.84753460763075));
#150761=CARTESIAN_POINT('Ctrl Pts',(8.53342977591951,1.08227801705046,2.8602041051281));
#150762=CARTESIAN_POINT('Ctrl Pts',(8.50836562150266,1.31475831827597,2.93460349954225));
#150763=CARTESIAN_POINT('Ctrl Pts',(8.48381312130125,1.50385659875946,3.00523583521544));
#150764=CARTESIAN_POINT('Ctrl Pts',(8.45615368107749,1.6924721118243,3.08114668946476));
#150765=CARTESIAN_POINT('',(8.652224619,1.69247211199998,2.477702391));
#150766=CARTESIAN_POINT('Ctrl Pts',(8.65222461931465,1.69247211184308,2.47770239070909));
#150767=CARTESIAN_POINT('Ctrl Pts',(8.6299822958743,1.50385659864939,2.55537337297999));
#150768=CARTESIAN_POINT('Ctrl Pts',(8.6083290405278,1.31475831803842,2.62694773048628));
#150769=CARTESIAN_POINT('Ctrl Pts',(8.58487550058799,1.08227801688607,2.70187044525523));
#150770=CARTESIAN_POINT('Ctrl Pts',(8.58085433453559,1.04120750294561,2.7146092571805));
#150771=CARTESIAN_POINT('Ctrl Pts',(8.57696801764159,1.00000000014065,2.72683325936026));
#150772=CARTESIAN_POINT('',(8.69830355250517,1.69247211177544,2.31073912599594));
#150773=CARTESIAN_POINT('Ctrl Pts',(8.65222461924908,1.6924721119451,2.47770239093806));
#150774=CARTESIAN_POINT('Ctrl Pts',(8.65281037451573,1.69743933267269,2.47565691277349));
#150775=CARTESIAN_POINT('Ctrl Pts',(8.65346314627405,1.70224131098984,2.47337470231207));
#150776=CARTESIAN_POINT('Ctrl Pts',(8.65633396507629,1.72064855709382,2.46331966420916));
#150777=CARTESIAN_POINT('Ctrl Pts',(8.65901422832519,1.73230722847671,2.45389504603908));
#150778=CARTESIAN_POINT('Ctrl Pts',(8.66407244115264,1.74686546576066,2.43596020740361));
#150779=CARTESIAN_POINT('Ctrl Pts',(8.66627437062938,1.75155833682684,2.42812019172599));
#150780=CARTESIAN_POINT('Ctrl Pts',(8.67093058043353,1.75781013650178,2.41143812564637));
#150781=CARTESIAN_POINT('Ctrl Pts',(8.6732843493065,1.7594073961121,2.40296040818192));
#150782=CARTESIAN_POINT('Ctrl Pts',(8.67566574636791,1.75940739610916,2.3943316097188));
#150783=CARTESIAN_POINT('Ctrl Pts',(8.67827896042827,1.75940739610594,2.38486284122433));
#150784=CARTESIAN_POINT('Ctrl Pts',(8.68085066892037,1.75748289688156,2.37548278293022));
#150785=CARTESIAN_POINT('Ctrl Pts',(8.6859877183523,1.74964163124872,2.35663357751048));
#150786=CARTESIAN_POINT('Ctrl Pts',(8.68843593219854,1.74349822269971,2.34758381910881));
#150787=CARTESIAN_POINT('Ctrl Pts',(8.69328929169141,1.72630637183858,2.32955554208354));
#150788=CARTESIAN_POINT('Ctrl Pts',(8.69548906264279,1.71456563927602,2.3213172167611));
#150789=CARTESIAN_POINT('Ctrl Pts',(8.69758717149787,1.69868853665797,2.31343463170188));
#150790=CARTESIAN_POINT('Ctrl Pts',(8.69795867862005,1.69560796559486,2.31203733302424));
#150791=CARTESIAN_POINT('Ctrl Pts',(8.69830355251919,1.69247211179278,2.31073912595777));
#150792=CARTESIAN_POINT('Ctrl Pts',(8.76147865593336,0.999999999896204,
2.05827397632682));
#150793=CARTESIAN_POINT('Ctrl Pts',(8.75854517807591,1.0412075030467,2.07076094547247));
#150794=CARTESIAN_POINT('Ctrl Pts',(8.75546341576689,1.08227801733033,2.08375901646764));
#150795=CARTESIAN_POINT('Ctrl Pts',(8.73716927257158,1.31475831846967,2.16010563424933));
#150796=CARTESIAN_POINT('Ctrl Pts',(8.71904704729885,1.5038565987368,2.23265449395954));
#150797=CARTESIAN_POINT('Ctrl Pts',(8.69830355239435,1.6924721115845,2.3107391264277));
#150798=CARTESIAN_POINT('',(8.839492837,1.69247211199998,1.692148455));
#150799=CARTESIAN_POINT('Ctrl Pts',(8.83949283651609,1.69247211196709,1.69214845482919));
#150800=CARTESIAN_POINT('Ctrl Pts',(8.82430242730659,1.50385659886908,1.77150054300318));
#150801=CARTESIAN_POINT('Ctrl Pts',(8.80915221754667,1.31475831835278,1.84472774598003));
#150802=CARTESIAN_POINT('Ctrl Pts',(8.79250911503047,1.08227801717924,1.92145120303552));
#150803=CARTESIAN_POINT('Ctrl Pts',(8.78964603529871,1.04120750311893,1.93449918683023));
#150804=CARTESIAN_POINT('Ctrl Pts',(8.78687111467305,1.00000000019332,1.94702234556373));
#150805=CARTESIAN_POINT('',(8.870419798,1.69247211199998,1.521726851));
#150806=CARTESIAN_POINT('Ctrl Pts',(8.83949283655333,1.6924721118822,1.69214845463461));
#150807=CARTESIAN_POINT('Ctrl Pts',(8.83989287848787,1.69743933253477,1.6900587042909));
#150808=CARTESIAN_POINT('Ctrl Pts',(8.84033844660459,1.70224131078139,1.68772716736003));
#150809=CARTESIAN_POINT('Ctrl Pts',(8.84229638166108,1.72064855683246,1.67745526970955));
#150810=CARTESIAN_POINT('Ctrl Pts',(8.84412103869952,1.73230722822604,1.6678283353348));
#150811=CARTESIAN_POINT('Ctrl Pts',(8.84755122211043,1.74686546552434,1.64951228238133));
#150812=CARTESIAN_POINT('Ctrl Pts',(8.84904151368015,1.75155833659586,1.64150644886353));
#150813=CARTESIAN_POINT('Ctrl Pts',(8.85218361007993,1.75781013627923,1.62447416044409));
#150814=CARTESIAN_POINT('Ctrl Pts',(8.85376796663779,1.75940739589287,1.61581958156026));
#150815=CARTESIAN_POINT('Ctrl Pts',(8.8553662973649,1.75940739589201,1.60701205331319));
#150816=CARTESIAN_POINT('Ctrl Pts',(8.85712021753,1.75940739589105,1.59734715659617));
#150817=CARTESIAN_POINT('Ctrl Pts',(8.85884075113717,1.7574828966693,1.5877743334884));
#150818=CARTESIAN_POINT('Ctrl Pts',(8.86226749057167,1.74964163104244,1.56854052787078));
#150819=CARTESIAN_POINT('Ctrl Pts',(8.86389463454005,1.74349822249752,1.55930774494077));
#150820=CARTESIAN_POINT('Ctrl Pts',(8.86711241354167,1.7263063716463,1.54091699267151));
#150821=CARTESIAN_POINT('Ctrl Pts',(8.8685648510738,1.71456563908997,1.5325146464782));
#150822=CARTESIAN_POINT('Ctrl Pts',(8.86994792407433,1.69868853657767,1.5244757214109));
#150823=CARTESIAN_POINT('Ctrl Pts',(8.87019268272299,1.6956079656182,1.52305074624817));
#150824=CARTESIAN_POINT('Ctrl Pts',(8.87041979787082,1.69247211192306,1.52172685116002));
#150825=CARTESIAN_POINT('Ctrl Pts',(8.91070977542002,0.999999999993989,
1.26461507907905));
#150826=CARTESIAN_POINT('Ctrl Pts',(8.90890743017016,1.04120750304135,1.27731473425656));
#150827=CARTESIAN_POINT('Ctrl Pts',(8.9070032122354,1.08227801722256,1.2905367258509));
#150828=CARTESIAN_POINT('Ctrl Pts',(8.89562637393289,1.31475831840746,1.36821586896249));
#150829=CARTESIAN_POINT('Ctrl Pts',(8.88408033304455,1.50385659881792,1.44209713210709));
#150830=CARTESIAN_POINT('Ctrl Pts',(8.87041979782602,1.69247211180957,1.52172685142119));
#150831=CARTESIAN_POINT('',(8.955590655,1.69247211199998,0.892970333000003));
#150832=CARTESIAN_POINT('Ctrl Pts',(8.95559065523521,1.69247211204864,0.892970333137615));
#150833=CARTESIAN_POINT('Ctrl Pts',(8.94757446449693,1.50385659895089,0.973364630912383));
#150834=CARTESIAN_POINT('Ctrl Pts',(8.93904928090067,1.3147583184345,1.04765509702603));
#150835=CARTESIAN_POINT('Ctrl Pts',(8.92935061629266,1.0822780171992,1.12556156422249));
#150836=CARTESIAN_POINT('Ctrl Pts',(8.92766867472662,1.04120750307671,1.13881366517733));
#150837=CARTESIAN_POINT('Ctrl Pts',(8.92602749240836,1.00000000008849,1.15153515133937));
#150838=CARTESIAN_POINT('',(8.971116639,1.69247211199998,0.720462526000001));
#150839=CARTESIAN_POINT('Ctrl Pts',(8.95559065523919,1.69247211203143,0.892970333097603));
#150840=CARTESIAN_POINT('Ctrl Pts',(8.9558017629423,1.69743933257032,0.890853136027186));
#150841=CARTESIAN_POINT('Ctrl Pts',(8.95603653996893,1.7022413107097,0.888491044806472));
#150842=CARTESIAN_POINT('Ctrl Pts',(8.95706582714207,1.72064855666455,0.878084990907337));
#150843=CARTESIAN_POINT('Ctrl Pts',(8.95802018690319,1.73230722806018,0.868333250744331));
#150844=CARTESIAN_POINT('Ctrl Pts',(8.95979472307499,1.7468654653616,0.849783453564592));
#150845=CARTESIAN_POINT('Ctrl Pts',(8.96056137778506,1.75155833643442,0.841676260471873));
#150846=CARTESIAN_POINT('Ctrl Pts',(8.96216406246514,1.7578101361195,0.824430883686815));
#150847=CARTESIAN_POINT('Ctrl Pts',(8.96296625039909,1.7594073957336,0.815669124965459));
#150848=CARTESIAN_POINT('Ctrl Pts',(8.96376864597118,1.75940739573273,0.806753779975069));
#150849=CARTESIAN_POINT('Ctrl Pts',(8.96464915070661,1.75940739573177,0.796970571100184));
#150850=CARTESIAN_POINT('Ctrl Pts',(8.96550465670329,1.75748289651019,0.787282057921248));
#150851=CARTESIAN_POINT('Ctrl Pts',(8.9671934960484,1.74964163088392,0.767818511397058));
#150852=CARTESIAN_POINT('Ctrl Pts',(8.96798646933209,1.74349822233937,0.758477040876455));
#150853=CARTESIAN_POINT('Ctrl Pts',(8.96954276017722,1.72630637148872,0.739871884883412));
#150854=CARTESIAN_POINT('Ctrl Pts',(8.97023617011667,1.71456563893236,0.731373168568872));
#150855=CARTESIAN_POINT('Ctrl Pts',(8.97089307157979,1.69868853652994,0.723242628198454));
#150856=CARTESIAN_POINT('Ctrl Pts',(8.97100911110934,1.69560796568501,0.721801449619328));
#150857=CARTESIAN_POINT('Ctrl Pts',(8.97111663891427,1.6924721121081,0.720462525739917));
#150858=CARTESIAN_POINT('Ctrl Pts',(8.98819709930371,0.999999999959406,
0.460774244146091));
#150859=CARTESIAN_POINT('Ctrl Pts',(8.98754039807928,1.04120750304597,0.473584335238513));
#150860=CARTESIAN_POINT('Ctrl Pts',(8.98682905615476,1.08227801726612,0.486923791773002));
#150861=CARTESIAN_POINT('Ctrl Pts',(8.98246112236426,1.31475831853779,0.565310033439549));
#150862=CARTESIAN_POINT('Ctrl Pts',(8.9775842278123,1.50385659899527,0.639928851482268));
#150863=CARTESIAN_POINT('Ctrl Pts',(8.97111663890039,1.69247211203383,0.72046252591272));
#150864=CARTESIAN_POINT('',(8.999583324,1.69247211199998,0.0866025400000026));
#150865=CARTESIAN_POINT('Ctrl Pts',(8.99958332369346,1.69247211191239,0.0866025397925534));
#150866=CARTESIAN_POINT('Ctrl Pts',(8.99880589307639,1.50385659887802,0.16739175952592));
#150867=CARTESIAN_POINT('Ctrl Pts',(8.99697437540593,1.31475831842477,0.242147345601195));
#150868=CARTESIAN_POINT('Ctrl Pts',(8.99429823665167,1.08227801725348,0.320609565836492));
#150869=CARTESIAN_POINT('Ctrl Pts',(8.99381097525934,1.04120750313013,0.333959085808914));
#150870=CARTESIAN_POINT('Ctrl Pts',(8.9933167450867,1.00000000014106,0.3467764734569));
#150871=CARTESIAN_POINT('',(8.999583324,1.69247211199998,-0.0866025400000003));
#150872=CARTESIAN_POINT('Ctrl Pts',(8.9995833236904,1.69247211204886,-0.0866025401111396));
#150873=CARTESIAN_POINT('Ctrl Pts',(8.99959624897225,1.69560796569572,-0.0852593676028344));
#150874=CARTESIAN_POINT('Ctrl Pts',(8.99960986283583,1.69868853660841,-0.0838135890526297));
#150875=CARTESIAN_POINT('Ctrl Pts',(8.99968442188485,1.71456563907318,-0.0756568956210146));
#150876=CARTESIAN_POINT('Ctrl Pts',(8.99975562246681,1.72630637162691,-0.0671302358526971));
#150877=CARTESIAN_POINT('Ctrl Pts',(8.999873350116,1.74349822247422,-0.0484604739130545));
#150878=CARTESIAN_POINT('Ctrl Pts',(8.99992093207107,1.74964163101758,-0.03908552782939));
#150879=CARTESIAN_POINT('Ctrl Pts',(8.99998359035555,1.75748289664218,-0.0195489494290202));
#150880=CARTESIAN_POINT('Ctrl Pts',(9.,1.7594073958629,-0.00982275238873509));
#150881=CARTESIAN_POINT('Ctrl Pts',(9.,1.7594073958629,2.22044604925031E-15));
#150882=CARTESIAN_POINT('Ctrl Pts',(9.,1.7594073958629,0.00895138061714817));
#150883=CARTESIAN_POINT('Ctrl Pts',(8.99998643943525,1.75781013624804,0.0177497746457833));
#150884=CARTESIAN_POINT('Ctrl Pts',(8.999936070349,1.75155833656183,0.0350693901608712));
#150885=CARTESIAN_POINT('Ctrl Pts',(8.99989922515123,1.7468654654886,0.0432126684760403));
#150886=CARTESIAN_POINT('Ctrl Pts',(8.99979462373951,1.73230722818546,0.0618468578232667));
#150887=CARTESIAN_POINT('Ctrl Pts',(8.99971824519885,1.72064855678819,0.071644888497604));
#150888=CARTESIAN_POINT('Ctrl Pts',(8.99962589311285,1.70224131079953,0.0821013152925228));
#150889=CARTESIAN_POINT('Ctrl Pts',(8.99960379745391,1.69743933262498,0.0844749426937048));
#150890=CARTESIAN_POINT('Ctrl Pts',(8.9995833236904,1.69247211204887,0.0866025401111421));
#150891=CARTESIAN_POINT('Ctrl Pts',(8.99331674508599,1.00000000014682,-0.346776473475384));
#150892=CARTESIAN_POINT('Ctrl Pts',(8.99381097525864,1.04120750313464,-0.333959085827752));
#150893=CARTESIAN_POINT('Ctrl Pts',(8.99429823665098,1.08227801725674,-0.320609565855717));
#150894=CARTESIAN_POINT('Ctrl Pts',(8.99697437540542,1.31475831842863,-0.242147345620229));
#150895=CARTESIAN_POINT('Ctrl Pts',(8.99880589307606,1.50385659888367,-0.16739175954417));
#150896=CARTESIAN_POINT('Ctrl Pts',(8.9995833236933,1.69247211191984,-0.0866025398099395));
#150897=CARTESIAN_POINT('',(8.971116639,1.69247211199998,-0.720462525999999));
#150898=CARTESIAN_POINT('Ctrl Pts',(8.9711166389309,1.69247211219709,-0.720462525532798));
#150899=CARTESIAN_POINT('Ctrl Pts',(8.97758422784487,1.50385659904378,-0.639928851033996));
#150900=CARTESIAN_POINT('Ctrl Pts',(8.98246112239683,1.31475831847271,-0.565310032927709));
#150901=CARTESIAN_POINT('Ctrl Pts',(8.98682905618331,1.08227801719273,-0.486923791245081));
#150902=CARTESIAN_POINT('Ctrl Pts',(8.98754039810538,1.0412075030817,-0.473584334742424));
#150903=CARTESIAN_POINT('Ctrl Pts',(8.98819709932766,1.000000000105,-0.460774243678976));
#150904=CARTESIAN_POINT('',(8.955590655,1.69247211199998,-0.892970333000001));
#150905=CARTESIAN_POINT('Ctrl Pts',(8.97111663891427,1.69247211210811,-0.720462525739922));
#150906=CARTESIAN_POINT('Ctrl Pts',(8.97094631389629,1.69743933260741,-0.72258339330523));
#150907=CARTESIAN_POINT('Ctrl Pts',(8.97075555028735,1.70224131070957,-0.724949445788228));
#150908=CARTESIAN_POINT('Ctrl Pts',(8.96991022372286,1.72064855663687,-0.735372056421064));
#150909=CARTESIAN_POINT('Ctrl Pts',(8.96910800608785,1.7323072280393,-0.745137489624583));
#150910=CARTESIAN_POINT('Ctrl Pts',(8.96754183055015,1.74686546534951,-0.763706039604086));
#150911=CARTESIAN_POINT('Ctrl Pts',(8.96684856957967,1.7515583364253,-0.771819838253878));
#150912=CARTESIAN_POINT('Ctrl Pts',(8.96534621752964,1.75781013611549,-0.789074245141246));
#150913=CARTESIAN_POINT('Ctrl Pts',(8.96457104154341,1.75940739573185,-0.797838434983122));
#150914=CARTESIAN_POINT('Ctrl Pts',(8.96376864597118,1.75940739573272,-0.806753779975073));
#150915=CARTESIAN_POINT('Ctrl Pts',(8.96288814123577,1.75940739573368,-0.816536988849692));
#150916=CARTESIAN_POINT('Ctrl Pts',(8.96199994807101,1.7574828965141,-0.826222560130256));
#150917=CARTESIAN_POINT('Ctrl Pts',(8.96018629664472,1.74964163089217,-0.845674873362596));
#150918=CARTESIAN_POINT('Ctrl Pts',(8.95929854255293,1.74349822235062,-0.855007813454951));
#150919=CARTESIAN_POINT('Ctrl Pts',(8.95750774428347,1.72630637150763,-0.873591863395173));
#150920=CARTESIAN_POINT('Ctrl Pts',(8.95667250644543,1.71456563895651,-0.882077814966651));
#150921=CARTESIAN_POINT('Ctrl Pts',(8.95586708718875,1.69868853652541,-0.890194988511481));
#150922=CARTESIAN_POINT('Ctrl Pts',(8.95572392954189,1.69560796564499,-0.891633726431581));
#150923=CARTESIAN_POINT('Ctrl Pts',(8.95559065523919,1.69247211203143,-0.892970333097606));
#150924=CARTESIAN_POINT('Ctrl Pts',(8.9260274923892,1.0000000001351,-1.1515351514879));
#150925=CARTESIAN_POINT('Ctrl Pts',(8.92766867470473,1.04120750303497,-1.13881366534867));
#150926=CARTESIAN_POINT('Ctrl Pts',(8.92935061626786,1.0822780170697,-1.12556156441892));
#150927=CARTESIAN_POINT('Ctrl Pts',(8.93904928087935,1.31475831830307,-1.04765509721038));
#150928=CARTESIAN_POINT('Ctrl Pts',(8.94757446448273,1.50385659890226,-0.97336463104732));
#150929=CARTESIAN_POINT('Ctrl Pts',(8.95559065522704,1.69247211208388,-0.892970333219478));
#150930=CARTESIAN_POINT('',(8.870419798,1.69247211199998,-1.521726851));
#150931=CARTESIAN_POINT('Ctrl Pts',(8.87041979790224,1.69247211200266,-1.52172685097689));
#150932=CARTESIAN_POINT('Ctrl Pts',(8.88408033312625,1.50385659891321,-1.44209713160694));
#150933=CARTESIAN_POINT('Ctrl Pts',(8.89562637401809,1.31475831840579,-1.36821586841045));
#150934=CARTESIAN_POINT('Ctrl Pts',(8.90700321231731,1.08227801720866,-1.29053672528529));
#150935=CARTESIAN_POINT('Ctrl Pts',(8.90890743024755,1.04120750311532,-1.27731473371655));
#150936=CARTESIAN_POINT('Ctrl Pts',(8.91070977549335,1.00000000015644,-1.26461507856234));
#150937=CARTESIAN_POINT('',(8.83949283668534,1.69247211210181,-1.69214845452143));
#150938=CARTESIAN_POINT('Ctrl Pts',(8.87041979787082,1.69247211192305,-1.52172685116002));
#150939=CARTESIAN_POINT('Ctrl Pts',(8.87006004542175,1.69743933254887,-1.52382391295804));
#150940=CARTESIAN_POINT('Ctrl Pts',(8.86965795845286,1.70224131077038,-1.52616334054193));
#150941=CARTESIAN_POINT('Ctrl Pts',(8.86788175929939,1.72064855680533,-1.53646821838201));
#150942=CARTESIAN_POINT('Ctrl Pts',(8.86620740447288,1.73230722820551,-1.54612242858823));
#150943=CARTESIAN_POINT('Ctrl Pts',(8.86298306190944,1.74686546551235,-1.56447583615116));
#150944=CARTESIAN_POINT('Ctrl Pts',(8.86156527650011,1.7515583365868,-1.57249482759809));
#150945=CARTESIAN_POINT('Ctrl Pts',(8.85852229936856,1.75781013627524,-1.58954510351491));
#150946=CARTESIAN_POINT('Ctrl Pts',(8.85696462809229,1.75940739589114,-1.59820452506459));
#150947=CARTESIAN_POINT('Ctrl Pts',(8.8553662973649,1.759407395892,-1.60701205331319));
#150948=CARTESIAN_POINT('Ctrl Pts',(8.85361237719985,1.75940739589295,-1.61667695002996));
#150949=CARTESIAN_POINT('Ctrl Pts',(8.85185955172326,1.75748289667319,-1.62624391302741));
#150950=CARTESIAN_POINT('Ctrl Pts',(8.84830950960882,1.74964163105063,-1.64545534250641));
#150951=CARTESIAN_POINT('Ctrl Pts',(8.84658873105369,1.74349822250869,-1.65467113326303));
#150952=CARTESIAN_POINT('Ctrl Pts',(8.84313928061765,1.72630637166506,-1.67301984336281));
#150953=CARTESIAN_POINT('Ctrl Pts',(8.84154673036709,1.71456563911395,-1.68139676284534));
#150954=CARTESIAN_POINT('Ctrl Pts',(8.84001693566233,1.69868853665975,-1.68940906182158));
#150955=CARTESIAN_POINT('Ctrl Pts',(8.83974538685126,1.69560796575533,-1.69082917526325));
#150956=CARTESIAN_POINT('Ctrl Pts',(8.83949283657224,1.69247211211698,-1.69214845453584));
#150957=CARTESIAN_POINT('Ctrl Pts',(8.78687111482176,0.999999999979339,
-1.94702234489257));
#150958=CARTESIAN_POINT('Ctrl Pts',(8.78964603545235,1.04120750300605,-1.93449918613234));
#150959=CARTESIAN_POINT('Ctrl Pts',(8.79250911518946,1.08227801716676,-1.92145120230824));
#150960=CARTESIAN_POINT('Ctrl Pts',(8.80915221770156,1.31475831840232,-1.84472774523967));
#150961=CARTESIAN_POINT('Ctrl Pts',(8.8243024274504,1.5038565988819,-1.77150054228567));
#150962=CARTESIAN_POINT('Ctrl Pts',(8.8394928366488,1.69247211194256,-1.69214845413589));
#150963=CARTESIAN_POINT('',(8.698303553,1.69247211199998,-2.310739126));
#150964=CARTESIAN_POINT('Ctrl Pts',(8.69830355259779,1.69247211209572,-2.31073912566189));
#150965=CARTESIAN_POINT('Ctrl Pts',(8.71904704750919,1.5038565991313,-2.23265449314007));
#150966=CARTESIAN_POINT('Ctrl Pts',(8.7371692727865,1.31475831874759,-2.16010563338116));
#150967=CARTESIAN_POINT('Ctrl Pts',(8.75546341597935,1.08227801752857,-2.08375901557486));
#150968=CARTESIAN_POINT('Ctrl Pts',(8.75854517828406,1.04120750328463,-2.07076094459201));
#150969=CARTESIAN_POINT('Ctrl Pts',(8.76147865613757,1.00000000017415,-2.05827397545756));
#150970=CARTESIAN_POINT('',(8.652224619,1.69247211199998,-2.477702391));
#150971=CARTESIAN_POINT('Ctrl Pts',(8.69830355250322,1.69247211193793,-2.31073912601786));
#150972=CARTESIAN_POINT('Ctrl Pts',(8.69775726913674,1.69743933262652,-2.31279549771895));
#150973=CARTESIAN_POINT('Ctrl Pts',(8.69714709617372,1.70224131090741,-2.31508946468108));
#150974=CARTESIAN_POINT('Ctrl Pts',(8.69445432534046,1.7206485570025,-2.32519364087844));
#150975=CARTESIAN_POINT('Ctrl Pts',(8.69192131424337,1.73230722840754,-2.33465889806523));
#150976=CARTESIAN_POINT('Ctrl Pts',(8.6870647651655,1.74686546571993,-2.35264939236908));
#150977=CARTESIAN_POINT('Ctrl Pts',(8.68493387049238,1.75155833679612,-2.36050901241015));
#150978=CARTESIAN_POINT('Ctrl Pts',(8.6803747685432,1.75781013648825,-2.37721787856243));
#150979=CARTESIAN_POINT('Ctrl Pts',(8.67804714343072,1.75940739610622,-2.38570281125058));
#150980=CARTESIAN_POINT('Ctrl Pts',(8.6756657463679,1.75940739610916,-2.3943316097188));
#150981=CARTESIAN_POINT('Ctrl Pts',(8.6730525323078,1.75940739611239,-2.40380037821235));
#150982=CARTESIAN_POINT('Ctrl Pts',(8.67044918724008,1.75748289689477,-2.41317170536637));
#150983=CARTESIAN_POINT('Ctrl Pts',(8.6651913372909,1.74964163127651,-2.43198757195745));
#150984=CARTESIAN_POINT('Ctrl Pts',(8.66265138897059,1.74349822273761,-2.44101201324904));
#150985=CARTESIAN_POINT('Ctrl Pts',(8.65757105931702,1.72630637190226,-2.45897765048096));
#150986=CARTESIAN_POINT('Ctrl Pts',(8.65523401893332,1.7145656393574,-2.46717809184323));
#150987=CARTESIAN_POINT('Ctrl Pts',(8.65299216577075,1.6986885367743,-2.47502100598598));
#150988=CARTESIAN_POINT('Ctrl Pts',(8.65259441213127,1.69560796572895,-2.47641106107899));
#150989=CARTESIAN_POINT('Ctrl Pts',(8.65222461924908,1.6924721119451,-2.47770239093806));
#150990=CARTESIAN_POINT('Ctrl Pts',(8.57696801773418,1.00000000004553,-2.72683325906904));
#150991=CARTESIAN_POINT('Ctrl Pts',(8.58085433463339,1.0412075029207,-2.71460925687145));
#150992=CARTESIAN_POINT('Ctrl Pts',(8.58487550069146,1.08227801693089,-2.70187044492656));
#150993=CARTESIAN_POINT('Ctrl Pts',(8.60832904062519,1.31475831807767,-2.62694773016633));
#150994=CARTESIAN_POINT('Ctrl Pts',(8.62998229595736,1.50385659861581,-2.55537337269809));
#150995=CARTESIAN_POINT('Ctrl Pts',(8.65222461938352,1.69247211173591,-2.47770239046857));
#150996=CARTESIAN_POINT('',(8.456153681,1.69247211199998,-3.081146689));
#150997=CARTESIAN_POINT('Ctrl Pts',(8.45615368104301,1.69247211178115,-3.0811466895594));
#150998=CARTESIAN_POINT('Ctrl Pts',(8.48381312126247,1.50385659874205,-3.00523583532452));
#150999=CARTESIAN_POINT('Ctrl Pts',(8.50836562146028,1.31475831828407,-2.93460349966487));
#151000=CARTESIAN_POINT('Ctrl Pts',(8.53342977587719,1.08227801706105,-2.86020410525441));
#151001=CARTESIAN_POINT('Ctrl Pts',(8.53766427000695,1.04120750289092,-2.84753460775047));
#151002=CARTESIAN_POINT('Ctrl Pts',(8.54170526181922,0.999999999854697,
-2.83536086243177));
#151003=CARTESIAN_POINT('',(8.395293776,1.69247211199998,-3.243307326));
#151004=CARTESIAN_POINT('Ctrl Pts',(8.45615368110477,1.6924721118584,-3.08114668938989));
#151005=CARTESIAN_POINT('Ctrl Pts',(8.45542526516039,1.69743933268663,-3.08314581432304));
#151006=CARTESIAN_POINT('Ctrl Pts',(8.45461191894058,1.70224131109879,-3.08537585102182));
#151007=CARTESIAN_POINT('Ctrl Pts',(8.45102425701386,1.72064855729134,-3.09519797272746));
#151008=CARTESIAN_POINT('Ctrl Pts',(8.44765298396233,1.73230722867518,-3.10439806820348));
#151009=CARTESIAN_POINT('Ctrl Pts',(8.44120333044822,1.74686546595974,-3.12188080035487));
#151010=CARTESIAN_POINT('Ctrl Pts',(8.43837648322229,1.75155833702592,-3.12951776794703));
#151011=CARTESIAN_POINT('Ctrl Pts',(8.432337963664,1.75781013670153,-3.14575069436043));
#151012=CARTESIAN_POINT('Ctrl Pts',(8.42925912538441,1.75940739631255,-3.15399282249319));
#151013=CARTESIAN_POINT('Ctrl Pts',(8.42611383559583,1.75940739631059,-3.16237341716321));
#151014=CARTESIAN_POINT('Ctrl Pts',(8.42266236770178,1.75940739630844,-3.17156982047768));
#151015=CARTESIAN_POINT('Ctrl Pts',(8.41922946364508,1.75748289708497,-3.18067005937171));
#151016=CARTESIAN_POINT('Ctrl Pts',(8.41230613897276,1.74964163145378,-3.19893886878413));
#151017=CARTESIAN_POINT('Ctrl Pts',(8.40896747105483,1.74349822290598,-3.20769930111941));
#151018=CARTESIAN_POINT('Ctrl Pts',(8.4022971660049,1.72630637204838,-3.22513721674513));
#151019=CARTESIAN_POINT('Ctrl Pts',(8.39923445196042,1.71456563948878,-3.23309515485904));
#151020=CARTESIAN_POINT('Ctrl Pts',(8.39629859042414,1.69868853682826,-3.24070553759573));
#151021=CARTESIAN_POINT('Ctrl Pts',(8.39577783443639,1.69560796571781,-3.24205434239871));
#151022=CARTESIAN_POINT('Ctrl Pts',(8.39529377630737,1.69247211186687,-3.24330732578562));
#151023=CARTESIAN_POINT('Ctrl Pts',(8.29800821684455,0.999999999902031,
-3.48468931659343));
#151024=CARTESIAN_POINT('Ctrl Pts',(8.30297463971393,1.04120750304222,-3.47286289132727));
#151025=CARTESIAN_POINT('Ctrl Pts',(8.30812151607148,1.08227801731563,-3.4605358165655));
#151026=CARTESIAN_POINT('Ctrl Pts',(8.33819665933032,1.3147583184983,-3.38801707773433));
#151027=CARTESIAN_POINT('Ctrl Pts',(8.36617862092732,1.50385659881755,-3.31867184053366));
#151028=CARTESIAN_POINT('Ctrl Pts',(8.39529377643312,1.69247211171741,-3.24330732546012));
#151029=CARTESIAN_POINT('',(8.145919833,1.69247211199998,-3.82674667));
#151030=CARTESIAN_POINT('Ctrl Pts',(8.14591983253155,1.69247211163032,-3.8267466707334));
#151031=CARTESIAN_POINT('Ctrl Pts',(8.18027252047733,1.50385659864394,-3.75362078440848));
#151032=CARTESIAN_POINT('Ctrl Pts',(8.21105761327326,1.3147583182386,-3.68547366293637));
#151033=CARTESIAN_POINT('Ctrl Pts',(8.24268997705341,1.08227801715203,-3.61362051213516));
#151034=CARTESIAN_POINT('Ctrl Pts',(8.24804310934497,1.04120750306483,-3.6013815954542));
#151035=CARTESIAN_POINT('Ctrl Pts',(8.2531590794202,1.00000000011213,-3.58961908978988));
#151036=CARTESIAN_POINT('',(8.070768965,1.69247211199998,-3.982799055));
#151037=CARTESIAN_POINT('Ctrl Pts',(8.14591983282591,1.69247211192685,-3.82674667010681));
#151038=CARTESIAN_POINT('Ctrl Pts',(8.14501514910682,1.69743933265066,-3.8286724524188));
#151039=CARTESIAN_POINT('Ctrl Pts',(8.14400517824978,1.70224131096443,-3.8308206038134));
#151040=CARTESIAN_POINT('Ctrl Pts',(8.13955151101689,1.72064855707355,-3.84028158896136));
#151041=CARTESIAN_POINT('Ctrl Pts',(8.13536911951963,1.73230722846373,-3.84914244897219));
#151042=CARTESIAN_POINT('Ctrl Pts',(8.12737829038705,1.746865465757,-3.86597665830251));
#151043=CARTESIAN_POINT('Ctrl Pts',(8.12387825071992,1.75155833682648,-3.87332948507807));
#151044=CARTESIAN_POINT('Ctrl Pts',(8.11640893216073,1.75781013650711,-3.88895577378551));
#151045=CARTESIAN_POINT('Ctrl Pts',(8.11260366970907,1.75940739611999,-3.89688873659974));
#151046=CARTESIAN_POINT('Ctrl Pts',(8.10871981121782,1.75940739611904,-3.90495365185858));
#151047=CARTESIAN_POINT('Ctrl Pts',(8.1044578786825,1.75940739611799,-3.91380364595949));
#151048=CARTESIAN_POINT('Ctrl Pts',(8.10022305536408,1.75748289689589,-3.92255952681935));
#151049=CARTESIAN_POINT('Ctrl Pts',(8.09168999851365,1.74964163126794,-3.94013418933555));
#151050=CARTESIAN_POINT('Ctrl Pts',(8.08757949199219,1.74349822272231,-3.94856007886008));
#151051=CARTESIAN_POINT('Ctrl Pts',(8.07937291692609,1.72630637186985,-3.96532987302819));
#151052=CARTESIAN_POINT('Ctrl Pts',(8.07560918839591,1.71456563931328,-3.97298123525237));
#151053=CARTESIAN_POINT('Ctrl Pts',(8.07200295636026,1.69868853680513,-3.98029781215841));
#151054=CARTESIAN_POINT('Ctrl Pts',(8.07136339088196,1.69560796585033,-3.98159450680377));
#151055=CARTESIAN_POINT('Ctrl Pts',(8.07076896488867,1.69247211216003,-3.98279905536167));
#151056=CARTESIAN_POINT('Ctrl Pts',(7.95223773338533,1.0000000000746,-4.2144887034755));
#151057=CARTESIAN_POINT('Ctrl Pts',(7.95824427546704,1.04120750308548,-4.20315507466545));
#151058=CARTESIAN_POINT('Ctrl Pts',(7.96447542245755,1.08227801723046,-4.19133898755649));
#151059=CARTESIAN_POINT('Ctrl Pts',(8.00093002168167,1.31475831851661,-4.12180810286586));
#151060=CARTESIAN_POINT('Ctrl Pts',(8.03501539531451,1.50385659906093,-4.05525031280324));
#151061=CARTESIAN_POINT('Ctrl Pts',(8.07076896486063,1.69247211218716,-3.9827990554185));
#151062=CARTESIAN_POINT('',(7.770099827,1.69247211199998,-4.541535938));
#151063=CARTESIAN_POINT('Ctrl Pts',(7.77009982692731,1.69247211184427,-4.54153593837858));
#151064=CARTESIAN_POINT('Ctrl Pts',(7.81086917503205,1.50385659862522,-4.47178378647428));
#151065=CARTESIAN_POINT('Ctrl Pts',(7.84763899702609,1.31475831798857,-4.40667055962398));
#151066=CARTESIAN_POINT('Ctrl Pts',(7.88558488501719,1.08227801676247,-4.33794217166716));
#151067=CARTESIAN_POINT('Ctrl Pts',(7.89201355519076,1.04120750277453,-4.32623237637253));
#151068=CARTESIAN_POINT('Ctrl Pts',(7.89816331274033,0.999999999921735,
-4.31497581514458));
#151069=CARTESIAN_POINT('',(7.681263067,1.69247211199998,-4.69022363));
#151070=CARTESIAN_POINT('Ctrl Pts',(7.77009982710407,1.69247211199432,-4.54153593807615));
#151071=CARTESIAN_POINT('Ctrl Pts',(7.76902615958796,1.69743933266121,-4.54337287251751));
#151072=CARTESIAN_POINT('Ctrl Pts',(7.7678276957807,1.70224131092096,-4.54542184297812));
#151073=CARTESIAN_POINT('Ctrl Pts',(7.76254388154541,1.72064855696661,-4.55444551730448));
#151074=CARTESIAN_POINT('Ctrl Pts',(7.75758404575993,1.73230722834436,-4.56289579941117));
#151075=CARTESIAN_POINT('Ctrl Pts',(7.74811637846731,1.74686546562212,-4.57894594675687));
#151076=CARTESIAN_POINT('Ctrl Pts',(7.74397132662032,1.75155833668634,-4.58595543207492));
#151077=CARTESIAN_POINT('Ctrl Pts',(7.73513134762145,1.75781013635739,-4.60084926938084));
#151078=CARTESIAN_POINT('Ctrl Pts',(7.73063029873371,1.75940739596569,-4.60840919532057));
#151079=CARTESIAN_POINT('Ctrl Pts',(7.72603914208534,1.75940739596087,-4.61609349720791));
#151080=CARTESIAN_POINT('Ctrl Pts',(7.72100105948174,1.75940739595559,-4.62452582714664));
#151081=CARTESIAN_POINT('Ctrl Pts',(7.71599841320752,1.75748289672922,-4.63286685276752));
#151082=CARTESIAN_POINT('Ctrl Pts',(7.70592432733086,1.74964163109228,-4.64960586754053));
#151083=CARTESIAN_POINT('Ctrl Pts',(7.70107507758454,1.74349822254039,-4.65762937394834));
#151084=CARTESIAN_POINT('Ctrl Pts',(7.69139830701292,1.72630637167157,-4.6735960261417));
#151085=CARTESIAN_POINT('Ctrl Pts',(7.68696386732323,1.71456563910334,-4.68087920820853));
#151086=CARTESIAN_POINT('Ctrl Pts',(7.68271630004147,1.6986885366654,-4.68784307054307));
#151087=CARTESIAN_POINT('Ctrl Pts',(7.68196307447331,1.69560796579604,-4.68907721483747));
#151088=CARTESIAN_POINT('Ctrl Pts',(7.68126306658054,1.692472112194,-4.69022363027454));
#151089=CARTESIAN_POINT('Ctrl Pts',(7.54244050719113,0.999999999972247,
-4.91035550601811));
#151090=CARTESIAN_POINT('Ctrl Pts',(7.54943880738768,1.0412075031992,-4.89960592529646));
#151091=CARTESIAN_POINT('Ctrl Pts',(7.55670405553103,1.08227801755879,-4.88839596193518));
#151092=CARTESIAN_POINT('Ctrl Pts',(7.59924459970586,1.31475831885198,-4.82241275323143));
#151093=CARTESIAN_POINT('Ctrl Pts',(7.63915894989652,1.50385659919618,-4.75917829468802));
#151094=CARTESIAN_POINT('Ctrl Pts',(7.6812630666695,1.69247211212086,-4.69022363012885));
#151095=CARTESIAN_POINT('',(7.331719547,1.69247211199998,-5.219759428));
#151096=CARTESIAN_POINT('Ctrl Pts',(7.33171954715669,1.69247211218445,-5.2197594275829));
#151097=CARTESIAN_POINT('Ctrl Pts',(7.37857730449581,1.5038565990772,-5.15394261357347));
#151098=CARTESIAN_POINT('Ctrl Pts',(7.42103580661076,1.31475831855127,-5.09238753490902));
#151099=CARTESIAN_POINT('Ctrl Pts',(7.46498970082048,1.08227801722486,-5.02733727038339));
#151100=CARTESIAN_POINT('Ctrl Pts',(7.47244214905171,1.04120750302035,-5.01625087677695));
#151101=CARTESIAN_POINT('Ctrl Pts',(7.47957617988741,0.999999999949517,
-5.00559089111973));
#151102=CARTESIAN_POINT('',(7.229912155,1.69247211199998,-5.359885281));
#151103=CARTESIAN_POINT('Ctrl Pts',(7.33171954712374,1.69247211216015,-5.21975942762917));
#151104=CARTESIAN_POINT('Ctrl Pts',(7.33048554037461,1.69743933266443,-5.22149272425506));
#151105=CARTESIAN_POINT('Ctrl Pts',(7.32910823297432,1.70224131077121,-5.22342601663965));
#151106=CARTESIAN_POINT('Ctrl Pts',(7.32303681394073,1.72064855669899,-5.2319397267822));
#151107=CARTESIAN_POINT('Ctrl Pts',(7.31733946754646,1.7323072280976,-5.23991139428903));
#151108=CARTESIAN_POINT('Ctrl Pts',(7.30647119017968,1.74686546540271,-5.25504825331498));
#151109=CARTESIAN_POINT('Ctrl Pts',(7.30171449967183,1.75155833647675,-5.26165796092615));
#151110=CARTESIAN_POINT('Ctrl Pts',(7.29157503454324,1.75781013616406,-5.27569943042096));
#151111=CARTESIAN_POINT('Ctrl Pts',(7.2864144390166,1.75940739577923,-5.2828254514138));
#151112=CARTESIAN_POINT('Ctrl Pts',(7.28115294950206,1.7594073957793,-5.29006727045672));
#151113=CARTESIAN_POINT('Ctrl Pts',(7.27537928051152,1.75940739577936,-5.29801404407049));
#151114=CARTESIAN_POINT('Ctrl Pts',(7.26964908964958,1.7574828965588,-5.30587305741948));
#151115=CARTESIAN_POINT('Ctrl Pts',(7.25811508536945,1.74964163093468,-5.32164165174141));
#151116=CARTESIAN_POINT('Ctrl Pts',(7.25256613571055,1.74349822239163,-5.32919817447285));
#151117=CARTESIAN_POINT('Ctrl Pts',(7.24149708131024,1.7263063715449,-5.34423313058701));
#151118=CARTESIAN_POINT('Ctrl Pts',(7.23642763396644,1.71456563899135,-5.35108949259296));
#151119=CARTESIAN_POINT('Ctrl Pts',(7.23157293031562,1.69868853650539,-5.3576445714967));
#151120=CARTESIAN_POINT('Ctrl Pts',(7.23071210915306,1.69560796557039,-5.3588062288934));
#151121=CARTESIAN_POINT('Ctrl Pts',(7.2299121553839,1.69247211190049,-5.35988528099549));
#151122=CARTESIAN_POINT('Ctrl Pts',(7.07191598531854,0.999999999848429,
-5.56668701263112));
#151123=CARTESIAN_POINT('Ctrl Pts',(7.0798496973723,1.04120750290071,-5.55660802939234));
#151124=CARTESIAN_POINT('Ctrl Pts',(7.08809055109799,1.08227801708678,-5.54609444591211));
#151125=CARTESIAN_POINT('Ctrl Pts',(7.13637452878035,1.31475831838269,-5.48419017118036));
#151126=CARTESIAN_POINT('Ctrl Pts',(7.18179648874699,1.50385659889642,-5.42478817067091));
#151127=CARTESIAN_POINT('Ctrl Pts',(7.22991215525667,1.69247211199201,-5.35988528116711));
#151128=CARTESIAN_POINT('',(6.834308572,1.69247211199998,-5.855956484));
#151129=CARTESIAN_POINT('Ctrl Pts',(6.83430857185789,1.69247211190127,-5.85595648418171));
#151130=CARTESIAN_POINT('Ctrl Pts',(6.88687746734898,1.50385659885685,-5.79460492632121));
#151131=CARTESIAN_POINT('Ctrl Pts',(6.93468279871554,1.31475831839393,-5.73710360111202));
#151132=CARTESIAN_POINT('Ctrl Pts',(6.98429080820646,1.08227801718584,-5.67625520655512));
#151133=CARTESIAN_POINT('Ctrl Pts',(6.99270703172362,1.04120750303555,-5.66588147583171));
#151134=CARTESIAN_POINT('Ctrl Pts',(7.0007678967871,1.00000000001932,-5.65590389374811));
#151135=CARTESIAN_POINT('',(6.720350242,1.69247211199998,-5.986392288));
#151136=CARTESIAN_POINT('Ctrl Pts',(6.83430857189648,1.69247211192666,-5.85595648413667));
#151137=CARTESIAN_POINT('Ctrl Pts',(6.83292416134052,1.69743933264487,-5.85757218755852));
#151138=CARTESIAN_POINT('Ctrl Pts',(6.83137909952495,1.70224131095345,-5.85937423625887));
#151139=CARTESIAN_POINT('Ctrl Pts',(6.82456895907562,1.72064855706258,-5.86730943498248));
#151140=CARTESIAN_POINT('Ctrl Pts',(6.81817997375613,1.73230722845711,-5.87473830470636));
#151141=CARTESIAN_POINT('Ctrl Pts',(6.80599859129646,1.74686546575594,-5.88884000231498));
#151142=CARTESIAN_POINT('Ctrl Pts',(6.80066856020435,1.75155833682737,-5.89499671473559));
#151143=CARTESIAN_POINT('Ctrl Pts',(6.78931124596146,1.75781013651138,-5.90807276275262));
#151144=CARTESIAN_POINT('Ctrl Pts',(6.78353265387896,1.75940739612577,-5.91470750426196));
#151145=CARTESIAN_POINT('Ctrl Pts',(6.77764319392101,1.75940739612599,-5.92144853358502));
#151146=CARTESIAN_POINT('Ctrl Pts',(6.77118042472805,1.75940739612624,-5.92884576812756));
#151147=CARTESIAN_POINT('Ctrl Pts',(6.76476882540303,1.75748289690548,-5.93615949305174));
#151148=CARTESIAN_POINT('Ctrl Pts',(6.75186776773318,1.74964163128043,-5.95083070747795));
#151149=CARTESIAN_POINT('Ctrl Pts',(6.74566379503783,1.74349822273683,-5.95785940585845));
#151150=CARTESIAN_POINT('Ctrl Pts',(6.73329157831985,1.72630637188949,-5.97184161327271));
#151151=CARTESIAN_POINT('Ctrl Pts',(6.72762793952884,1.71456563933645,-5.97821595182398));
#151152=CARTESIAN_POINT('Ctrl Pts',(6.72220518672269,1.69868853678518,-5.98430946965148));
#151153=CARTESIAN_POINT('Ctrl Pts',(6.72124370078741,1.69560796578166,-5.98538928716462));
#151154=CARTESIAN_POINT('Ctrl Pts',(6.72035024189579,1.69247211204104,-5.98639228803552));
#151155=CARTESIAN_POINT('Ctrl Pts',(6.54445255413051,0.999999999900245,
-6.17819882868257));
#151156=CARTESIAN_POINT('Ctrl Pts',(6.553257800479,1.04120750293032,-6.16887159293748));
#151157=CARTESIAN_POINT('Ctrl Pts',(6.56240790930224,1.08227801709433,-6.15913903849141));
#151158=CARTESIAN_POINT('Ctrl Pts',(6.6160465662733,1.31475831833009,-6.10181211457691));
#151159=CARTESIAN_POINT('Ctrl Pts',(6.66661042504181,1.5038565988065,-6.0467208421714));
#151160=CARTESIAN_POINT('Ctrl Pts',(6.72035024216997,1.69247211186447,-5.98639228772773));
#151161=CARTESIAN_POINT('',(6.281871763,1.69247211199998,-6.445004822));
#151162=CARTESIAN_POINT('Ctrl Pts',(6.28187176315731,1.69247211214928,-6.44500482166204));
#151163=CARTESIAN_POINT('Ctrl Pts',(6.33972854297822,1.50385659908022,-6.38861248658687));
#151164=CARTESIAN_POINT('Ctrl Pts',(6.39249580318891,1.31475831859254,-6.33562788166308));
#151165=CARTESIAN_POINT('Ctrl Pts',(6.44735851345534,1.08227801735199,-6.27947127252895));
#151166=CARTESIAN_POINT('Ctrl Pts',(6.45667074978433,1.04120750319416,-6.26989372785291));
#151167=CARTESIAN_POINT('Ctrl Pts',(6.46559354773797,1.00000000017037,-6.26067888295264));
#151168=CARTESIAN_POINT('',(6.15668002,1.69247211199998,-6.564700384));
#151169=CARTESIAN_POINT('Ctrl Pts',(6.28187176296278,1.69247211203293,-6.44500482185164));
#151170=CARTESIAN_POINT('Ctrl Pts',(6.28034809508384,1.69743933281709,-6.44648992333557));
#151171=CARTESIAN_POINT('Ctrl Pts',(6.27864771881356,1.70224131118791,-6.44814621926316));
#151172=CARTESIAN_POINT('Ctrl Pts',(6.27115368823405,1.72064855735323,-6.45543901695008));
#151173=CARTESIAN_POINT('Ctrl Pts',(6.26412450434272,1.73230722874697,-6.46226527600085));
#151174=CARTESIAN_POINT('Ctrl Pts',(6.25072809411953,1.74686546604395,-6.47521827361668));
#151175=CARTESIAN_POINT('Ctrl Pts',(6.24486763671979,1.75155833711437,-6.48087242061939));
#151176=CARTESIAN_POINT('Ctrl Pts',(6.23238391577944,1.7578101367976,-6.49287776651093));
#151177=CARTESIAN_POINT('Ctrl Pts',(6.22603385296701,1.75940739641221,-6.4989678095005));
#151178=CARTESIAN_POINT('Ctrl Pts',(6.21956384103444,1.75940739641324,-6.50515377430056));
#151179=CARTESIAN_POINT('Ctrl Pts',(6.21246400605725,1.75940739641437,-6.51194191158886));
#151180=CARTESIAN_POINT('Ctrl Pts',(6.20542262069756,1.75748289719422,-6.51865146227563));
#151181=CARTESIAN_POINT('Ctrl Pts',(6.19125838137018,1.74964163157005,-6.53210717281417));
#151182=CARTESIAN_POINT('Ctrl Pts',(6.18444933637955,1.74349822302713,-6.53855145589715));
#151183=CARTESIAN_POINT('Ctrl Pts',(6.17087357116009,1.72630637218225,-6.55136833809903));
#151184=CARTESIAN_POINT('Ctrl Pts',(6.16466134121213,1.71456563963166,-6.55720933076995));
#151185=CARTESIAN_POINT('Ctrl Pts',(6.15871420003383,1.69868853693743,-6.56279222612325));
#151186=CARTESIAN_POINT('Ctrl Pts',(6.15765979061543,1.69560796578235,-6.56378150971813));
#151187=CARTESIAN_POINT('Ctrl Pts',(6.15668002018172,1.69247211188529,-6.56470038380239));
#151188=CARTESIAN_POINT('Ctrl Pts',(5.96429703930701,0.999999999993495,
-6.73996742031544));
#151189=CARTESIAN_POINT('Ctrl Pts',(5.97390292527019,1.04120750293781,-6.73146702949198));
#151190=CARTESIAN_POINT('Ctrl Pts',(5.98388861787979,1.08227801701666,-6.7225938648969));
#151191=CARTESIAN_POINT('Ctrl Pts',(6.04245008719923,1.31475831813608,-6.67030585448667));
#151192=CARTESIAN_POINT('Ctrl Pts',(6.09774873431317,1.50385659858127,-6.61996887270678));
#151193=CARTESIAN_POINT('Ctrl Pts',(6.15668002065362,1.69247211160818,-6.56470038335982));
#151194=CARTESIAN_POINT('',(5.678857015,1.69247211199998,-6.982161771));
#151195=CARTESIAN_POINT('Ctrl Pts',(5.67885701527804,1.69247211202244,-6.98216177125877));
#151196=CARTESIAN_POINT('Ctrl Pts',(5.74153585071579,1.50385659882619,-6.93118269686947));
#151197=CARTESIAN_POINT('Ctrl Pts',(5.79884018886956,1.31475831821191,-6.88314141309411));
#151198=CARTESIAN_POINT('Ctrl Pts',(5.85851587764468,1.08227801691581,-6.83212872938778));
#151199=CARTESIAN_POINT('Ctrl Pts',(5.86864915011615,1.04120750283384,-6.82342448353686));
#151200=CARTESIAN_POINT('Ctrl Pts',(5.87836203982082,0.999999999886374,
-6.81504656835106));
#151201=CARTESIAN_POINT('',(5.54343983025803,1.69247211212479,-7.09015337246984));
#151202=CARTESIAN_POINT('Ctrl Pts',(5.678857014964,1.69247211184902,-6.98216177151419));
#151203=CARTESIAN_POINT('Ctrl Pts',(5.67720635746447,1.6974393325806,-6.98350431387102));
#151204=CARTESIAN_POINT('Ctrl Pts',(5.67536435720178,1.70224131090145,-6.98500152147185));
#151205=CARTESIAN_POINT('Ctrl Pts',(5.66724677406077,1.72064855700609,-6.9915932007598));
#151206=CARTESIAN_POINT('Ctrl Pts',(5.65963398645625,1.73230722838638,-6.9977618881084));
#151207=CARTESIAN_POINT('Ctrl Pts',(5.64513040849172,1.74686546566725,-7.00946189580317));
#151208=CARTESIAN_POINT('Ctrl Pts',(5.63878670974101,1.7515583367325,-7.01456795351954));
#151209=CARTESIAN_POINT('Ctrl Pts',(5.6252770936824,1.75781013640549,-7.02540593729717));
#151210=CARTESIAN_POINT('Ctrl Pts',(5.61840668711161,1.75940739601474,-7.03090224832022));
#151211=CARTESIAN_POINT('Ctrl Pts',(5.61140821593638,1.75940739601077,-7.03648334284404));
#151212=CARTESIAN_POINT('Ctrl Pts',(5.60372847887254,1.75940739600641,-7.04260772878465));
#151213=CARTESIAN_POINT('Ctrl Pts',(5.59611400057448,1.75748289678096,-7.04865908387314));
#151214=CARTESIAN_POINT('Ctrl Pts',(5.58080062171539,1.74964163114593,-7.06079095305036));
#151215=CARTESIAN_POINT('Ctrl Pts',(5.57344132685394,1.74349822259538,-7.0665989352571));
#151216=CARTESIAN_POINT('Ctrl Pts',(5.55877131720443,1.72630637173008,-7.0781472982493));
#151217=CARTESIAN_POINT('Ctrl Pts',(5.55206051331797,1.71456563916439,-7.08340791680299));
#151218=CARTESIAN_POINT('Ctrl Pts',(5.54563686680511,1.69868853671578,-7.08843523935245));
#151219=CARTESIAN_POINT('Ctrl Pts',(5.54449802352356,1.69560796583262,-7.08932602377848));
#151220=CARTESIAN_POINT('Ctrl Pts',(5.54343983019798,1.69247211221631,-7.09015337273987));
#151221=CARTESIAN_POINT('Ctrl Pts',(5.33612051021732,1.00000000003863,-7.24746975850455));
#151222=CARTESIAN_POINT('Ctrl Pts',(5.34644969490054,1.04120750312078,-7.23986465271198));
#151223=CARTESIAN_POINT('Ctrl Pts',(5.35719057242632,1.08227801733654,-7.23192231942854));
#151224=CARTESIAN_POINT('Ctrl Pts',(5.42020335165464,1.3147583185972,-7.1850942147898));
#151225=CARTESIAN_POINT('Ctrl Pts',(5.47979155494116,1.50385659904842,-7.13991680741592));
#151226=CARTESIAN_POINT('Ctrl Pts',(5.54343983044598,1.69247211208145,-7.09015337254597));
#151227=CARTESIAN_POINT('',(5.030119452,1.69247211199998,-7.463102458));
#151228=CARTESIAN_POINT('Ctrl Pts',(5.03011945219447,1.69247211210035,-7.4631024578693));
#151229=CARTESIAN_POINT('Ctrl Pts',(5.09711568993067,1.50385659918751,-7.41794709780783));
#151230=CARTESIAN_POINT('Ctrl Pts',(5.15849572502523,1.31475831885526,-7.37523593545209));
#151231=CARTESIAN_POINT('Ctrl Pts',(5.22250391870522,1.08227801764803,-7.3297779013181));
#151232=CARTESIAN_POINT('Ctrl Pts',(5.23337664023476,1.0412075033625,-7.32201703570375));
#151233=CARTESIAN_POINT('Ctrl Pts',(5.24380141927541,1.00000000021015,-7.31454350422534));
#151234=CARTESIAN_POINT('',(4.885567124,1.69247211199998,-7.558520614));
#151235=CARTESIAN_POINT('Ctrl Pts',(5.03011945218954,1.69247211209782,-7.46310245787263));
#151236=CARTESIAN_POINT('Ctrl Pts',(5.02835509520953,1.69743933274049,-7.46429163173374));
#151237=CARTESIAN_POINT('Ctrl Pts',(5.0263863016777,1.70224131097822,-7.46561769636424));
#151238=CARTESIAN_POINT('Ctrl Pts',(5.01771052400475,1.72064855704178,-7.47145518492247));
#151239=CARTESIAN_POINT('Ctrl Pts',(5.00957542636926,1.7323072284545,-7.47691663393612));
#151240=CARTESIAN_POINT('Ctrl Pts',(4.99408145493216,1.74686546577659,-7.48726945014651));
#151241=CARTESIAN_POINT('Ctrl Pts',(4.98730559056023,1.75155833685605,-7.49178630760795));
#151242=CARTESIAN_POINT('Ctrl Pts',(4.97287885086278,1.75781013655407,-7.50136966821126));
#151243=CARTESIAN_POINT('Ctrl Pts',(4.96554341700395,1.7594073961748,-7.50622799421012));
#151244=CARTESIAN_POINT('Ctrl Pts',(4.95807283415526,1.75940739618001,-7.51115928277464));
#151245=CARTESIAN_POINT('Ctrl Pts',(4.94987502773369,1.75940739618573,-7.51657060741685));
#151246=CARTESIAN_POINT('Ctrl Pts',(4.94174876379916,1.75748289697065,-7.52191504495913));
#151247=CARTESIAN_POINT('Ctrl Pts',(4.92540953973939,1.74964163135777,-7.53262539410137));
#151248=CARTESIAN_POINT('Ctrl Pts',(4.91755924773006,1.7434982228226,-7.53775031297301));
#151249=CARTESIAN_POINT('Ctrl Pts',(4.90191310796274,1.72630637199696,-7.54793717612113));
#151250=CARTESIAN_POINT('Ctrl Pts',(4.89475776159462,1.71456563945896,-7.55257506514705));
#151251=CARTESIAN_POINT('Ctrl Pts',(4.88790932897337,1.69868853680129,-7.55700633800827));
#151252=CARTESIAN_POINT('Ctrl Pts',(4.88669522094921,1.69560796567097,-7.55779145133232));
#151253=CARTESIAN_POINT('Ctrl Pts',(4.88556712453283,1.69247211179938,-7.5585206139617));
#151254=CARTESIAN_POINT('Ctrl Pts',(4.66498067898464,0.999999999967123,
-7.69661972977099));
#151255=CARTESIAN_POINT('Ctrl Pts',(4.67594999777918,1.04120750284047,-7.68997114090538));
#151256=CARTESIAN_POINT('Ctrl Pts',(4.6873595808967,1.08227801684883,-7.68302358599243));
#151257=CARTESIAN_POINT('Ctrl Pts',(4.75431632809316,1.31475831803052,-7.6420324195285));
#151258=CARTESIAN_POINT('Ctrl Pts',(4.81771431840041,1.50385659860426,-7.60237832843866));
#151259=CARTESIAN_POINT('Ctrl Pts',(4.88556712461049,1.69247211175979,-7.55852061391151));
#151260=CARTESIAN_POINT('',(4.340882323,1.69247211199998,-7.883954633));
#151261=CARTESIAN_POINT('Ctrl Pts',(4.34088232282825,1.69247211188109,-7.88395463326351));
#151262=CARTESIAN_POINT('Ctrl Pts',(4.41165654866182,1.50385659901075,-7.84498655187241));
#151263=CARTESIAN_POINT('Ctrl Pts',(4.47661808484275,1.31475831872082,-7.80794939604147));
#151264=CARTESIAN_POINT('Ctrl Pts',(4.54444342707815,1.08227801765357,-7.76841201286517));
#151265=CARTESIAN_POINT('Ctrl Pts',(4.55596805683155,1.04120750346539,-7.76165701347467));
#151266=CARTESIAN_POINT('Ctrl Pts',(4.56702079094976,1.00000000041109,-7.75514803824096));
#151267=CARTESIAN_POINT('',(4.188358703,1.69247211199998,-7.966031093));
#151268=CARTESIAN_POINT('Ctrl Pts',(4.34088232285577,1.69247211189453,-7.88395463324836));
#151269=CARTESIAN_POINT('Ctrl Pts',(4.33901847194056,1.69743933251756,-7.88498086410161));
#151270=CARTESIAN_POINT('Ctrl Pts',(4.33693873668266,1.70224131073673,-7.88612510909012));
#151271=CARTESIAN_POINT('Ctrl Pts',(4.32777461670889,1.72064855678308,-7.8911614069149));
#151272=CARTESIAN_POINT('Ctrl Pts',(4.31918270807021,1.73230722819561,-7.89587164520932));
#151273=CARTESIAN_POINT('Ctrl Pts',(4.30282309151686,1.74686546551823,-7.90479391513174));
#151274=CARTESIAN_POINT('Ctrl Pts',(4.29566961680087,1.75155833659819,-7.90868520525309));
#151275=CARTESIAN_POINT('Ctrl Pts',(4.28044190909277,1.75781013629617,-7.91693678308729));
#151276=CARTESIAN_POINT('Ctrl Pts',(4.27270050854823,1.75940739591638,-7.92111800767207));
#151277=CARTESIAN_POINT('Ctrl Pts',(4.26481796277002,1.75940739592062,-7.92535978643457));
#151278=CARTESIAN_POINT('Ctrl Pts',(4.25616809090658,1.75940739592527,-7.93001448097121));
#151279=CARTESIAN_POINT('Ctrl Pts',(4.24759546923469,1.75748289670936,-7.93460897069477));
#151280=CARTESIAN_POINT('Ctrl Pts',(4.23036195379284,1.74964163109505,-7.94381156636527));
#151281=CARTESIAN_POINT('Ctrl Pts',(4.22208387056526,1.74349822255884,-7.94821215906903));
#151282=CARTESIAN_POINT('Ctrl Pts',(4.20558757418279,1.7263063717299,-7.95695550374436));
#151283=CARTESIAN_POINT('Ctrl Pts',(4.19804529596739,1.71456563918895,-7.96093332168898));
#151284=CARTESIAN_POINT('Ctrl Pts',(4.19082721695448,1.69868853668133,-7.96473286674421));
#151285=CARTESIAN_POINT('Ctrl Pts',(4.18954761961683,1.69560796571051,-7.96540598759677));
#151286=CARTESIAN_POINT('Ctrl Pts',(4.18835870300193,1.69247211200357,-7.96603109302166));
#151287=CARTESIAN_POINT('Ctrl Pts',(3.95628116469446,1.00000000003948,-8.08380104566434));
#151288=CARTESIAN_POINT('Ctrl Pts',(3.96780229915045,1.04120750292555,-8.07816250421748));
#151289=CARTESIAN_POINT('Ctrl Pts',(3.97978872466482,1.08227801694657,-8.0722656652622));
#151290=CARTESIAN_POINT('Ctrl Pts',(4.05015034350906,1.31475831811704,-8.03744147373217));
#151291=CARTESIAN_POINT('Ctrl Pts',(4.11684767745441,1.50385659866781,-8.00362997039905));
#151292=CARTESIAN_POINT('Ctrl Pts',(4.18835870342248,1.69247211180005,-7.96603109280055));
#151293=CARTESIAN_POINT('',(3.61669496163465,1.69247211178013,-8.24132984144472));
#151294=CARTESIAN_POINT('Ctrl Pts',(3.61669496156912,1.69247211175992,-8.24132984141276));
#151295=CARTESIAN_POINT('Ctrl Pts',(3.69067734322808,1.5038565985687,-8.20886278668498));
#151296=CARTESIAN_POINT('Ctrl Pts',(3.75869734856277,1.3147583179601,-8.17779783869765));
#151297=CARTESIAN_POINT('Ctrl Pts',(3.82979374964924,1.08227801680555,-8.14449943819061));
#151298=CARTESIAN_POINT('Ctrl Pts',(3.84187749804066,1.04120750286063,-8.13880469232044));
#151299=CARTESIAN_POINT('Ctrl Pts',(3.85346919708018,1.00000000005117,-8.13331267978517));
#151300=CARTESIAN_POINT('',(3.45742808,1.69247211199998,-8.309403774));
#151301=CARTESIAN_POINT('Ctrl Pts',(3.61669496113721,1.69247211155784,-8.2413298416023));
#151302=CARTESIAN_POINT('Ctrl Pts',(3.61474662287773,1.69743933229287,-8.24218486685928));
#151303=CARTESIAN_POINT('Ctrl Pts',(3.61257269064702,1.702241310617,-8.24313807944231));
#151304=CARTESIAN_POINT('Ctrl Pts',(3.60299401241548,1.72064855672639,-8.24733263725376));
#151305=CARTESIAN_POINT('Ctrl Pts',(3.59401446977581,1.73230722810798,-8.25125374075692));
#151306=CARTESIAN_POINT('Ctrl Pts',(3.57692092613147,1.74686546539134,-8.25867362751413));
#151307=CARTESIAN_POINT('Ctrl Pts',(3.56944743664772,1.75155833645782,-8.26190801991309));
#151308=CARTESIAN_POINT('Ctrl Pts',(3.55354136548705,1.75781013613199,-8.2687613781201));
#151309=CARTESIAN_POINT('Ctrl Pts',(3.54545632746743,1.75940739574123,-8.2722318365261));
#151310=CARTESIAN_POINT('Ctrl Pts',(3.53722528439024,1.75940739573664,-8.27574995317466));
#151311=CARTESIAN_POINT('Ctrl Pts',(3.52819299076564,1.7594073957316,-8.27961054074264));
#151312=CARTESIAN_POINT('Ctrl Pts',(3.51924303306519,1.75748289650574,-8.28341809051765));
#151313=CARTESIAN_POINT('Ctrl Pts',(3.50125398036881,1.74964163087024,-8.29103883882884));
#151314=CARTESIAN_POINT('Ctrl Pts',(3.4926147561768,1.74349822231929,-8.29467967438142));
#151315=CARTESIAN_POINT('Ctrl Pts',(3.47540112164681,1.72630637145232,-8.30190910431719));
#151316=CARTESIAN_POINT('Ctrl Pts',(3.46753263756868,1.71456563888475,-8.30519482413073));
#151317=CARTESIAN_POINT('Ctrl Pts',(3.46000302790207,1.69868853650819,-8.30833204968783));
#151318=CARTESIAN_POINT('Ctrl Pts',(3.45866824382614,1.69560796570203,-8.30888775850462));
#151319=CARTESIAN_POINT('Ctrl Pts',(3.45742807947873,1.69247211216522,-8.30940377375128));
#151320=CARTESIAN_POINT('Ctrl Pts',(3.21572799916628,1.00000000027708,-8.40589634931207));
#151321=CARTESIAN_POINT('Ctrl Pts',(3.22770818794206,1.04120750338201,-8.40131325348497));
#151322=CARTESIAN_POINT('Ctrl Pts',(3.2401749482664,1.08227801762046,-8.39651460834608));
#151323=CARTESIAN_POINT('Ctrl Pts',(3.31337492842116,1.31475831887219,-8.36813777565844));
#151324=CARTESIAN_POINT('Ctrl Pts',(3.3828345982506,1.50385659929336,-8.34044109045194));
#151325=CARTESIAN_POINT('Ctrl Pts',(3.45742807919782,1.69247211229553,-8.30940377386816));
#151326=CARTESIAN_POINT('',(2.8633881,1.69247211199998,-8.532350707));
#151327=CARTESIAN_POINT('Ctrl Pts',(2.86338810042523,1.69247211217985,-8.53235070694725));
#151328=CARTESIAN_POINT('Ctrl Pts',(2.93998297503229,1.50385659913088,-8.50664608461792));
#151329=CARTESIAN_POINT('Ctrl Pts',(3.01051379221962,1.31475831866339,-8.48180346126633));
#151330=CARTESIAN_POINT('Ctrl Pts',(3.08430882573711,1.08227801739708,-8.45501214257094));
#151331=CARTESIAN_POINT('Ctrl Pts',(3.09685440167008,1.04120750319233,-8.45042350089904));
#151332=CARTESIAN_POINT('Ctrl Pts',(3.10889173621482,1.00000000012129,-8.44599266945545));
#151333=CARTESIAN_POINT('',(2.698660279,1.69247211199998,-8.585874021));
#151334=CARTESIAN_POINT('Ctrl Pts',(2.86338809984566,1.69247211191797,-8.53235070714175));
#151335=CARTESIAN_POINT('Ctrl Pts',(2.86137096114923,1.69743933266371,-8.53302764262381));
#151336=CARTESIAN_POINT('Ctrl Pts',(2.85912033521171,1.70224131099841,-8.53378214807124));
#151337=CARTESIAN_POINT('Ctrl Pts',(2.84920422065504,1.72064855713832,-8.53710119373165));
#151338=CARTESIAN_POINT('Ctrl Pts',(2.83990934200035,1.73230722853923,-8.54020159203121));
#151339=CARTESIAN_POINT('Ctrl Pts',(2.82221949840695,1.746865465846,-8.54605935507156));
#151340=CARTESIAN_POINT('Ctrl Pts',(2.81448616629378,1.75155833692005,-8.54861080832647));
#151341=CARTESIAN_POINT('Ctrl Pts',(2.79802979800296,1.7578101366089,-8.55401076770457));
#151342=CARTESIAN_POINT('Ctrl Pts',(2.78966621847435,1.75940739622565,-8.55674251784626));
#151343=CARTESIAN_POINT('Ctrl Pts',(2.78115294960864,1.7594073962279,-8.55950864658031));
#151344=CARTESIAN_POINT('Ctrl Pts',(2.77181095693985,1.75940739623038,-8.56254404400075));
#151345=CARTESIAN_POINT('Ctrl Pts',(2.76255572300506,1.75748289701185,-8.56553399767843));
#151346=CARTESIAN_POINT('Ctrl Pts',(2.74395597033507,1.74964163139145,-8.57151154084734));
#151347=CARTESIAN_POINT('Ctrl Pts',(2.73502516313977,1.74349822285109,-8.57436330538031));
#151348=CARTESIAN_POINT('Ctrl Pts',(2.71723278454769,1.72630637201231,-8.58002061345237));
#151349=CARTESIAN_POINT('Ctrl Pts',(2.70910144702475,1.71456563946542,-8.58258778044829));
#151350=CARTESIAN_POINT('Ctrl Pts',(2.7013209304805,1.69868853681972,-8.58503742749617));
#151351=CARTESIAN_POINT('Ctrl Pts',(2.69994170637387,1.69560796571128,-8.58547125010984));
#151352=CARTESIAN_POINT('Ctrl Pts',(2.69866027920764,1.69247211186233,-8.5858740205891));
#151353=CARTESIAN_POINT('Ctrl Pts',(2.44928368492693,1.00000000003541,-8.66031231715986));
#151354=CARTESIAN_POINT('Ctrl Pts',(2.46162647047221,1.04120750294047,-8.65682156738601));
#151355=CARTESIAN_POINT('Ctrl Pts',(2.47447319045866,1.08227801698034,-8.65315975197741));
#151356=CARTESIAN_POINT('Ctrl Pts',(2.54992216866385,1.31475831816348,-8.63145875170902));
#151357=CARTESIAN_POINT('Ctrl Pts',(2.62158492606628,1.50385659870848,-8.61009988199061));
#151358=CARTESIAN_POINT('Ctrl Pts',(2.69866027926731,1.69247211183557,-8.58587402057035));
#151359=CARTESIAN_POINT('',(2.08702692,1.69247211199998,-8.754674102));
#151360=CARTESIAN_POINT('Ctrl Pts',(2.08702692043405,1.69247211217429,-8.75467410206591));
#151361=CARTESIAN_POINT('Ctrl Pts',(2.1656175912421,1.50385659900165,-8.7359388706045));
#151362=CARTESIAN_POINT('Ctrl Pts',(2.2380913477429,1.31475831841118,-8.71751859004947));
#151363=CARTESIAN_POINT('Ctrl Pts',(2.31399085943843,1.08227801716552,-8.69745006113722));
#151364=CARTESIAN_POINT('Ctrl Pts',(2.32689725319462,1.04120750310917,-8.69400446875687));
#151365=CARTESIAN_POINT('Ctrl Pts',(2.33928330559697,1.00000000018754,-8.69067049289957));
#151366=CARTESIAN_POINT('',(1.918164453,1.69247211199998,-8.793215858));
#151367=CARTESIAN_POINT('Ctrl Pts',(2.08702692043181,1.69247211217334,-8.75467410206644));
#151368=CARTESIAN_POINT('Ctrl Pts',(2.08495722210436,1.69743933294414,-8.75516749748884));
#151369=CARTESIAN_POINT('Ctrl Pts',(2.08264802316623,1.70224131130219,-8.75571722096838));
#151370=CARTESIAN_POINT('Ctrl Pts',(2.0724743109975,1.72064855744848,-8.7581340314743));
#151371=CARTESIAN_POINT('Ctrl Pts',(2.06293893323256,1.73230722883562,-8.76038876198234));
#151372=CARTESIAN_POINT('Ctrl Pts',(2.04479521792301,1.74686546612392,-8.76463723803522));
#151373=CARTESIAN_POINT('Ctrl Pts',(2.03686430742724,1.75155833719122,-8.76648520934269));
#151374=CARTESIAN_POINT('Ctrl Pts',(2.019990139016,1.75781013686931,-8.77038829258981));
#151375=CARTESIAN_POINT('Ctrl Pts',(2.01141535660801,1.75940739648177,-8.77235934001887));
#151376=CARTESIAN_POINT('Ctrl Pts',(2.00268840579558,1.75940739648129,-8.77435120959333));
#151377=CARTESIAN_POINT('Ctrl Pts',(1.99311193031393,1.75940739648077,-8.77653697762989));
#151378=CARTESIAN_POINT('Ctrl Pts',(1.98362593784728,1.75748289725883,-8.77868526185969));
#151379=CARTESIAN_POINT('Ctrl Pts',(1.96456523947057,1.74964163163066,-8.78297147222287));
#151380=CARTESIAN_POINT('Ctrl Pts',(1.95541475487494,1.74349822308499,-8.7850112050058));
#151381=CARTESIAN_POINT('Ctrl Pts',(1.93718688597779,1.72630637223326,-8.78905084189892));
#151382=CARTESIAN_POINT('Ctrl Pts',(1.92885816375222,1.71456563967815,-8.7908787867595));
#151383=CARTESIAN_POINT('Ctrl Pts',(1.92088938462464,1.69868853704811,-8.79262113211972));
#151384=CARTESIAN_POINT('Ctrl Pts',(1.91947682532086,1.69560796596479,-8.79292957559287));
#151385=CARTESIAN_POINT('Ctrl Pts',(1.91816445274598,1.69247211214181,-8.79321585838888));
#151386=CARTESIAN_POINT('Ctrl Pts',(1.66311917827957,0.999999999892245,
-8.84500054261381));
#151387=CARTESIAN_POINT('Ctrl Pts',(1.67572518383153,1.04120750292225,-8.8426302443313));
#151388=CARTESIAN_POINT('Ctrl Pts',(1.6888484293412,1.0822780170862,-8.84013474140826));
#151389=CARTESIAN_POINT('Ctrl Pts',(1.76593893483276,1.31475831833986,-8.82528429724149));
#151390=CARTESIAN_POINT('Ctrl Pts',(1.83922779333879,1.50385659883379,-8.81043521210152));
#151391=CARTESIAN_POINT('Ctrl Pts',(1.91816445327559,1.6924721119096,-8.79321585827335));
#151392=CARTESIAN_POINT('',(1.293862227,1.69247211199998,-8.906510009));
#151393=CARTESIAN_POINT('Ctrl Pts',(1.29386222704835,1.69247211203084,-8.9065100088316));
#151394=CARTESIAN_POINT('Ctrl Pts',(1.37381592810969,1.50385659888228,-8.8948950133268));
#151395=CARTESIAN_POINT('Ctrl Pts',(1.44764910778165,1.31475831831576,-8.88304538485746));
#151396=CARTESIAN_POINT('Ctrl Pts',(1.52504199941119,1.08227801709192,-8.86986122572233));
#151397=CARTESIAN_POINT('Ctrl Pts',(1.53820529634083,1.04120750303301,-8.86758642450121));
#151398=CARTESIAN_POINT('Ctrl Pts',(1.55084034142984,1.0000000001088,-8.86537614742848));
#151399=CARTESIAN_POINT('',(1.12222469370069,1.69247211186443,-8.92975989245308));
#151400=CARTESIAN_POINT('Ctrl Pts',(1.29386222678592,1.69247211191724,-8.90651000886972));
#151401=CARTESIAN_POINT('Ctrl Pts',(1.29175663284455,1.6974393326443,-8.90681589169734));
#151402=CARTESIAN_POINT('Ctrl Pts',(1.28940745324757,1.70224131096108,-8.90715640715206));
#151403=CARTESIAN_POINT('Ctrl Pts',(1.27905805625247,1.72064855707061,-8.90865152375759));
#151404=CARTESIAN_POINT('Ctrl Pts',(1.26935895263178,1.73230722845891,-8.91004243270966));
#151405=CARTESIAN_POINT('Ctrl Pts',(1.25090744812925,1.74686546574982,-8.91264741554434));
#151406=CARTESIAN_POINT('Ctrl Pts',(1.24284281427571,1.75155833681844,-8.91377702612638));
#151407=CARTESIAN_POINT('Ctrl Pts',(1.22568670661819,1.75781013649756,-8.91615180791229));
#151408=CARTESIAN_POINT('Ctrl Pts',(1.21696976043267,1.75940739610974,-8.9173462829144));
#151409=CARTESIAN_POINT('Ctrl Pts',(1.20809939194526,1.75940739610823,-8.91854785596744));
#151410=CARTESIAN_POINT('Ctrl Pts',(1.19836553780406,1.75940739610657,-8.91986639609967));
#151411=CARTESIAN_POINT('Ctrl Pts',(1.18872516244252,1.75748289688384,-8.92115571415885));
#151412=CARTESIAN_POINT('Ctrl Pts',(1.16935698390139,1.74964163125454,-8.92371608166787));
#151413=CARTESIAN_POINT('Ctrl Pts',(1.1600604962301,1.74349822270799,-8.9249273599703));
#151414=CARTESIAN_POINT('Ctrl Pts',(1.14154389711402,1.72630637185311,-8.92731680090106));
#151415=CARTESIAN_POINT('Ctrl Pts',(1.13308484816045,1.71456563929485,-8.92839080608824));
#151416=CARTESIAN_POINT('Ctrl Pts',(1.12499196639287,1.6986885367259,-8.92941182141989));
#151417=CARTESIAN_POINT('Ctrl Pts',(1.12355744500622,1.69560796570946,-8.92959240234685));
#151418=CARTESIAN_POINT('Ctrl Pts',(1.12222469348958,1.69247211195553,-8.92975989247875));
#151419=CARTESIAN_POINT('Ctrl Pts',(0.863564213439779,0.999999999851495,
-8.95847402459069));
#151420=CARTESIAN_POINT('Ctrl Pts',(0.87633194283773,1.04120750294903,-8.95724326205628));
#151421=CARTESIAN_POINT('Ctrl Pts',(0.889626053196569,1.08227801718005,
-8.95593416395052));
#151422=CARTESIAN_POINT('Ctrl Pts',(0.967737398493407,1.31475831834262,
-8.94805384294514));
#151423=CARTESIAN_POINT('Ctrl Pts',(1.04206227925682,1.50385659868299,-8.93983409849226));
#151424=CARTESIAN_POINT('Ctrl Pts',(1.12222469430304,1.69247211160434,-8.92975989237653));
#151425=CARTESIAN_POINT('',(0.490280117,1.69247211199998,-8.986635934));
#151426=CARTESIAN_POINT('Ctrl Pts',(0.490280116634964,1.69247211184778,
-8.98663593383155));
#151427=CARTESIAN_POINT('Ctrl Pts',(0.570953107639295,1.50385659894552,
-8.98223469139443));
#151428=CARTESIAN_POINT('Ctrl Pts',(0.645551249023958,1.31475831862389,
-8.97705112125193));
#151429=CARTESIAN_POINT('Ctrl Pts',(0.723814398508999,1.08227801747435,
-8.97085748298641));
#151430=CARTESIAN_POINT('Ctrl Pts',(0.737128615539833,1.04120750323641,
-8.96977178828106));
#151431=CARTESIAN_POINT('Ctrl Pts',(0.74991092341197,1.00000000013195,-8.9687030058391));
#151432=CARTESIAN_POINT('',(0.317249443000001,1.69247211199998,-8.99440675));
#151433=CARTESIAN_POINT('Ctrl Pts',(0.490280117042473,1.6924721120226,-8.98663593380931));
#151434=CARTESIAN_POINT('Ctrl Pts',(0.488155580485674,1.69743933273218,
-8.98675184125671));
#151435=CARTESIAN_POINT('Ctrl Pts',(0.485785334434538,1.70224131103288,
-8.98688040706054));
#151436=CARTESIAN_POINT('Ctrl Pts',(0.475343579859998,1.72064855714611,
-8.98744179197277));
#151437=CARTESIAN_POINT('Ctrl Pts',(0.465558841857586,1.73230722855128,
-8.98795768059026));
#151438=CARTESIAN_POINT('Ctrl Pts',(0.446948108818821,1.74686546586344,
-8.98889819642084));
#151439=CARTESIAN_POINT('Ctrl Pts',(0.438814683296199,1.75155833693934,
-8.98930035131872));
#151440=CARTESIAN_POINT('Ctrl Pts',(0.421514767281569,1.75781013663147,
-8.99012771129987));
#151441=CARTESIAN_POINT('Ctrl Pts',(0.41272584104224,1.75940739624973,-8.99053599666621));
#151442=CARTESIAN_POINT('Ctrl Pts',(0.403783473868803,1.7594073962532,-8.99093759883976));
#151443=CARTESIAN_POINT('Ctrl Pts',(0.393970612336502,1.75940739625701,
-8.9913782949601));
#151444=CARTESIAN_POINT('Ctrl Pts',(0.384253472711401,1.75748289703986,
-8.99179826602011));
#151445=CARTESIAN_POINT('Ctrl Pts',(0.364733755191164,1.74964163142237,
-8.99261217610549));
#151446=CARTESIAN_POINT('Ctrl Pts',(0.355366114298915,1.74349822288405,
-8.99298524742859));
#151447=CARTESIAN_POINT('Ctrl Pts',(0.336709869740617,1.7263063720505,-8.99370525402671));
#151448=CARTESIAN_POINT('Ctrl Pts',(0.328188601351915,1.71456563950727,
-8.99401667228355));
#151449=CARTESIAN_POINT('Ctrl Pts',(0.320036776042563,1.69868853696225,
-8.99430813697986));
#151450=CARTESIAN_POINT('Ctrl Pts',(0.318591842470323,1.69560796595495,
-8.99435940143549));
#151451=CARTESIAN_POINT('Ctrl Pts',(0.317249442521872,1.69247211221038,
-8.99440675037657));
#151452=CARTESIAN_POINT('Ctrl Pts',(0.0570563382849732,0.999999999911668,
-8.99981914119731));
#151453=CARTESIAN_POINT('Ctrl Pts',(0.069882993212187,1.04120750284218,
-8.99973782378958));
#151454=CARTESIAN_POINT('Ctrl Pts',(0.0832409319874684,1.08227801690732,
-8.99962567059221));
#151455=CARTESIAN_POINT('Ctrl Pts',(0.161744210525078,1.31475831815755,
-8.99877892044582));
#151456=CARTESIAN_POINT('Ctrl Pts',(0.236506693492214,1.50385659874335,
-8.99725469720449));
#151457=CARTESIAN_POINT('Ctrl Pts',(0.317249443220438,1.69247211191093,
-8.99440675035193));
#151458=CARTESIAN_POINT('',(-0.317249441999998,1.69247211199998,-8.99440675));
#151459=CARTESIAN_POINT('Ctrl Pts',(-0.3172494417691,1.69247211210491,-8.99440675040312));
#151460=CARTESIAN_POINT('Ctrl Pts',(-0.236506691980428,1.50385659883905,
-8.99725469724477));
#151461=CARTESIAN_POINT('Ctrl Pts',(-0.161744208956718,1.3147583181561,
-8.99877892047434));
#151462=CARTESIAN_POINT('Ctrl Pts',(-0.0832409304009231,1.08227801689511,
-8.99962567060685));
#151463=CARTESIAN_POINT('Ctrl Pts',(-0.0698829916511323,1.0412075029195,
-8.99973782380167));
#151464=CARTESIAN_POINT('Ctrl Pts',(-0.0570563367470325,1.00000000007913,
-8.99981914120706));
#151465=CARTESIAN_POINT('',(-0.490280117,1.69247211199998,-8.986635934));
#151466=CARTESIAN_POINT('Ctrl Pts',(-0.317249442367008,1.69247211184862,
-8.99440675038203));
#151467=CARTESIAN_POINT('Ctrl Pts',(-0.319375816065643,1.69743933266917,
-8.99433174922977));
#151468=CARTESIAN_POINT('Ctrl Pts',(-0.32174804480143,1.70224131107396,
-8.99424733024544));
#151469=CARTESIAN_POINT('Ctrl Pts',(-0.332198086155421,1.72064855725429,
-8.99387046351945));
#151470=CARTESIAN_POINT('Ctrl Pts',(-0.341989677572707,1.7323072286332,
-8.9935071781673));
#151471=CARTESIAN_POINT('Ctrl Pts',(-0.360609796449266,1.74686546591158,
-8.99277565450731));
#151472=CARTESIAN_POINT('Ctrl Pts',(-0.368746528075211,1.75155833697566,
-8.99244711580377));
#151473=CARTESIAN_POINT('Ctrl Pts',(-0.386050963682256,1.75781013664746,
-8.99172039255882));
#151474=CARTESIAN_POINT('Ctrl Pts',(-0.394841106701602,1.75940739625667,
-8.99133920101302));
#151475=CARTESIAN_POINT('Ctrl Pts',(-0.4037834738688,1.7594073962532,-8.99093759883976));
#151476=CARTESIAN_POINT('Ctrl Pts',(-0.413596335402218,1.75940739624939,
-8.99049690271936));
#151477=CARTESIAN_POINT('Ctrl Pts',(-0.423312002595473,1.75748289702424,
-8.99004414541729));
#151478=CARTESIAN_POINT('Ctrl Pts',(-0.442826097813949,1.74964163138952,
-8.98910504494811));
#151479=CARTESIAN_POINT('Ctrl Pts',(-0.452189469197941,1.74349822283924,
-8.98863690553838));
#151480=CARTESIAN_POINT('Ctrl Pts',(-0.47083515010459,1.72630637197522,
-8.98768168072916));
#151481=CARTESIAN_POINT('Ctrl Pts',(-0.479350029693784,1.71456563941106,
-8.98722800469669));
#151482=CARTESIAN_POINT('Ctrl Pts',(-0.487495164855626,1.69868853682224,
-8.98678757205289));
#151483=CARTESIAN_POINT('Ctrl Pts',(-0.488938876868527,1.69560796579138,
-8.98670910728539));
#151484=CARTESIAN_POINT('Ctrl Pts',(-0.490280117042473,1.6924721120226,
-8.98663593380931));
#151485=CARTESIAN_POINT('Ctrl Pts',(-0.749910923055967,1.00000000002074,
-8.96870300586887));
#151486=CARTESIAN_POINT('Ctrl Pts',(-0.73712861517006,1.04120750317642,
-8.96977178831146));
#151487=CARTESIAN_POINT('Ctrl Pts',(-0.723814398124092,1.08227801746521,
-8.97085748301749));
#151488=CARTESIAN_POINT('Ctrl Pts',(-0.645551248646323,1.31475831860558,
-8.97705112127892));
#151489=CARTESIAN_POINT('Ctrl Pts',(-0.570953107291633,1.503856598869,-8.98223469141623));
#151490=CARTESIAN_POINT('Ctrl Pts',(-0.490280116319863,1.69247211171261,
-8.98663593384873));
#151491=CARTESIAN_POINT('',(-1.122224693,1.69247211199998,-8.929759892));
#151492=CARTESIAN_POINT('Ctrl Pts',(-1.12222469326036,1.69247211191644,
-8.92975989250756));
#151493=CARTESIAN_POINT('Ctrl Pts',(-1.04206227819181,1.50385659894457,
-8.9398340986166));
#151494=CARTESIAN_POINT('Ctrl Pts',(-0.967737397408281,1.31475831855362,
-8.9480538430626));
#151495=CARTESIAN_POINT('Ctrl Pts',(-0.889626052114516,1.08227801739532,
-8.95593416405797));
#151496=CARTESIAN_POINT('Ctrl Pts',(-0.876331941773366,1.04120750322035,
-8.95724326216039));
#151497=CARTESIAN_POINT('Ctrl Pts',(-0.863564212391512,1.00000000017931,
-8.95847402469174));
#151498=CARTESIAN_POINT('',(-1.293862227,1.69247211199998,-8.906510009));
#151499=CARTESIAN_POINT('Ctrl Pts',(-1.12222469343999,1.69247211183886,
-8.92975989248499));
#151500=CARTESIAN_POINT('Ctrl Pts',(-1.12433578390216,1.69743933257241,
-8.92949458660048));
#151501=CARTESIAN_POINT('Ctrl Pts',(-1.12669089544509,1.70224131089559,
-8.92919786252279));
#151502=CARTESIAN_POINT('Ctrl Pts',(-1.13706508588636,1.72064855702356,
-8.9278857784736));
#151503=CARTESIAN_POINT('Ctrl Pts',(-1.1467846945914,1.73230722842328,-8.92664624411453));
#151504=CARTESIAN_POINT('Ctrl Pts',(-1.16526428107703,1.74686546572887,
-8.92424857076721));
#151505=CARTESIAN_POINT('Ctrl Pts',(-1.17333880663464,1.75155833680263,
-8.92319198366484));
#151506=CARTESIAN_POINT('Ctrl Pts',(-1.19050843670974,1.7578101364906,-8.92091702834642));
#151507=CARTESIAN_POINT('Ctrl Pts',(-1.19922902345514,1.75940739610672,
-8.91974942902085));
#151508=CARTESIAN_POINT('Ctrl Pts',(-1.20809939194526,1.75940739610823,
-8.91854785596744));
#151509=CARTESIAN_POINT('Ctrl Pts',(-1.21783324608597,1.75940739610989,
-8.91722931583528));
#151510=CARTESIAN_POINT('Ctrl Pts',(-1.22746921600719,1.75748289689063,
-8.91590747550959));
#151511=CARTESIAN_POINT('Ctrl Pts',(-1.24682057289392,1.74964163126884,
-8.91322292557665));
#151512=CARTESIAN_POINT('Ctrl Pts',(-1.25610428640085,1.74349822272748,
-8.91191734462038));
#151513=CARTESIAN_POINT('Ctrl Pts',(-1.27458927957878,1.72630637188588,
-8.90929457931835));
#151514=CARTESIAN_POINT('Ctrl Pts',(-1.28302921355709,1.71456563933674,
-8.90807946173197));
#151515=CARTESIAN_POINT('Ctrl Pts',(-1.29110207873021,1.69868853674836,
-8.90691067785349));
#151516=CARTESIAN_POINT('Ctrl Pts',(-1.29253294526348,1.69560796570205,
-8.906703115614));
#151517=CARTESIAN_POINT('Ctrl Pts',(-1.29386222678592,1.69247211191724,
-8.90651000886972));
#151518=CARTESIAN_POINT('Ctrl Pts',(-1.5508403410948,1.00000000000292,-8.86537614748708));
#151519=CARTESIAN_POINT('Ctrl Pts',(-1.53820529599185,1.04120750297962,
-8.86758642456176));
#151520=CARTESIAN_POINT('Ctrl Pts',(-1.52504199904687,1.08227801709064,
-8.869861225785));
#151521=CARTESIAN_POINT('Ctrl Pts',(-1.44764910742439,1.31475831830606,
-8.88304538491551));
#151522=CARTESIAN_POINT('Ctrl Pts',(-1.37381592778245,1.50385659881392,
-8.89489501337705));
#151523=CARTESIAN_POINT('Ctrl Pts',(-1.29386222675377,1.69247211190334,
-8.90651000887439));
#151524=CARTESIAN_POINT('',(-1.918164453,1.69247211199998,-8.793215858));
#151525=CARTESIAN_POINT('Ctrl Pts',(-1.91816445274452,1.69247211214243,
-8.7932158583892));
#151526=CARTESIAN_POINT('Ctrl Pts',(-1.8392277928231,1.50385659907754,-8.81043521220902));
#151527=CARTESIAN_POINT('Ctrl Pts',(-1.76593893433233,1.31475831859373,
-8.82528429734153));
#151528=CARTESIAN_POINT('Ctrl Pts',(-1.68884842884387,1.08227801731721,
-8.84013474150328));
#151529=CARTESIAN_POINT('Ctrl Pts',(-1.67572518332552,1.04120750311924,
-8.84263024442721));
#151530=CARTESIAN_POINT('Ctrl Pts',(-1.66311917776566,1.00000000005502,
-8.84500054271044));
#151531=CARTESIAN_POINT('',(-2.08702692,1.69247211199998,-8.754674102));
#151532=CARTESIAN_POINT('Ctrl Pts',(-1.91816445274599,1.69247211214183,
-8.79321585838888));
#151533=CARTESIAN_POINT('Ctrl Pts',(-1.92024326275654,1.69743933291711,
-8.79276238385459));
#151534=CARTESIAN_POINT('Ctrl Pts',(-1.92256229518958,1.70224131127948,
-8.7922557437256));
#151535=CARTESIAN_POINT('Ctrl Pts',(-1.93277710790523,1.72064855743359,
-8.79001900647378));
#151536=CARTESIAN_POINT('Ctrl Pts',(-1.94234647731931,1.73230722882437,
-8.78791320310792));
#151537=CARTESIAN_POINT('Ctrl Pts',(-1.96053674463813,1.74686546611736,
-8.78386868472646));
#151538=CARTESIAN_POINT('Ctrl Pts',(-1.96848405279003,1.75155833718626,
-8.7820925562423));
#151539=CARTESIAN_POINT('Ctrl Pts',(-1.9853806375546,1.75781013686712,-8.77828768545104));
#151540=CARTESIAN_POINT('Ctrl Pts',(-1.99396145498231,1.75940739648082,
-8.77634307916798));
#151541=CARTESIAN_POINT('Ctrl Pts',(-2.00268840579558,1.75940739648129,
-8.77435120959333));
#151542=CARTESIAN_POINT('Ctrl Pts',(-2.0122648812771,1.75940739648181,-8.7721654415568));
#151543=CARTESIAN_POINT('Ctrl Pts',(-2.02174357076493,1.75748289726095,
-8.76998516088618));
#151544=CARTESIAN_POINT('Ctrl Pts',(-2.04077638358099,1.74964163163514,
-8.76557677590213));
#151545=CARTESIAN_POINT('Ctrl Pts',(-2.04990569221385,1.74349822309111,
-8.76344426516706));
#151546=CARTESIAN_POINT('Ctrl Pts',(-2.06808116737671,1.72630637224354,
-8.75917507633169));
#151547=CARTESIAN_POINT('Ctrl Pts',(-2.07637820236166,1.71456563969127,
-8.75720830060181));
#151548=CARTESIAN_POINT('Ctrl Pts',(-2.08431379958806,1.69868853706913,
-8.75532057584465));
#151549=CARTESIAN_POINT('Ctrl Pts',(-2.08572030015037,1.69560796599098,
-8.7549855872994));
#151550=CARTESIAN_POINT('Ctrl Pts',(-2.08702692043181,1.69247211217333,
-8.75467410206644));
#151551=CARTESIAN_POINT('Ctrl Pts',(-2.33928330456152,0.99999999985376,
-8.69067049317829));
#151552=CARTESIAN_POINT('Ctrl Pts',(-2.32689725212172,1.04120750291753,
-8.69400446904408));
#151553=CARTESIAN_POINT('Ctrl Pts',(-2.31399085832435,1.08227801711502,
-8.6974500614337));
#151554=CARTESIAN_POINT('Ctrl Pts',(-2.23809134664659,1.31475831833215,
-8.71751859033044));
#151555=CARTESIAN_POINT('Ctrl Pts',(-2.1656175902253,1.50385659875801,-8.73593887085572));
#151556=CARTESIAN_POINT('Ctrl Pts',(-2.08702691950424,1.69247211176485,
-8.75467410228756));
#151557=CARTESIAN_POINT('',(-2.698660279,1.69247211199998,-8.585874021));
#151558=CARTESIAN_POINT('Ctrl Pts',(-2.69866027953189,1.69247211171677,
-8.58587402048719));
#151559=CARTESIAN_POINT('Ctrl Pts',(-2.62158492637212,1.50385659866213,
-8.61009988189709));
#151560=CARTESIAN_POINT('Ctrl Pts',(-2.54992216900827,1.3147583181889,-8.63145875160704));
#151561=CARTESIAN_POINT('Ctrl Pts',(-2.47447319081348,1.0822780170125,-8.65315975187598));
#151562=CARTESIAN_POINT('Ctrl Pts',(-2.46162647080814,1.04120750290523,
-8.65682156729051));
#151563=CARTESIAN_POINT('Ctrl Pts',(-2.44928368524565,0.999999999932309,
-8.66031231706972));
#151564=CARTESIAN_POINT('',(-2.8633881,1.69247211199998,-8.532350707));
#151565=CARTESIAN_POINT('Ctrl Pts',(-2.69866027920764,1.69247211186232,
-8.5858740205891));
#151566=CARTESIAN_POINT('Ctrl Pts',(-2.70069007140367,1.69743933265977,
-8.58523602851499));
#151567=CARTESIAN_POINT('Ctrl Pts',(-2.70295435323217,1.70224131104289,
-8.58452355150266));
#151568=CARTESIAN_POINT('Ctrl Pts',(-2.71292754454375,1.72064855720862,
-8.5813801699417));
#151569=CARTESIAN_POINT('Ctrl Pts',(-2.72226962772906,1.73230722859247,
-8.57842505226088));
#151570=CARTESIAN_POINT('Ctrl Pts',(-2.74002411854314,1.74686546587731,
-8.57276625293122));
#151571=CARTESIAN_POINT('Ctrl Pts',(-2.74778022223851,1.75155833694367,
-8.5702848834079));
#151572=CARTESIAN_POINT('Ctrl Pts',(-2.76426772033127,1.7578101366193,-8.56498073172688));
#151573=CARTESIAN_POINT('Ctrl Pts',(-2.77263968074679,1.75940739623016,
-8.56227477531311));
#151574=CARTESIAN_POINT('Ctrl Pts',(-2.78115294960864,1.7594073962279,-8.55950864658031));
#151575=CARTESIAN_POINT('Ctrl Pts',(-2.79049494227812,1.75940739622543,
-8.55647324915965));
#151576=CARTESIAN_POINT('Ctrl Pts',(-2.79974003449488,1.7574828970017,-8.5534520824834));
#151577=CARTESIAN_POINT('Ctrl Pts',(-2.81830106221837,1.74964163137009,
-8.54735535617395));
#151578=CARTESIAN_POINT('Ctrl Pts',(-2.82720246215093,1.74349822282197,
-8.54441308538321));
#151579=CARTESIAN_POINT('Ctrl Pts',(-2.8449220810608,1.72630637196336,-8.53853184601318));
#151580=CARTESIAN_POINT('Ctrl Pts',(-2.8530094142069,1.71456563940285,-8.53582924746147));
#151581=CARTESIAN_POINT('Ctrl Pts',(-2.86074385070298,1.69868853678566,
-8.53323778068014));
#151582=CARTESIAN_POINT('Ctrl Pts',(-2.86211466095963,1.69560796572133,
-8.53277806296399));
#151583=CARTESIAN_POINT('Ctrl Pts',(-2.86338809984565,1.69247211191798,
-8.53235070714175));
#151584=CARTESIAN_POINT('Ctrl Pts',(-3.10889173543709,1.00000000015543,
-8.44599266974172));
#151585=CARTESIAN_POINT('Ctrl Pts',(-3.09685440089955,1.04120750319919,
-8.45042350118141));
#151586=CARTESIAN_POINT('Ctrl Pts',(-3.08430882497445,1.08227801737684,
-8.45501214284914));
#151587=CARTESIAN_POINT('Ctrl Pts',(-3.01051379149162,1.31475831853189,
-8.4818034615245));
#151588=CARTESIAN_POINT('Ctrl Pts',(-2.93998297433824,1.50385659891702,
-8.5066460848574));
#151589=CARTESIAN_POINT('Ctrl Pts',(-2.86338809976883,1.69247211188328,
-8.53235070716753));
#151590=CARTESIAN_POINT('',(-3.45742808,1.69247211199998,-8.309403774));
#151591=CARTESIAN_POINT('Ctrl Pts',(-3.45742807951293,1.69247211214934,
-8.30940377373705));
#151592=CARTESIAN_POINT('Ctrl Pts',(-3.38283459860251,1.50385659921542,
-8.34044109030884));
#151593=CARTESIAN_POINT('Ctrl Pts',(-3.31337492880746,1.31475831886194,
-8.36813777550526));
#151594=CARTESIAN_POINT('Ctrl Pts',(-3.24017494866242,1.08227801761983,
-8.39651460819328));
#151595=CARTESIAN_POINT('Ctrl Pts',(-3.22770818832162,1.04120750332116,
-8.40131325333917));
#151596=CARTESIAN_POINT('Ctrl Pts',(-3.21572799953086,1.00000000015557,
-8.4058963491726));
#151597=CARTESIAN_POINT('',(-3.616694961,1.69247211199998,-8.241329842));
#151598=CARTESIAN_POINT('Ctrl Pts',(-3.45742807947874,1.69247211216523,
-8.30940377375127));
#151599=CARTESIAN_POINT('Ctrl Pts',(-3.45939251105716,1.69743933261943,
-8.30858640091872));
#151600=CARTESIAN_POINT('Ctrl Pts',(-3.46158381147326,1.70224131067939,
-8.30767382352641));
#151601=CARTESIAN_POINT('Ctrl Pts',(-3.47123508293639,1.72064855658343,
-8.30364910638717));
#151602=CARTESIAN_POINT('Ctrl Pts',(-3.48027466293968,1.73230722799974,
-8.29986846725979));
#151603=CARTESIAN_POINT('Ctrl Pts',(-3.49745042854421,1.74686546532774,
-8.29264094830292));
#151604=CARTESIAN_POINT('Ctrl Pts',(-3.50495288020258,1.75155833640983,
-8.28947431626728));
#151605=CARTESIAN_POINT('Ctrl Pts',(-3.52089854399714,1.75781013611086,
-8.28271358960317));
#151606=CARTESIAN_POINT('Ctrl Pts',(-3.52899424130546,1.75940739573205,
-8.27926806982646));
#151607=CARTESIAN_POINT('Ctrl Pts',(-3.53722528439024,1.75940739573664,
-8.27574995317466));
#151608=CARTESIAN_POINT('Ctrl Pts',(-3.54625757801348,1.75940739574168,
-8.27188936560725));
#151609=CARTESIAN_POINT('Ctrl Pts',(-3.5551946369119,1.75748289652637,-8.26805163758463));
#151610=CARTESIAN_POINT('Ctrl Pts',(-3.57313443705391,1.74964163091365,
-8.26031565721045));
#151611=CARTESIAN_POINT('Ctrl Pts',(-3.58173625944174,1.74349822237848,
-8.25658731580187));
#151612=CARTESIAN_POINT('Ctrl Pts',(-3.598857354133,1.72630637155178,-8.24914137818544));
#151613=CARTESIAN_POINT('Ctrl Pts',(-3.60666987098363,1.71456563901188,
-8.24572471654922));
#151614=CARTESIAN_POINT('Ctrl Pts',(-3.61414087354956,1.6986885365718,-8.24245037274111));
#151615=CARTESIAN_POINT('Ctrl Pts',(-3.61546495648722,1.69560796567022,
-8.24186962725644));
#151616=CARTESIAN_POINT('Ctrl Pts',(-3.61669496095015,1.69247211203475,
-8.2413298416844));
#151617=CARTESIAN_POINT('Ctrl Pts',(-3.85346919584841,0.999999999908194,
-8.13331268036876));
#151618=CARTESIAN_POINT('Ctrl Pts',(-3.84187749678661,1.04120750281033,
-8.13880469291244));
#151619=CARTESIAN_POINT('Ctrl Pts',(-3.82979374837063,1.08227801684729,
-8.14449943879189));
#151620=CARTESIAN_POINT('Ctrl Pts',(-3.75869734727944,1.31475831804488,
-8.17779783928727));
#151621=CARTESIAN_POINT('Ctrl Pts',(-3.69067734197139,1.50385659860643,
-8.20886278724963));
#151622=CARTESIAN_POINT('Ctrl Pts',(-3.61669496034055,1.6924721117496,-8.24132984195192));
#151623=CARTESIAN_POINT('',(-4.188358703,1.69247211199998,-7.966031093));
#151624=CARTESIAN_POINT('Ctrl Pts',(-4.18835870309451,1.69247211195876,
-7.96603109297299));
#151625=CARTESIAN_POINT('Ctrl Pts',(-4.11684767709351,1.50385659876227,
-8.00362997058504));
#151626=CARTESIAN_POINT('Ctrl Pts',(-4.05015034311738,1.31475831814771,
-8.03744147392975));
#151627=CARTESIAN_POINT('Ctrl Pts',(-3.97978872423843,1.08227801688172,
-8.07226566547243));
#151628=CARTESIAN_POINT('Ctrl Pts',(-3.96780229871458,1.04120750283049,
-8.07816250443158));
#151629=CARTESIAN_POINT('Ctrl Pts',(-3.95628116424985,0.999999999913972,
-8.08380104588193));
#151630=CARTESIAN_POINT('',(-4.340882323,1.69247211199998,-7.883954633));
#151631=CARTESIAN_POINT('Ctrl Pts',(-4.18835870300193,1.69247211200357,
-7.96603109302167));
#151632=CARTESIAN_POINT('Ctrl Pts',(-4.19024195767692,1.69743933264773,
-7.96504092037284));
#151633=CARTESIAN_POINT('Ctrl Pts',(-4.19234263382752,1.70224131088609,
-7.96393559005548));
#151634=CARTESIAN_POINT('Ctrl Pts',(-4.2015942793333,1.72064855691523,-7.95906194189281));
#151635=CARTESIAN_POINT('Ctrl Pts',(-4.21025857475973,1.73230722829565,
-7.95448622080491));
#151636=CARTESIAN_POINT('Ctrl Pts',(-4.2267173259628,1.74686546557695,-7.94574817396073));
#151637=CARTESIAN_POINT('Ctrl Pts',(-4.23390572024391,1.75155833664249,
-7.94192177527461));
#151638=CARTESIAN_POINT('Ctrl Pts',(-4.24918116460585,1.75781013631568,
-7.93375890702995));
#151639=CARTESIAN_POINT('Ctrl Pts',(-4.25693541699852,1.75940739592486,
-7.92960156519345));
#151640=CARTESIAN_POINT('Ctrl Pts',(-4.26481796277002,1.75940739592062,
-7.92535978643457));
#151641=CARTESIAN_POINT('Ctrl Pts',(-4.27346783463465,1.75940739591597,
-7.92070509189728));
#151642=CARTESIAN_POINT('Ctrl Pts',(-4.28202490427399,1.75748289669032,
-7.91608170165457));
#151643=CARTESIAN_POINT('Ctrl Pts',(-4.29919903612613,1.74964163105498,
-7.90676875277056));
#151644=CARTESIAN_POINT('Ctrl Pts',(-4.30743202416365,1.7434982225042,-7.90228435915018));
#151645=CARTESIAN_POINT('Ctrl Pts',(-4.32381674566996,1.72630637163808,
-7.89333367358511));
#151646=CARTESIAN_POINT('Ctrl Pts',(-4.3312915444412,1.71456563907159,-7.88923045780918));
#151647=CARTESIAN_POINT('Ctrl Pts',(-4.33843896105432,1.69868853654903,
-7.88529960002584));
#151648=CARTESIAN_POINT('Ctrl Pts',(-4.3397056560187,1.69560796558959,-7.88460250256148));
#151649=CARTESIAN_POINT('Ctrl Pts',(-4.34088232285577,1.69247211189454,
-7.88395463324836));
#151650=CARTESIAN_POINT('Ctrl Pts',(-4.56702079088811,0.999999999926176,
-7.75514803827726));
#151651=CARTESIAN_POINT('Ctrl Pts',(-4.55596805673791,1.04120750310877,
-7.7616570135297));
#151652=CARTESIAN_POINT('Ctrl Pts',(-4.54444342694939,1.08227801742429,
-7.76841201294057));
#151653=CARTESIAN_POINT('Ctrl Pts',(-4.47661808467103,1.31475831862242,
-7.80794939613996));
#151654=CARTESIAN_POINT('Ctrl Pts',(-4.41165654848376,1.50385659891625,
-7.84498655197261));
#151655=CARTESIAN_POINT('Ctrl Pts',(-4.34088232264358,1.69247211179079,
-7.88395463336519));
#151656=CARTESIAN_POINT('',(-4.885567124,1.69247211199998,-7.558520614));
#151657=CARTESIAN_POINT('Ctrl Pts',(-4.88556712448748,1.69247211182252,
-7.55852061399101));
#151658=CARTESIAN_POINT('Ctrl Pts',(-4.81771431823801,1.50385659859261,
-7.60237832854206));
#151659=CARTESIAN_POINT('Ctrl Pts',(-4.75431632789337,1.31475831794536,
-7.64203241965308));
#151660=CARTESIAN_POINT('Ctrl Pts',(-4.6873595806634,1.08227801668198,-7.68302358613477));
#151661=CARTESIAN_POINT('Ctrl Pts',(-4.67594999754258,1.0412075026676,-7.68997114104925));
#151662=CARTESIAN_POINT('Ctrl Pts',(-4.66498067874495,0.999999999788168,
-7.69661972991626));
#151663=CARTESIAN_POINT('',(-5.030119452,1.69247211199998,-7.463102458));
#151664=CARTESIAN_POINT('Ctrl Pts',(-4.88556712453282,1.69247211179936,
-7.55852061396171));
#151665=CARTESIAN_POINT('Ctrl Pts',(-4.8873540394334,1.69743933262183,-7.55736561377867));
#151666=CARTESIAN_POINT('Ctrl Pts',(-4.88934717789494,1.7022413110283,-7.55607642999801));
#151667=CARTESIAN_POINT('Ctrl Pts',(-4.89812470861776,1.72064855720425,
-7.55039309055105));
#151668=CARTESIAN_POINT('Ctrl Pts',(-4.90634395966117,1.7323072285775,-7.54505912851645));
#151669=CARTESIAN_POINT('Ctrl Pts',(-4.92195318028781,1.74686546584881,
-7.53488090739656));
#151670=CARTESIAN_POINT('Ctrl Pts',(-4.92876964047148,1.75155833691055,
-7.53042554997138));
#151671=CARTESIAN_POINT('Ctrl Pts',(-4.94325187651329,1.75781013657807,
-7.52092626275953));
#151672=CARTESIAN_POINT('Ctrl Pts',(-4.95060225131441,1.75940739618522,
-7.51609057133398));
#151673=CARTESIAN_POINT('Ctrl Pts',(-4.95807283415526,1.75940739618001,
-7.51115928277463));
#151674=CARTESIAN_POINT('Ctrl Pts',(-4.96627064057824,1.75940739617429,
-7.50574795813149));
#151675=CARTESIAN_POINT('Ctrl Pts',(-4.97437882446556,1.75748289694722,
-7.5003761304885));
#151676=CARTESIAN_POINT('Ctrl Pts',(-4.99064901201181,1.74964163130847,
-7.48956119548551));
#151677=CARTESIAN_POINT('Ctrl Pts',(-4.99844687851583,1.74349822275537,
-7.48435685535607));
#151678=CARTESIAN_POINT('Ctrl Pts',(-5.01396330668297,1.726306371884,-7.47397348750484));
#151679=CARTESIAN_POINT('Ctrl Pts',(-5.02104020468543,1.71456563931459,
-7.46921675427245));
#151680=CARTESIAN_POINT('Ctrl Pts',(-5.02780648852956,1.69868853677723,
-7.46466103147771));
#151681=CARTESIAN_POINT('Ctrl Pts',(-5.02900559682142,1.6956079658055,-7.4638531946588));
#151682=CARTESIAN_POINT('Ctrl Pts',(-5.03011945218954,1.69247211209781,
-7.46310245787262));
#151683=CARTESIAN_POINT('Ctrl Pts',(-5.24380141833698,1.00000000010371,
-7.31454350489811));
#151684=CARTESIAN_POINT('Ctrl Pts',(-5.23337663930275,1.04120750322152,
-7.32201703636988));
#151685=CARTESIAN_POINT('Ctrl Pts',(-5.2225039177803,1.08227801747272,-7.32977790197709));
#151686=CARTESIAN_POINT('Ctrl Pts',(-5.15849572412172,1.31475831856601,
-7.37523593608384));
#151687=CARTESIAN_POINT('Ctrl Pts',(-5.09711568904592,1.50385659881995,
-7.41794709841542));
#151688=CARTESIAN_POINT('Ctrl Pts',(-5.03011945133157,1.69247211165461,
-7.46310245845089));
#151689=CARTESIAN_POINT('',(-5.54343983057961,1.69247211214186,-7.09015337246368));
#151690=CARTESIAN_POINT('Ctrl Pts',(-5.54343983074268,1.69247211204734,
-7.09015337231399));
#151691=CARTESIAN_POINT('Ctrl Pts',(-5.47979155526345,1.50385659906037,
-7.13991680716822));
#151692=CARTESIAN_POINT('Ctrl Pts',(-5.42020335200143,1.31475831865458,
-7.185094214528));
#151693=CARTESIAN_POINT('Ctrl Pts',(-5.35719057279498,1.08227801744158,
-7.23192231915544));
#151694=CARTESIAN_POINT('Ctrl Pts',(-5.34644969527096,1.0412075032267,-7.23986465243842));
#151695=CARTESIAN_POINT('Ctrl Pts',(-5.33612051058942,1.00000000014546,
-7.24746975823059));
#151696=CARTESIAN_POINT('',(-5.678857015,1.69247211099998,-6.982161771));
#151697=CARTESIAN_POINT('Ctrl Pts',(-5.54343983023425,1.69247211232382,
-7.09015337271151));
#151698=CARTESIAN_POINT('Ctrl Pts',(-5.54511601804185,1.69743933283043,
-7.08884284446661));
#151699=CARTESIAN_POINT('Ctrl Pts',(-5.54698557106644,1.7022413109397,-7.08738018708892));
#151700=CARTESIAN_POINT('Ctrl Pts',(-5.55521831528555,1.72064855688249,
-7.08093291540944));
#151701=CARTESIAN_POINT('Ctrl Pts',(-5.56292634537752,1.73230722829277,
-7.07488365835213));
#151702=CARTESIAN_POINT('Ctrl Pts',(-5.57756035917907,1.74686546561218,
-7.06334721200287));
#151703=CARTESIAN_POINT('Ctrl Pts',(-5.58395000314327,1.75155833669096,
-7.05829876775499));
#151704=CARTESIAN_POINT('Ctrl Pts',(-5.59752242843277,1.7578101363872,-7.04753954424595));
#151705=CARTESIAN_POINT('Ctrl Pts',(-5.60440974475557,1.7594073960068,-7.04206443737231));
#151706=CARTESIAN_POINT('Ctrl Pts',(-5.61140821593638,1.75940739601077,
-7.03648334284404));
#151707=CARTESIAN_POINT('Ctrl Pts',(-5.61908795299921,1.75940739601513,
-7.03035895690423));
#151708=CARTESIAN_POINT('Ctrl Pts',(-5.62668196880536,1.75748289679882,
-7.02428194266244));
#151709=CARTESIAN_POINT('Ctrl Pts',(-5.64191721405734,1.74964163118351,
-7.01205209704977));
#151710=CARTESIAN_POINT('Ctrl Pts',(-5.64921717518735,1.74349822264663,
-7.00616971270524));
#151711=CARTESIAN_POINT('Ctrl Pts',(-5.66374038085022,1.72630637181619,
-6.99443726335543));
#151712=CARTESIAN_POINT('Ctrl Pts',(-5.67036239905914,1.71456563927445,
-6.9890653110919));
#151713=CARTESIAN_POINT('Ctrl Pts',(-5.67669307213168,1.69868853641841,
-6.98392140317848));
#151714=CARTESIAN_POINT('Ctrl Pts',(-5.67781493935397,1.69560796508514,
-6.98300933113573));
#151715=CARTESIAN_POINT('Ctrl Pts',(-5.67885701524478,1.69247211100408,
-6.98216177128582));
#151716=CARTESIAN_POINT('Ctrl Pts',(-5.87836203940153,1.00000000015303,
-6.81504656871272));
#151717=CARTESIAN_POINT('Ctrl Pts',(-5.86864914972266,1.04120750297626,
-6.82342448387522));
#151718=CARTESIAN_POINT('Ctrl Pts',(-5.85851587727959,1.08227801693488,
-6.83212872970076));
#151719=CARTESIAN_POINT('Ctrl Pts',(-5.79884018861093,1.3147583177969,-6.88314141331103));
#151720=CARTESIAN_POINT('Ctrl Pts',(-5.74153585055806,1.50385659810718,
-6.9311826969984));
#151721=CARTESIAN_POINT('Ctrl Pts',(-5.6788570152349,1.69247211099862,-6.98216177129385));
#151722=CARTESIAN_POINT('',(-6.15668002,1.69247211199998,-6.564700384));
#151723=CARTESIAN_POINT('Ctrl Pts',(-6.15668002040535,1.69247211175397,
-6.56470038359265));
#151724=CARTESIAN_POINT('Ctrl Pts',(-6.09774873405703,1.50385659870572,
-6.6199688729428));
#151725=CARTESIAN_POINT('Ctrl Pts',(-6.04245008693597,1.31475831823908,
-6.67030585472521));
#151726=CARTESIAN_POINT('Ctrl Pts',(-5.98388861759739,1.0822780170448,-6.7225938651483));
#151727=CARTESIAN_POINT('Ctrl Pts',(-5.97390292497523,1.04120750291261,
-6.73146702975377));
#151728=CARTESIAN_POINT('Ctrl Pts',(-5.96429703900053,0.999999999914591,
-6.73996742058665));
#151729=CARTESIAN_POINT('',(-6.281871763,1.69247211199998,-6.445004822));
#151730=CARTESIAN_POINT('Ctrl Pts',(-6.15668002018172,1.69247211188528,
-6.56470038380239));
#151731=CARTESIAN_POINT('Ctrl Pts',(-6.158231985384,1.69743933273647,-6.56324487896678));
#151732=CARTESIAN_POINT('Ctrl Pts',(-6.15996290064517,1.70224131117035,
-6.56162052427873));
#151733=CARTESIAN_POINT('Ctrl Pts',(-6.16758457340519,1.7206485573853,-6.55446122979663));
#151734=CARTESIAN_POINT('Ctrl Pts',(-6.17471932200857,1.73230722877125,
-6.54774538278079));
#151735=CARTESIAN_POINT('Ctrl Pts',(-6.18826030448658,1.7468654660582,-6.53494359589355));
#151736=CARTESIAN_POINT('Ctrl Pts',(-6.19417168656543,1.75155833712512,
-6.52934271193098));
#151737=CARTESIAN_POINT('Ctrl Pts',(-6.20672502389223,1.75781013680233,
-6.51741017907483));
#151738=CARTESIAN_POINT('Ctrl Pts',(-6.21309382910321,1.75940739641427,
-6.51133973909935));
#151739=CARTESIAN_POINT('Ctrl Pts',(-6.21956384103444,1.75940739641324,
-6.50515377430056));
#151740=CARTESIAN_POINT('Ctrl Pts',(-6.22666367601187,1.75940739641211,
-6.49836563701204));
#151741=CARTESIAN_POINT('Ctrl Pts',(-6.23368238118683,1.7574828971896,-6.49163236471182));
#151742=CARTESIAN_POINT('Ctrl Pts',(-6.24776001891508,1.74964163156032,
-6.47808607599983));
#151743=CARTESIAN_POINT('Ctrl Pts',(-6.25450329968281,1.74349822301387,
-6.47157300893044));
#151744=CARTESIAN_POINT('Ctrl Pts',(-6.2679163505422,1.72630637215997,-6.45858594084605));
#151745=CARTESIAN_POINT('Ctrl Pts',(-6.27403017236557,1.71456563960319,
-6.4526420213443));
#151746=CARTESIAN_POINT('Ctrl Pts',(-6.2798742635728,1.69868853696113,-6.44695134421518));
#151747=CARTESIAN_POINT('Ctrl Pts',(-6.28090985690551,1.69560796586702,
-6.44594238057608));
#151748=CARTESIAN_POINT('Ctrl Pts',(-6.28187176296278,1.69247211203292,
-6.44500482185164));
#151749=CARTESIAN_POINT('Ctrl Pts',(-6.46559354741529,1.00000000002598,
-6.26067888328588));
#151750=CARTESIAN_POINT('Ctrl Pts',(-6.45667074945246,1.04120750309549,
-6.2698937281947));
#151751=CARTESIAN_POINT('Ctrl Pts',(-6.44735851311334,1.0822780172987,-6.27947127288012));
#151752=CARTESIAN_POINT('Ctrl Pts',(-6.39249580284863,1.31475831852555,
-6.3356278820062));
#151753=CARTESIAN_POINT('Ctrl Pts',(-6.33972854265469,1.5038565989558,-6.38861248690754));
#151754=CARTESIAN_POINT('Ctrl Pts',(-6.28187176285275,1.69247211196711,
-6.44500482195888));
#151755=CARTESIAN_POINT('',(-6.720350242,1.69247211199998,-5.986392288));
#151756=CARTESIAN_POINT('Ctrl Pts',(-6.72035024195089,1.69247211200556,
-5.98639228797367));
#151757=CARTESIAN_POINT('Ctrl Pts',(-6.66661042481084,1.50385659891639,
-6.04672084242625));
#151758=CARTESIAN_POINT('Ctrl Pts',(-6.61604656603123,1.31475831840883,
-6.10181211483948));
#151759=CARTESIAN_POINT('Ctrl Pts',(-6.56240790905556,1.0822780171616,-6.15913903875423));
#151760=CARTESIAN_POINT('Ctrl Pts',(-6.55325780023636,1.04120750301805,
-6.16887159319522));
#151761=CARTESIAN_POINT('Ctrl Pts',(-6.54445255389156,1.0000000000086,-6.17819882893568));
#151762=CARTESIAN_POINT('',(-6.834308572,1.69247211199998,-5.855956484));
#151763=CARTESIAN_POINT('Ctrl Pts',(-6.72035024189579,1.69247211204104,
-5.98639228803552));
#151764=CARTESIAN_POINT('Ctrl Pts',(-6.72176548885911,1.69743933272174,
-5.98480352558651));
#151765=CARTESIAN_POINT('Ctrl Pts',(-6.72334382988621,1.70224131099489,
-5.98303055207738));
#151766=CARTESIAN_POINT('Ctrl Pts',(-6.7302930657659,1.72064855706955,-5.97521687739586));
#151767=CARTESIAN_POINT('Ctrl Pts',(-6.73679708808431,1.73230722846238,
-5.96788851247172));
#151768=CARTESIAN_POINT('Ctrl Pts',(-6.74913601522039,1.74686546575903,
-5.95392445750275));
#151769=CARTESIAN_POINT('Ctrl Pts',(-6.75452154044654,1.75155833682971,
-5.94781622884727));
#151770=CARTESIAN_POINT('Ctrl Pts',(-6.76595471773228,1.75781013651241,
-5.93480646037548));
#151771=CARTESIAN_POINT('Ctrl Pts',(-6.77175373396333,1.75940739612622,
-5.92818956290777));
#151772=CARTESIAN_POINT('Ctrl Pts',(-6.77764319392101,1.75940739612599,
-5.92144853358502));
#151773=CARTESIAN_POINT('Ctrl Pts',(-6.78410596311402,1.75940739612575,
-5.91405129904242));
#151774=CARTESIAN_POINT('Ctrl Pts',(-6.79049284716903,1.75748289690447,
-5.90671598103711));
#151775=CARTESIAN_POINT('Ctrl Pts',(-6.80329953250677,1.74964163127831,
-5.89196231598691));
#151776=CARTESIAN_POINT('Ctrl Pts',(-6.80943183997698,1.74349822273392,
-5.88487100558439));
#151777=CARTESIAN_POINT('Ctrl Pts',(-6.82162674202863,1.72630637188464,
-5.87073388301057));
#151778=CARTESIAN_POINT('Ctrl Pts',(-6.82718314256655,1.71456563933025,
-5.86426585321871));
#151779=CARTESIAN_POINT('Ctrl Pts',(-6.83249359879879,1.69868853674338,
-5.85807422480591));
#151780=CARTESIAN_POINT('Ctrl Pts',(-6.83343458031894,1.69560796570414,
-5.85697649310469));
#151781=CARTESIAN_POINT('Ctrl Pts',(-6.83430857189647,1.69247211192666,
-5.85595648413667));
#151782=CARTESIAN_POINT('Ctrl Pts',(-7.00076789655381,0.999999999903773,
-5.65590389403687));
#151783=CARTESIAN_POINT('Ctrl Pts',(-6.99270703148499,1.04120750294805,
-5.66588147612623));
#151784=CARTESIAN_POINT('Ctrl Pts',(-6.98429080796196,1.08227801712618,
-5.67625520685598));
#151785=CARTESIAN_POINT('Ctrl Pts',(-6.93468279847113,1.31475831832256,
-5.73710360140729));
#151786=CARTESIAN_POINT('Ctrl Pts',(-6.88687746711329,1.50385659874697,
-5.79460492660105));
#151787=CARTESIAN_POINT('Ctrl Pts',(-6.83430857163228,1.69247211175275,
-5.855956484445));
#151788=CARTESIAN_POINT('',(-7.229912155,1.69247211199998,-5.359885281));
#151789=CARTESIAN_POINT('Ctrl Pts',(-7.22991215493042,1.69247211222666,
-5.35988528160718));
#151790=CARTESIAN_POINT('Ctrl Pts',(-7.18179648839481,1.50385659905977,
-5.4247881711377));
#151791=CARTESIAN_POINT('Ctrl Pts',(-7.13637452840358,1.31475831847509,
-5.48419017167095));
#151792=CARTESIAN_POINT('Ctrl Pts',(-7.08809055071594,1.08227801718246,
-5.54609444640031));
#151793=CARTESIAN_POINT('Ctrl Pts',(-7.07984969700402,1.04120750307276,
-5.55660802986153));
#151794=CARTESIAN_POINT('Ctrl Pts',(-7.07191598496282,1.00000000009741,
-5.56668701308303));
#151795=CARTESIAN_POINT('',(-7.331719547,1.69247211199998,-5.219759428));
#151796=CARTESIAN_POINT('Ctrl Pts',(-7.2299121553839,1.69247211190049,-5.35988528099549));
#151797=CARTESIAN_POINT('Ctrl Pts',(-7.23117928939508,1.69743933249794,
-5.35817605269869));
#151798=CARTESIAN_POINT('Ctrl Pts',(-7.23259234834446,1.70224131069263,
-5.35626873528853));
#151799=CARTESIAN_POINT('Ctrl Pts',(-7.23881319621897,1.72064855670075,
-5.34786359149697));
#151800=CARTESIAN_POINT('Ctrl Pts',(-7.24463412568797,1.73230722809895,
-5.33998171234982));
#151801=CARTESIAN_POINT('Ctrl Pts',(-7.25567165169415,1.74686546540357,
-5.3249678196583));
#151802=CARTESIAN_POINT('Ctrl Pts',(-7.26048795898428,1.75155833647739,
-5.31840142617492));
#151803=CARTESIAN_POINT('Ctrl Pts',(-7.2707089230063,1.75781013616434,-5.30441916909238));
#151804=CARTESIAN_POINT('Ctrl Pts',(-7.27589145998758,1.75940739577936,
-5.29730908949956));
#151805=CARTESIAN_POINT('Ctrl Pts',(-7.28115294950206,1.7594073957793,-5.29006727045672));
#151806=CARTESIAN_POINT('Ctrl Pts',(-7.28692661849261,1.75940739577923,
-5.28212049684293));
#151807=CARTESIAN_POINT('Ctrl Pts',(-7.29263025799209,1.75748289655853,
-5.27424219279995));
#151808=CARTESIAN_POINT('Ctrl Pts',(-7.30406287903831,1.7496416309341,-5.25839993924684));
#151809=CARTESIAN_POINT('Ctrl Pts',(-7.30953483947672,1.74349822239083,
-5.25078748057242));
#151810=CARTESIAN_POINT('Ctrl Pts',(-7.32041340653932,1.72630637154358,
-5.23561412730616));
#151811=CARTESIAN_POINT('Ctrl Pts',(-7.32536764892154,1.71456563898968,
-5.22867406399611));
#151812=CARTESIAN_POINT('Ctrl Pts',(-7.33010171347168,1.69868853658723,
-5.22203133570847));
#151813=CARTESIAN_POINT('Ctrl Pts',(-7.33094050691843,1.69560796573972,
-5.22085367428564));
#151814=CARTESIAN_POINT('Ctrl Pts',(-7.33171954712374,1.69247211216014,
-5.21975942762917));
#151815=CARTESIAN_POINT('Ctrl Pts',(-7.47957617958272,1.00000000003768,
-5.00559089157501));
#151816=CARTESIAN_POINT('Ctrl Pts',(-7.472442148756,1.0412075030462,-5.01625087721741));
#151817=CARTESIAN_POINT('Ctrl Pts',(-7.46498970053469,1.08227801718884,
-5.0273372708077));
#151818=CARTESIAN_POINT('Ctrl Pts',(-7.42103580633786,1.3147583184205,-5.09238753530659));
#151819=CARTESIAN_POINT('Ctrl Pts',(-7.37857730422628,1.50385659891382,
-5.15394261395913));
#151820=CARTESIAN_POINT('Ctrl Pts',(-7.33171954689144,1.69247211198855,
-5.21975942795546));
#151821=CARTESIAN_POINT('',(-7.681263067,1.69247211199998,-4.69022363));
#151822=CARTESIAN_POINT('Ctrl Pts',(-7.68126306643363,1.69247211231474,
-4.69022363051514));
#151823=CARTESIAN_POINT('Ctrl Pts',(-7.63915894961858,1.50385659926452,
-4.75917829513542));
#151824=CARTESIAN_POINT('Ctrl Pts',(-7.59924459938713,1.31475831879601,
-4.8224127537344));
#151825=CARTESIAN_POINT('Ctrl Pts',(-7.55670405519824,1.08227801749227,
-4.88839596244951));
#151826=CARTESIAN_POINT('Ctrl Pts',(-7.54943880707296,1.0412075032506,-4.89960592578131));
#151827=CARTESIAN_POINT('Ctrl Pts',(-7.54244050689292,1.00000000014238,
-4.91035550647617));
#151828=CARTESIAN_POINT('',(-7.770099827,1.69247211199998,-4.541535938));
#151829=CARTESIAN_POINT('Ctrl Pts',(-7.68126306658055,1.69247211219402,
-4.69022363027453));
#151830=CARTESIAN_POINT('Ctrl Pts',(-7.68237188542729,1.6974393327218,-4.68840769783155));
#151831=CARTESIAN_POINT('Ctrl Pts',(-7.68360828518667,1.70224131085113,
-4.68638139311886));
#151832=CARTESIAN_POINT('Ctrl Pts',(-7.68905065845813,1.72064855681643,
-4.6774524534919));
#151833=CARTESIAN_POINT('Ctrl Pts',(-7.69414162837981,1.73230722823066,
-4.6690805203751));
#151834=CARTESIAN_POINT('Ctrl Pts',(-7.70378888559198,1.74686546555534,
-4.65313767299271));
#151835=CARTESIAN_POINT('Ctrl Pts',(-7.7079971968728,1.75155833663595,-4.64616598342078));
#151836=CARTESIAN_POINT('Ctrl Pts',(-7.71692365444042,1.7578101363352,-4.6313238146405));
#151837=CARTESIAN_POINT('Ctrl Pts',(-7.72144798543252,1.75940739595605,
-4.6237777991027));
#151838=CARTESIAN_POINT('Ctrl Pts',(-7.72603914208534,1.75940739596087,
-4.61609349720791));
#151839=CARTESIAN_POINT('Ctrl Pts',(-7.73107722468816,1.75940739596616,
-4.6076611672705));
#151840=CARTESIAN_POINT('Ctrl Pts',(-7.73605169728343,1.75748289675087,
-4.59930330866004));
#151841=CARTESIAN_POINT('Ctrl Pts',(-7.74601820529917,1.74964163113785,
-4.58250001911516));
#151842=CARTESIAN_POINT('Ctrl Pts',(-7.75078576169847,1.74349822260255,
-4.57442770321189));
#151843=CARTESIAN_POINT('Ctrl Pts',(-7.76026040594584,1.726306371776,-4.55834028617847));
#151844=CARTESIAN_POINT('Ctrl Pts',(-7.76457260152491,1.7145656392368,-4.55098406666299));
#151845=CARTESIAN_POINT('Ctrl Pts',(-7.76869215858641,1.69868853671208,
-4.54394372171134));
#151846=CARTESIAN_POINT('Ctrl Pts',(-7.76942201057285,1.69560796572158,
-4.54269561228854));
#151847=CARTESIAN_POINT('Ctrl Pts',(-7.77009982710407,1.69247211199432,
-4.54153593807615));
#151848=CARTESIAN_POINT('Ctrl Pts',(-7.89816331283003,0.999999999979971,
-4.3149758149804));
#151849=CARTESIAN_POINT('Ctrl Pts',(-7.89201355528089,1.04120750283238,
-4.3262323762081));
#151850=CARTESIAN_POINT('Ctrl Pts',(-7.88558488510778,1.08227801681994,
-4.33794217150246));
#151851=CARTESIAN_POINT('Ctrl Pts',(-7.84763899711798,1.31475831805313,
-4.40667055946035));
#151852=CARTESIAN_POINT('Ctrl Pts',(-7.81086917512473,1.50385659869719,
-4.47178378631242));
#151853=CARTESIAN_POINT('Ctrl Pts',(-7.77009982702067,1.69247211192352,
-4.54153593821884));
#151854=CARTESIAN_POINT('',(-8.070768965,1.69247211199998,-3.982799055));
#151855=CARTESIAN_POINT('Ctrl Pts',(-8.07076896483244,1.69247211221444,
-3.98279905547561));
#151856=CARTESIAN_POINT('Ctrl Pts',(-8.03501539529515,1.50385659911875,
-4.05525031284116));
#151857=CARTESIAN_POINT('Ctrl Pts',(-8.00093002167116,1.31475831860448,
-4.12180810288601));
#151858=CARTESIAN_POINT('Ctrl Pts',(-7.96447542245618,1.08227801735784,
-4.19133898755908));
#151859=CARTESIAN_POINT('Ctrl Pts',(-7.95824427546741,1.04120750322134,
-4.20315507466473));
#151860=CARTESIAN_POINT('Ctrl Pts',(-7.95223773338732,1.00000000021904,
-4.21448870347174));
#151861=CARTESIAN_POINT('',(-8.1459198327977,1.69247211207413,-3.82674667047894));
#151862=CARTESIAN_POINT('Ctrl Pts',(-8.07076896488867,1.69247211216004,
-3.98279905536167));
#151863=CARTESIAN_POINT('Ctrl Pts',(-8.07171054104207,1.69743933278747,
-3.98089103954382));
#151864=CARTESIAN_POINT('Ctrl Pts',(-8.07276032688418,1.70224131101044,
-3.97876206207974));
#151865=CARTESIAN_POINT('Ctrl Pts',(-8.07738040680549,1.72064855704358,
-3.96938121711276));
#151866=CARTESIAN_POINT('Ctrl Pts',(-8.08170042767802,1.73230722844107,
-3.96058663591419));
#151867=CARTESIAN_POINT('Ctrl Pts',(-8.08987974204303,1.74686546574379,
-3.94384319628409));
#151868=CARTESIAN_POINT('Ctrl Pts',(-8.09344617446283,1.75155833681651,
-3.93652234257194));
#151869=CARTESIAN_POINT('Ctrl Pts',(-8.10100625498023,1.75781013650272,
-3.92093976251732));
#151870=CARTESIAN_POINT('Ctrl Pts',(-8.10483595272582,1.75940739611808,
-3.91301856711897));
#151871=CARTESIAN_POINT('Ctrl Pts',(-8.10871981121782,1.75940739611904,
-3.90495365185858));
#151872=CARTESIAN_POINT('Ctrl Pts',(-8.11298174375302,1.75940739612008,
-3.89610365775793));
#151873=CARTESIAN_POINT('Ctrl Pts',(-8.11718699791386,1.75748289690017,
-3.88733353714228));
#151874=CARTESIAN_POINT('Ctrl Pts',(-8.12560714843641,1.74964163127695,
-3.86970450180576));
#151875=CARTESIAN_POINT('Ctrl Pts',(-8.12963191523694,1.74349822273462,
-3.86123732220918));
#151876=CARTESIAN_POINT('Ctrl Pts',(-8.13762635240814,1.72630637189051,
-3.84436536781835));
#151877=CARTESIAN_POINT('Ctrl Pts',(-8.14126178192233,1.71456563933967,
-3.83665222004584));
#151878=CARTESIAN_POINT('Ctrl Pts',(-8.14473366319477,1.69868853683266,
-3.8292709432193));
#151879=CARTESIAN_POINT('Ctrl Pts',(-8.14534869733938,1.69560796587296,
-3.82796243490334));
#151880=CARTESIAN_POINT('Ctrl Pts',(-8.14591983278025,1.69247211217755,
-3.826746670204));
#151881=CARTESIAN_POINT('Ctrl Pts',(-8.25315907928445,1.00000000000618,
-3.589619090102));
#151882=CARTESIAN_POINT('Ctrl Pts',(-8.24804310921235,1.04120750292176,
-3.6013815957579));
#151883=CARTESIAN_POINT('Ctrl Pts',(-8.24268997692429,1.08227801697206,
-3.61362051242964));
#151884=CARTESIAN_POINT('Ctrl Pts',(-8.21105761312823,1.31475831812732,
-3.68547366326024));
#151885=CARTESIAN_POINT('Ctrl Pts',(-8.18027252030632,1.50385659863499,
-3.75362078478248));
#151886=CARTESIAN_POINT('Ctrl Pts',(-8.14591983233074,1.6924721117247,-3.82674667116087));
#151887=CARTESIAN_POINT('',(-8.395293776,1.69247211199998,-3.243307326));
#151888=CARTESIAN_POINT('Ctrl Pts',(-8.39529377643543,1.69247211171466,
-3.24330732545413));
#151889=CARTESIAN_POINT('Ctrl Pts',(-8.36617862092618,1.50385659880013,
-3.31867184053676));
#151890=CARTESIAN_POINT('Ctrl Pts',(-8.33819665932569,1.31475831846641,
-3.38801707774584));
#151891=CARTESIAN_POINT('Ctrl Pts',(-8.30812151607705,1.08227801737161,
-3.460535816552));
#151892=CARTESIAN_POINT('Ctrl Pts',(-8.30297463973183,1.04120750320158,
-3.47286289128436));
#151893=CARTESIAN_POINT('Ctrl Pts',(-8.29800821687382,1.0000000001655,-3.48468931652372));
#151894=CARTESIAN_POINT('',(-8.456153681,1.69247211199998,-3.081146689));
#151895=CARTESIAN_POINT('Ctrl Pts',(-8.39529377630737,1.69247211186686,
-3.24330732578562));
#151896=CARTESIAN_POINT('Ctrl Pts',(-8.39606052875182,1.69743933266437,
-3.24132258879396));
#151897=CARTESIAN_POINT('Ctrl Pts',(-8.39691524842105,1.70224131104791,
-3.23910807982608));
#151898=CARTESIAN_POINT('Ctrl Pts',(-8.4006758368303,1.72064855723026,-3.22935085853309));
#151899=CARTESIAN_POINT('Ctrl Pts',(-8.40419012638921,1.73230722862894,
-3.22020443804666));
#151900=CARTESIAN_POINT('Ctrl Pts',(-8.41083564288389,1.7468654659326,-3.20279521449444));
#151901=CARTESIAN_POINT('Ctrl Pts',(-8.41373148162846,1.75155833700544,
-3.19518413985006));
#151902=CARTESIAN_POINT('Ctrl Pts',(-8.41986431577829,1.75781013669251,
-3.17898661028975));
#151903=CARTESIAN_POINT('Ctrl Pts',(-8.42296854580602,1.75940739630863,
-3.17075401183652));
#151904=CARTESIAN_POINT('Ctrl Pts',(-8.42611383559583,1.75940739631059,
-3.1623734171632));
#151905=CARTESIAN_POINT('Ctrl Pts',(-8.42956530348967,1.75940739631274,
-3.15317701384931));
#151906=CARTESIAN_POINT('Ctrl Pts',(-8.43296748098366,1.75748289709377,
-3.1440652430834));
#151907=CARTESIAN_POINT('Ctrl Pts',(-8.43977347991322,1.74964163147231,
-3.12575240058616));
#151908=CARTESIAN_POINT('Ctrl Pts',(-8.44302305205915,1.74349822293125,
-3.11695853005104));
#151909=CARTESIAN_POINT('Ctrl Pts',(-8.44947291564613,1.72630637209083,
-3.09943788136671));
#151910=CARTESIAN_POINT('Ctrl Pts',(-8.45240230875442,1.71456563954304,
-3.09142990707129));
#151911=CARTESIAN_POINT('Ctrl Pts',(-8.45519856073018,1.69868853687056,
-3.08376712797648));
#151912=CARTESIAN_POINT('Ctrl Pts',(-8.45569382517283,1.69560796573517,
-3.08240875602404));
#151913=CARTESIAN_POINT('Ctrl Pts',(-8.45615368110476,1.69247211185841,
-3.08114668938989));
#151914=CARTESIAN_POINT('Ctrl Pts',(-8.54170526185697,0.999999999891994,
-2.83536086231805));
#151915=CARTESIAN_POINT('Ctrl Pts',(-8.53766427004687,1.04120750290419,
-2.84753460763075));
#151916=CARTESIAN_POINT('Ctrl Pts',(-8.53342977591951,1.08227801705046,
-2.8602041051281));
#151917=CARTESIAN_POINT('Ctrl Pts',(-8.50836562150266,1.31475831827597,
-2.93460349954225));
#151918=CARTESIAN_POINT('Ctrl Pts',(-8.48381312130125,1.50385659875945,
-3.00523583521544));
#151919=CARTESIAN_POINT('Ctrl Pts',(-8.45615368107748,1.69247211182429,
-3.08114668946476));
#151920=CARTESIAN_POINT('',(-8.652224619,1.69247211199998,-2.477702391));
#151921=CARTESIAN_POINT('Ctrl Pts',(-8.65222461931464,1.69247211184308,
-2.47770239070908));
#151922=CARTESIAN_POINT('Ctrl Pts',(-8.6299822958743,1.50385659864939,-2.55537337297999));
#151923=CARTESIAN_POINT('Ctrl Pts',(-8.60832904052779,1.31475831803842,
-2.62694773048628));
#151924=CARTESIAN_POINT('Ctrl Pts',(-8.58487550058799,1.08227801688606,
-2.70187044525523));
#151925=CARTESIAN_POINT('Ctrl Pts',(-8.58085433453559,1.04120750294561,
-2.7146092571805));
#151926=CARTESIAN_POINT('Ctrl Pts',(-8.57696801764159,1.00000000014065,
-2.72683325936026));
#151927=CARTESIAN_POINT('',(-8.69830355250517,1.69247211177544,-2.31073912599594));
#151928=CARTESIAN_POINT('Ctrl Pts',(-8.65222461924908,1.6924721119451,-2.47770239093806));
#151929=CARTESIAN_POINT('Ctrl Pts',(-8.65281037451572,1.69743933267268,
-2.4756569127735));
#151930=CARTESIAN_POINT('Ctrl Pts',(-8.65346314627405,1.70224131098984,
-2.47337470231207));
#151931=CARTESIAN_POINT('Ctrl Pts',(-8.6563339650763,1.7206485570939,-2.46331966420912));
#151932=CARTESIAN_POINT('Ctrl Pts',(-8.65901422832519,1.73230722847676,
-2.45389504603903));
#151933=CARTESIAN_POINT('Ctrl Pts',(-8.66407244115263,1.74686546576065,
-2.43596020740362));
#151934=CARTESIAN_POINT('Ctrl Pts',(-8.66627437062938,1.75155833682684,
-2.428120191726));
#151935=CARTESIAN_POINT('Ctrl Pts',(-8.67093058043352,1.75781013650177,
-2.41143812564638));
#151936=CARTESIAN_POINT('Ctrl Pts',(-8.6732843493065,1.7594073961121,-2.40296040818193));
#151937=CARTESIAN_POINT('Ctrl Pts',(-8.6756657463679,1.75940739610916,-2.3943316097188));
#151938=CARTESIAN_POINT('Ctrl Pts',(-8.67827896042827,1.75940739610594,
-2.38486284122433));
#151939=CARTESIAN_POINT('Ctrl Pts',(-8.68085066892036,1.75748289688156,
-2.37548278293022));
#151940=CARTESIAN_POINT('Ctrl Pts',(-8.68598771835229,1.74964163124873,
-2.35663357751049));
#151941=CARTESIAN_POINT('Ctrl Pts',(-8.68843593219853,1.74349822269972,
-2.34758381910882));
#151942=CARTESIAN_POINT('Ctrl Pts',(-8.6932892916914,1.72630637183859,-2.32955554208355));
#151943=CARTESIAN_POINT('Ctrl Pts',(-8.69548906264279,1.71456563927603,
-2.32131721676111));
#151944=CARTESIAN_POINT('Ctrl Pts',(-8.69758717149787,1.69868853665797,
-2.31343463170189));
#151945=CARTESIAN_POINT('Ctrl Pts',(-8.69795867862004,1.69560796559486,
-2.31203733302424));
#151946=CARTESIAN_POINT('Ctrl Pts',(-8.69830355251919,1.69247211179278,
-2.31073912595777));
#151947=CARTESIAN_POINT('Ctrl Pts',(-8.76147865593336,0.999999999896205,
-2.05827397632681));
#151948=CARTESIAN_POINT('Ctrl Pts',(-8.75854517807591,1.0412075030467,-2.07076094547247));
#151949=CARTESIAN_POINT('Ctrl Pts',(-8.75546341576689,1.08227801733034,
-2.08375901646764));
#151950=CARTESIAN_POINT('Ctrl Pts',(-8.73716927257158,1.31475831846968,
-2.16010563424933));
#151951=CARTESIAN_POINT('Ctrl Pts',(-8.71904704729885,1.5038565987368,-2.23265449395954));
#151952=CARTESIAN_POINT('Ctrl Pts',(-8.69830355239435,1.6924721115845,-2.3107391264277));
#151953=CARTESIAN_POINT('',(-8.839492837,1.69247211199998,-1.692148455));
#151954=CARTESIAN_POINT('Ctrl Pts',(-8.83949283651608,1.69247211196708,
-1.69214845482919));
#151955=CARTESIAN_POINT('Ctrl Pts',(-8.82430242730659,1.50385659886907,
-1.77150054300318));
#151956=CARTESIAN_POINT('Ctrl Pts',(-8.80915221754667,1.31475831835278,
-1.84472774598002));
#151957=CARTESIAN_POINT('Ctrl Pts',(-8.79250911503047,1.08227801717924,
-1.92145120303552));
#151958=CARTESIAN_POINT('Ctrl Pts',(-8.78964603529871,1.04120750311893,
-1.93449918683022));
#151959=CARTESIAN_POINT('Ctrl Pts',(-8.78687111467304,1.00000000019332,
-1.94702234556372));
#151960=CARTESIAN_POINT('',(-8.870419798,1.69247211199998,-1.521726851));
#151961=CARTESIAN_POINT('Ctrl Pts',(-8.83949283655333,1.6924721118822,-1.69214845463461));
#151962=CARTESIAN_POINT('Ctrl Pts',(-8.83989287848787,1.69743933253479,
-1.6900587042909));
#151963=CARTESIAN_POINT('Ctrl Pts',(-8.84033844660458,1.70224131078141,
-1.68772716736002));
#151964=CARTESIAN_POINT('Ctrl Pts',(-8.84229638166105,1.72064855683224,
-1.67745526970967));
#151965=CARTESIAN_POINT('Ctrl Pts',(-8.84412103869949,1.7323072282259,-1.66782833533496));
#151966=CARTESIAN_POINT('Ctrl Pts',(-8.84755122211043,1.74686546552436,
-1.64951228238131));
#151967=CARTESIAN_POINT('Ctrl Pts',(-8.84904151368015,1.75155833659586,
-1.64150644886352));
#151968=CARTESIAN_POINT('Ctrl Pts',(-8.85218361007993,1.75781013627922,
-1.62447416044409));
#151969=CARTESIAN_POINT('Ctrl Pts',(-8.85376796663778,1.75940739589287,
-1.61581958156026));
#151970=CARTESIAN_POINT('Ctrl Pts',(-8.8553662973649,1.759407395892,-1.60701205331319));
#151971=CARTESIAN_POINT('Ctrl Pts',(-8.85712021753,1.75940739589105,-1.59734715659617));
#151972=CARTESIAN_POINT('Ctrl Pts',(-8.85884075113716,1.75748289666931,
-1.58777433348841));
#151973=CARTESIAN_POINT('Ctrl Pts',(-8.86226749057167,1.74964163104244,
-1.56854052787078));
#151974=CARTESIAN_POINT('Ctrl Pts',(-8.86389463454005,1.74349822249752,
-1.55930774494077));
#151975=CARTESIAN_POINT('Ctrl Pts',(-8.86711241354167,1.72630637164629,
-1.54091699267149));
#151976=CARTESIAN_POINT('Ctrl Pts',(-8.8685648510738,1.71456563908994,-1.53251464647819));
#151977=CARTESIAN_POINT('Ctrl Pts',(-8.86994792407433,1.69868853657767,
-1.5244757214109));
#151978=CARTESIAN_POINT('Ctrl Pts',(-8.87019268272298,1.6956079656182,-1.52305074624817));
#151979=CARTESIAN_POINT('Ctrl Pts',(-8.87041979787082,1.69247211192306,
-1.52172685116002));
#151980=CARTESIAN_POINT('Ctrl Pts',(-8.91070977542002,0.999999999993989,
-1.26461507907905));
#151981=CARTESIAN_POINT('Ctrl Pts',(-8.90890743017016,1.04120750304135,
-1.27731473425656));
#151982=CARTESIAN_POINT('Ctrl Pts',(-8.9070032122354,1.08227801722256,-1.2905367258509));
#151983=CARTESIAN_POINT('Ctrl Pts',(-8.89562637393288,1.31475831840746,
-1.36821586896249));
#151984=CARTESIAN_POINT('Ctrl Pts',(-8.88408033304455,1.50385659881792,
-1.44209713210709));
#151985=CARTESIAN_POINT('Ctrl Pts',(-8.87041979782602,1.69247211180957,
-1.52172685142118));
#151986=CARTESIAN_POINT('',(-8.955590655,1.69247211199998,-0.892970333000001));
#151987=CARTESIAN_POINT('Ctrl Pts',(-8.9555906552352,1.69247211204864,-0.892970333137612));
#151988=CARTESIAN_POINT('Ctrl Pts',(-8.94757446449693,1.50385659895089,
-0.97336463091238));
#151989=CARTESIAN_POINT('Ctrl Pts',(-8.93904928090067,1.3147583184345,-1.04765509702603));
#151990=CARTESIAN_POINT('Ctrl Pts',(-8.92935061629266,1.0822780171992,-1.12556156422249));
#151991=CARTESIAN_POINT('Ctrl Pts',(-8.92766867472662,1.04120750307671,
-1.13881366517733));
#151992=CARTESIAN_POINT('Ctrl Pts',(-8.92602749240836,1.00000000008849,
-1.15153515133937));
#151993=CARTESIAN_POINT('',(-8.971116639,1.69247211199998,-0.720462525999999));
#151994=CARTESIAN_POINT('Ctrl Pts',(-8.95559065523919,1.69247211203143,
-0.892970333097604));
#151995=CARTESIAN_POINT('Ctrl Pts',(-8.9558017629423,1.69743933257032,-0.890853136027187));
#151996=CARTESIAN_POINT('Ctrl Pts',(-8.95603653996893,1.7022413107097,-0.888491044806472));
#151997=CARTESIAN_POINT('Ctrl Pts',(-8.95706582714206,1.72064855666438,
-0.878084990907433));
#151998=CARTESIAN_POINT('Ctrl Pts',(-8.95802018690317,1.73230722806008,
-0.868333250744462));
#151999=CARTESIAN_POINT('Ctrl Pts',(-8.95979472307499,1.7468654653616,-0.849783453564588));
#152000=CARTESIAN_POINT('Ctrl Pts',(-8.96056137778506,1.75155833643442,
-0.841676260471871));
#152001=CARTESIAN_POINT('Ctrl Pts',(-8.96216406246514,1.7578101361195,-0.824430883686811));
#152002=CARTESIAN_POINT('Ctrl Pts',(-8.96296625039908,1.7594073957336,-0.815669124965457));
#152003=CARTESIAN_POINT('Ctrl Pts',(-8.96376864597117,1.75940739573272,
-0.806753779975071));
#152004=CARTESIAN_POINT('Ctrl Pts',(-8.96464915070661,1.75940739573176,
-0.796970571100177));
#152005=CARTESIAN_POINT('Ctrl Pts',(-8.96550465670328,1.75748289651018,
-0.787282057921237));
#152006=CARTESIAN_POINT('Ctrl Pts',(-8.9671934960484,1.74964163088392,-0.767818511397056));
#152007=CARTESIAN_POINT('Ctrl Pts',(-8.96798646933209,1.74349822233936,
-0.758477040876453));
#152008=CARTESIAN_POINT('Ctrl Pts',(-8.96954276017722,1.72630637148871,
-0.739871884883414));
#152009=CARTESIAN_POINT('Ctrl Pts',(-8.97023617011667,1.71456563893235,
-0.731373168568874));
#152010=CARTESIAN_POINT('Ctrl Pts',(-8.97089307157978,1.69868853652994,
-0.723242628198457));
#152011=CARTESIAN_POINT('Ctrl Pts',(-8.97100911110934,1.695607965685,-0.72180144961933));
#152012=CARTESIAN_POINT('Ctrl Pts',(-8.97111663891427,1.6924721121081,-0.720462525739919));
#152013=CARTESIAN_POINT('Ctrl Pts',(-8.98819709930371,0.999999999959407,
-0.460774244146092));
#152014=CARTESIAN_POINT('Ctrl Pts',(-8.98754039807928,1.04120750304597,
-0.473584335238514));
#152015=CARTESIAN_POINT('Ctrl Pts',(-8.98682905615476,1.08227801726612,
-0.486923791773003));
#152016=CARTESIAN_POINT('Ctrl Pts',(-8.98246112236426,1.31475831853778,
-0.56531003343955));
#152017=CARTESIAN_POINT('Ctrl Pts',(-8.9775842278123,1.50385659899527,-0.639928851482268));
#152018=CARTESIAN_POINT('Ctrl Pts',(-8.97111663890039,1.69247211203383,
-0.72046252591272));
#152019=CARTESIAN_POINT('',(-8.999583324,1.69247211199998,-0.0866025400000003));
#152020=CARTESIAN_POINT('Ctrl Pts',(-8.99958332369346,1.69247211191239,
-0.0866025397925534));
#152021=CARTESIAN_POINT('Ctrl Pts',(-8.99880589307639,1.50385659887802,
-0.167391759525919));
#152022=CARTESIAN_POINT('Ctrl Pts',(-8.99697437540592,1.31475831842477,
-0.242147345601193));
#152023=CARTESIAN_POINT('Ctrl Pts',(-8.99429823665166,1.08227801725347,
-0.320609565836488));
#152024=CARTESIAN_POINT('Ctrl Pts',(-8.99381097525933,1.04120750313013,
-0.333959085808913));
#152025=CARTESIAN_POINT('Ctrl Pts',(-8.9933167450867,1.00000000014106,-0.346776473456898));
#152026=CARTESIAN_POINT('Ctrl Pts',(-8.9995833236904,1.69247211204887,-0.0866025401111392));
#152027=CARTESIAN_POINT('Ctrl Pts',(-8.99960379745391,1.69743933262498,
-0.0844749426937014));
#152028=CARTESIAN_POINT('Ctrl Pts',(-8.99962589311285,1.70224131079953,
-0.082101315292519));
#152029=CARTESIAN_POINT('Ctrl Pts',(-8.99971824519885,1.72064855678832,
-0.0716448884975285));
#152030=CARTESIAN_POINT('Ctrl Pts',(-8.99979462373951,1.73230722818554,
-0.0618468578231623));
#152031=CARTESIAN_POINT('Ctrl Pts',(-8.99989922515123,1.7468654654886,-0.0432126684760381));
#152032=CARTESIAN_POINT('Ctrl Pts',(-8.999936070349,1.75155833656183,-0.0350693901608667));
#152033=CARTESIAN_POINT('Ctrl Pts',(-8.99998643943524,1.75781013624805,
-0.0177497746457722));
#152034=CARTESIAN_POINT('Ctrl Pts',(-9.,1.75940739586291,-0.00895138061713929));
#152035=CARTESIAN_POINT('Ctrl Pts',(-9.,1.75940739586291,2.22044604925031E-15));
#152036=CARTESIAN_POINT('Origin',(1.11022302462516E-15,2.49999999999998,
2.22044604925031E-15));
#152037=CARTESIAN_POINT('',(-3.5,2.49999999999998,2.64907242895189E-15));
#152038=CARTESIAN_POINT('',(-3.5,2.49999999999998,2.64907242895189E-15));
#152039=CARTESIAN_POINT('Origin',(1.11022302462516E-15,2.49999999999998,
2.22044604925031E-15));
#152040=CARTESIAN_POINT('Origin',(1.11022302462516E-15,2.49999999999998,
2.22044604925031E-15));
#152041=CARTESIAN_POINT('',(-2.5,2.49999999999998,2.52660774903715E-15));
#152042=CARTESIAN_POINT('Origin',(3.5,4.99999999999998,2.22044604925031E-15));
#152043=CARTESIAN_POINT('Origin',(9.,2.49999999999998,2.22044604925031E-15));
#152044=CARTESIAN_POINT('Origin',(2.5,-1.50000000000002,2.22044604925031E-15));
#152045=CARTESIAN_POINT('Origin',(10.516666667,-1.77635683940025E-14,0.0866025400000026));
#152046=CARTESIAN_POINT('Origin',(10.516666667,-1.77635683940025E-14,0.0866025400000026));
#152047=CARTESIAN_POINT('Origin',(10.516666667,-1.77635683940025E-14,2.22044604925031E-15));
#152048=CARTESIAN_POINT('Origin',(10.516666667,-1.77635683940025E-14,-0.0866025400000003));
#152049=CARTESIAN_POINT('Origin',(10.516666667,-1.77635683940025E-14,-0.349999999999999));
#152050=CARTESIAN_POINT('Origin',(10.48209265,-1.77635683940025E-14,-0.856452827999998));
#152051=CARTESIAN_POINT('Origin',(10.48209265,-1.77635683940025E-14,-0.856452827999998));
#152052=CARTESIAN_POINT('Origin',(10.474329659,-1.77635683940025E-14,-0.942706732));
#152053=CARTESIAN_POINT('Origin',(10.466566667,-1.77635683940025E-14,-1.028960636));
#152054=CARTESIAN_POINT('Origin',(10.4429559,-1.77635683940025E-14,-1.291297735));
#152055=CARTESIAN_POINT('Origin',(10.363122987,-1.77635683940025E-14,-1.792612542));
#152056=CARTESIAN_POINT('Origin',(10.363122987,-1.77635683940025E-14,-1.792612542));
#152057=CARTESIAN_POINT('Origin',(10.347659507,-1.77635683940025E-14,-1.877823344));
#152058=CARTESIAN_POINT('Origin',(10.332196026,-1.77635683940025E-14,-1.963034146));
#152059=CARTESIAN_POINT('Origin',(10.285164594,-1.77635683940025E-14,-2.2221987));
#152060=CARTESIAN_POINT('Origin',(10.160715552,-1.77635683940025E-14,-2.714339193));
#152061=CARTESIAN_POINT('Origin',(10.160715552,-1.77635683940025E-14,-2.714339193));
#152062=CARTESIAN_POINT('Origin',(10.137676085,-1.77635683940025E-14,-2.797820826));
#152063=CARTESIAN_POINT('Origin',(10.114636618,-1.77635683940025E-14,-2.881302458));
#152064=CARTESIAN_POINT('Origin',(10.044563189,-1.77635683940025E-14,-3.135207827));
#152065=CARTESIAN_POINT('Origin',(9.876500009,-1.77635683940025E-14,-3.614211582));
#152066=CARTESIAN_POINT('Origin',(9.876500009,-1.77635683940025E-14,-3.614211582));
#152067=CARTESIAN_POINT('Origin',(9.846070056,-1.77635683940025E-14,-3.6952919));
#152068=CARTESIAN_POINT('Origin',(9.815640104,-1.77635683940025E-14,-3.776372218));
#152069=CARTESIAN_POINT('Origin',(9.723088868,-1.77635683940025E-14,-4.022974105));
#152070=CARTESIAN_POINT('Origin',(9.512764695,-1.77635683940025E-14,-4.484984464));
#152071=CARTESIAN_POINT('Origin',(9.512764695,-1.77635683940025E-14,-4.484984464));
#152072=CARTESIAN_POINT('Origin',(9.475189261,-1.77635683940025E-14,-4.563010656));
#152073=CARTESIAN_POINT('Origin',(9.437613827,-1.77635683940025E-14,-4.641036849));
#152074=CARTESIAN_POINT('Origin',(9.323329952,-1.77635683940025E-14,-4.87834976));
#152075=CARTESIAN_POINT('Origin',(9.072438193,-1.77635683940025E-14,-5.319646888));
#152076=CARTESIAN_POINT('Origin',(9.072438193,-1.77635683940025E-14,-5.319646888));
#152077=CARTESIAN_POINT('Origin',(9.028019813,-1.77635683940025E-14,-5.393990734));
#152078=CARTESIAN_POINT('Origin',(8.983601433,-1.77635683940025E-14,-5.46833458));
#152079=CARTESIAN_POINT('Origin',(8.848505066,-1.77635683940025E-14,-5.694447812));
#152080=CARTESIAN_POINT('Origin',(8.559065754,-1.77635683940025E-14,-6.111478643));
#152081=CARTESIAN_POINT('Origin',(8.559065754,-1.77635683940025E-14,-6.111478643));
#152082=CARTESIAN_POINT('Origin',(8.508162058,-1.77635683940025E-14,-6.18154157));
#152083=CARTESIAN_POINT('Origin',(8.457258362,-1.77635683940025E-14,-6.251604497));
#152084=CARTESIAN_POINT('Origin',(8.302437219,-1.77635683940025E-14,-6.464697518));
#152085=CARTESIAN_POINT('Origin',(7.976780749,-1.77635683940025E-14,-6.854104366));
#152086=CARTESIAN_POINT('Origin',(7.976780749,-1.77635683940025E-14,-6.854104366));
#152087=CARTESIAN_POINT('Origin',(7.919801584,-1.77635683940025E-14,-6.919322268));
#152088=CARTESIAN_POINT('Origin',(7.862822419,-1.77635683940025E-14,-6.98454017));
#152089=CARTESIAN_POINT('Origin',(7.68952303,-1.77635683940025E-14,-7.182897281));
#152090=CARTESIAN_POINT('Origin',(7.330271397,-1.77635683940025E-14,-7.54154487));
#152091=CARTESIAN_POINT('Origin',(7.330271397,-1.77635683940025E-14,-7.54154487));
#152092=CARTESIAN_POINT('Origin',(7.267675525,-1.77635683940025E-14,-7.601392651));
#152093=CARTESIAN_POINT('Origin',(7.205079654,-1.77635683940025E-14,-7.661240432));
#152094=CARTESIAN_POINT('Origin',(7.014697323,-1.77635683940025E-14,-7.843264578));
#152095=CARTESIAN_POINT('Origin',(6.624743009,-1.77635683940025E-14,-8.16826529));
#152096=CARTESIAN_POINT('Origin',(6.624743009,-1.77635683940025E-14,-8.16826529));
#152097=CARTESIAN_POINT('Origin',(6.557034416,-1.77635683940025E-14,-8.222261091));
#152098=CARTESIAN_POINT('Origin',(6.489325824,-1.77635683940025E-14,-8.276256891));
#152099=CARTESIAN_POINT('Origin',(6.283393397,-1.77635683940025E-14,-8.440482521));
#152100=CARTESIAN_POINT('Origin',(5.865876086,-1.77635683940025E-14,-8.72921964));
#152101=CARTESIAN_POINT('Origin',(5.865876086,-1.77635683940025E-14,-8.72921964));
#152102=CARTESIAN_POINT('Origin',(5.793599922,-1.77635683940025E-14,-8.776928718));
#152103=CARTESIAN_POINT('Origin',(5.721323758,-1.77635683940025E-14,-8.824637796));
#152104=CARTESIAN_POINT('Origin',(5.501499283,-1.77635683940025E-14,-8.969742662));
#152105=CARTESIAN_POINT('Origin',(5.059780577,-1.77635683940025E-14,-9.219891447));
#152106=CARTESIAN_POINT('Origin',(5.059780577,-1.77635683940025E-14,-9.219891447));
#152107=CARTESIAN_POINT('Origin',(4.983518767,-1.77635683940025E-14,-9.260929677));
#152108=CARTESIAN_POINT('Origin',(4.907256957,-1.77635683940025E-14,-9.301967907));
#152109=CARTESIAN_POINT('Origin',(4.675310331,-1.77635683940025E-14,-9.426783709));
#152110=CARTESIAN_POINT('Origin',(4.212946691,-1.77635683940025E-14,-9.636330108));
#152111=CARTESIAN_POINT('Origin',(4.212946691,-1.77635683940025E-14,-9.636330108));
#152112=CARTESIAN_POINT('Origin',(4.13331325,-1.77635683940025E-14,-9.670367075));
#152113=CARTESIAN_POINT('Origin',(4.053679809,-1.77635683940025E-14,-9.704404041));
#152114=CARTESIAN_POINT('Origin',(3.811478529,-1.77635683940025E-14,-9.807925836));
#152115=CARTESIAN_POINT('Origin',(3.332192635,-1.77635683940025E-14,-9.975182706));
#152116=CARTESIAN_POINT('Origin',(3.332192635,-1.77635683940025E-14,-9.975182706));
#152117=CARTESIAN_POINT('Origin',(3.249828724,-1.77635683940025E-14,-10.001944363));
#152118=CARTESIAN_POINT('Origin',(3.167464814,-1.77635683940025E-14,-10.02870602));
#152119=CARTESIAN_POINT('Origin',(2.916958943,-1.77635683940025E-14,-10.110100311));
#152120=CARTESIAN_POINT('Origin',(2.424609723,-1.77635683940025E-14,-10.233720998));
#152121=CARTESIAN_POINT('Origin',(2.424609723,-1.77635683940025E-14,-10.233720998));
#152122=CARTESIAN_POINT('Origin',(2.340178489,-1.77635683940025E-14,-10.252991876));
#152123=CARTESIAN_POINT('Origin',(2.255747255,-1.77635683940025E-14,-10.272262754));
#152124=CARTESIAN_POINT('Origin',(1.99895372,-1.77635683940025E-14,-10.330874203));
#152125=CARTESIAN_POINT('Origin',(1.497505279,-1.77635683940025E-14,-10.409863386));
#152126=CARTESIAN_POINT('Origin',(1.497505279,-1.77635683940025E-14,-10.409863386));
#152127=CARTESIAN_POINT('Origin',(1.411686512,-1.77635683940025E-14,-10.421488328));
#152128=CARTESIAN_POINT('Origin',(1.325867745,-1.77635683940025E-14,-10.43311327));
#152129=CARTESIAN_POINT('Origin',(1.064854096,-1.77635683940025E-14,-10.468469971));
#152130=CARTESIAN_POINT('Origin',(0.558343803000001,-1.77635683940025E-14,
-10.502191675));
#152131=CARTESIAN_POINT('Origin',(0.558343803000001,-1.77635683940025E-14,
-10.502191675));
#152132=CARTESIAN_POINT('Origin',(0.471828466000001,-1.77635683940025E-14,
-10.506077083));
#152133=CARTESIAN_POINT('Origin',(0.385313129000001,-1.77635683940025E-14,
-10.509962491));
#152134=CARTESIAN_POINT('Origin',(0.122180893,-1.77635683940025E-14,-10.521779774));
#152135=CARTESIAN_POINT('Origin',(-0.385313127999999,-1.77635683940025E-14,
-10.509962491));
#152136=CARTESIAN_POINT('Origin',(-0.385313127999999,-1.77635683940025E-14,
-10.509962491));
#152137=CARTESIAN_POINT('Origin',(-0.471828465999998,-1.77635683940025E-14,
-10.506077083));
#152138=CARTESIAN_POINT('Origin',(-0.558343802999999,-1.77635683940025E-14,
-10.502191675));
#152139=CARTESIAN_POINT('Origin',(-0.821476038999999,-1.77635683940025E-14,
-10.490374393));
#152140=CARTESIAN_POINT('Origin',(-1.325867745,-1.77635683940025E-14,-10.43311327));
#152141=CARTESIAN_POINT('Origin',(-1.325867745,-1.77635683940025E-14,-10.43311327));
#152142=CARTESIAN_POINT('Origin',(-1.411686512,-1.77635683940025E-14,-10.421488328));
#152143=CARTESIAN_POINT('Origin',(-1.497505279,-1.77635683940025E-14,-10.409863386));
#152144=CARTESIAN_POINT('Origin',(-1.758518929,-1.77635683940025E-14,-10.374506685));
#152145=CARTESIAN_POINT('Origin',(-2.255747255,-1.77635683940025E-14,-10.272262755));
#152146=CARTESIAN_POINT('Origin',(-2.255747255,-1.77635683940025E-14,-10.272262755));
#152147=CARTESIAN_POINT('Origin',(-2.340178489,-1.77635683940025E-14,-10.252991876));
#152148=CARTESIAN_POINT('Origin',(-2.424609723,-1.77635683940025E-14,-10.233720998));
#152149=CARTESIAN_POINT('Origin',(-2.681403258,-1.77635683940025E-14,-10.17510955));
#152150=CARTESIAN_POINT('Origin',(-3.167464814,-1.77635683940025E-14,-10.02870602));
#152151=CARTESIAN_POINT('Origin',(-3.167464814,-1.77635683940025E-14,-10.02870602));
#152152=CARTESIAN_POINT('Origin',(-3.249828724,-1.77635683940025E-14,-10.001944363));
#152153=CARTESIAN_POINT('Origin',(-3.332192634,-1.77635683940025E-14,-9.975182706));
#152154=CARTESIAN_POINT('Origin',(-3.582698505,-1.77635683940025E-14,-9.893788415));
#152155=CARTESIAN_POINT('Origin',(-4.053679809,-1.77635683940025E-14,-9.704404041));
#152156=CARTESIAN_POINT('Origin',(-4.053679809,-1.77635683940025E-14,-9.704404041));
#152157=CARTESIAN_POINT('Origin',(-4.13331325,-1.77635683940025E-14,-9.670367075));
#152158=CARTESIAN_POINT('Origin',(-4.212946691,-1.77635683940025E-14,-9.636330109));
#152159=CARTESIAN_POINT('Origin',(-4.45514797,-1.77635683940025E-14,-9.532808314));
#152160=CARTESIAN_POINT('Origin',(-4.907256957,-1.77635683940025E-14,-9.301967907));
#152161=CARTESIAN_POINT('Origin',(-4.907256957,-1.77635683940025E-14,-9.301967907));
#152162=CARTESIAN_POINT('Origin',(-4.983518767,-1.77635683940025E-14,-9.260929677));
#152163=CARTESIAN_POINT('Origin',(-5.059780577,-1.77635683940025E-14,-9.219891447));
#152164=CARTESIAN_POINT('Origin',(-5.291727203,-1.77635683940025E-14,-9.095075645));
#152165=CARTESIAN_POINT('Origin',(-5.721323758,-1.77635683940025E-14,-8.824637796));
#152166=CARTESIAN_POINT('Origin',(-5.721323758,-1.77635683940025E-14,-8.824637796));
#152167=CARTESIAN_POINT('Origin',(-5.793599922,-1.77635683940025E-14,-8.776928718));
#152168=CARTESIAN_POINT('Origin',(-5.865876086,-1.77635683940025E-14,-8.72921964));
#152169=CARTESIAN_POINT('Origin',(-6.08570056,-1.77635683940025E-14,-8.584114775));
#152170=CARTESIAN_POINT('Origin',(-6.489325824,-1.77635683940025E-14,-8.276256891));
#152171=CARTESIAN_POINT('Origin',(-6.489325824,-1.77635683940025E-14,-8.276256891));
#152172=CARTESIAN_POINT('Origin',(-6.557034416,-1.77635683940025E-14,-8.222261091));
#152173=CARTESIAN_POINT('Origin',(-6.624743009,-1.77635683940025E-14,-8.16826529));
#152174=CARTESIAN_POINT('Origin',(-6.830675435,-1.77635683940025E-14,-8.00403966));
#152175=CARTESIAN_POINT('Origin',(-7.205079654,-1.77635683940025E-14,-7.661240432));
#152176=CARTESIAN_POINT('Origin',(-7.205079654,-1.77635683940025E-14,-7.661240432));
#152177=CARTESIAN_POINT('Origin',(-7.267675525,-1.77635683940025E-14,-7.601392651));
#152178=CARTESIAN_POINT('Origin',(-7.330271396,-1.77635683940025E-14,-7.54154487));
#152179=CARTESIAN_POINT('Origin',(-7.520653728,-1.77635683940025E-14,-7.359520724));
#152180=CARTESIAN_POINT('Origin',(-7.862822419,-1.77635683940025E-14,-6.98454017));
#152181=CARTESIAN_POINT('Origin',(-7.862822419,-1.77635683940025E-14,-6.98454017));
#152182=CARTESIAN_POINT('Origin',(-7.919801584,-1.77635683940025E-14,-6.919322268));
#152183=CARTESIAN_POINT('Origin',(-7.976780749,-1.77635683940025E-14,-6.854104366));
#152184=CARTESIAN_POINT('Origin',(-8.150080138,-1.77635683940025E-14,-6.655747255));
#152185=CARTESIAN_POINT('Origin',(-8.457258361,-1.77635683940025E-14,-6.251604497));
#152186=CARTESIAN_POINT('Origin',(-8.457258361,-1.77635683940025E-14,-6.251604497));
#152187=CARTESIAN_POINT('Origin',(-8.508162058,-1.77635683940025E-14,-6.18154157));
#152188=CARTESIAN_POINT('Origin',(-8.559065754,-1.77635683940025E-14,-6.111478643));
#152189=CARTESIAN_POINT('Origin',(-8.713886896,-1.77635683940025E-14,-5.898385622));
#152190=CARTESIAN_POINT('Origin',(-8.983601432,-1.77635683940025E-14,-5.46833458));
#152191=CARTESIAN_POINT('Origin',(-8.983601432,-1.77635683940025E-14,-5.46833458));
#152192=CARTESIAN_POINT('Origin',(-9.028019813,-1.77635683940025E-14,-5.393990734));
#152193=CARTESIAN_POINT('Origin',(-9.072438193,-1.77635683940025E-14,-5.319646888));
#152194=CARTESIAN_POINT('Origin',(-9.20753456,-1.77635683940025E-14,-5.093533656));
#152195=CARTESIAN_POINT('Origin',(-9.437613827,-1.77635683940025E-14,-4.641036849));
#152196=CARTESIAN_POINT('Origin',(-9.437613827,-1.77635683940025E-14,-4.641036849));
#152197=CARTESIAN_POINT('Origin',(-9.475189261,-1.77635683940025E-14,-4.563010656));
#152198=CARTESIAN_POINT('Origin',(-9.512764695,-1.77635683940025E-14,-4.484984463));
#152199=CARTESIAN_POINT('Origin',(-9.627048569,-1.77635683940025E-14,-4.247671553));
#152200=CARTESIAN_POINT('Origin',(-9.815640104,-1.77635683940025E-14,-3.776372218));
#152201=CARTESIAN_POINT('Origin',(-9.815640104,-1.77635683940025E-14,-3.776372218));
#152202=CARTESIAN_POINT('Origin',(-9.846070056,-1.77635683940025E-14,-3.6952919));
#152203=CARTESIAN_POINT('Origin',(-9.876500008,-1.77635683940025E-14,-3.614211582));
#152204=CARTESIAN_POINT('Origin',(-9.969051245,-1.77635683940025E-14,-3.367609695));
#152205=CARTESIAN_POINT('Origin',(-10.114636618,-1.77635683940025E-14,-2.881302458));
#152206=CARTESIAN_POINT('Origin',(-10.114636618,-1.77635683940025E-14,-2.881302458));
#152207=CARTESIAN_POINT('Origin',(-10.137676085,-1.77635683940025E-14,-2.797820826));
#152208=CARTESIAN_POINT('Origin',(-10.160715552,-1.77635683940025E-14,-2.714339193));
#152209=CARTESIAN_POINT('Origin',(-10.230788981,-1.77635683940025E-14,-2.460433825));
#152210=CARTESIAN_POINT('Origin',(-10.332196026,-1.77635683940025E-14,-1.963034146));
#152211=CARTESIAN_POINT('Origin',(-10.332196026,-1.77635683940025E-14,-1.963034146));
#152212=CARTESIAN_POINT('Origin',(-10.347659507,-1.77635683940025E-14,-1.877823344));
#152213=CARTESIAN_POINT('Origin',(-10.363122988,-1.77635683940025E-14,-1.792612542));
#152214=CARTESIAN_POINT('Origin',(-10.41015442,-1.77635683940025E-14,-1.533447988));
#152215=CARTESIAN_POINT('Origin',(-10.466566667,-1.77635683940025E-14,-1.028960636));
#152216=CARTESIAN_POINT('Origin',(-10.466566667,-1.77635683940025E-14,-1.028960636));
#152217=CARTESIAN_POINT('Origin',(-10.474329659,-1.77635683940025E-14,-0.942706732));
#152218=CARTESIAN_POINT('Origin',(-10.482092651,-1.77635683940025E-14,-0.856452827999998));
#152219=CARTESIAN_POINT('Origin',(-10.505703417,-1.77635683940025E-14,-0.594115729));
#152220=CARTESIAN_POINT('Origin',(-10.516666667,-1.77635683940025E-14,-0.0866025400000003));
#152221=CARTESIAN_POINT('Origin',(-10.516666667,-1.77635683940025E-14,-0.0866025400000003));
#152222=CARTESIAN_POINT('Origin',(-10.516666667,-1.77635683940025E-14,2.22044604925031E-15));
#152223=CARTESIAN_POINT('Origin',(-10.516666667,-1.77635683940025E-14,0.0866025400000026));
#152224=CARTESIAN_POINT('Origin',(-10.516666667,-1.77635683940025E-14,0.349999999999999));
#152225=CARTESIAN_POINT('Origin',(-10.48209265,-1.77635683940025E-14,0.856452828000001));
#152226=CARTESIAN_POINT('Origin',(-10.48209265,-1.77635683940025E-14,0.856452828000001));
#152227=CARTESIAN_POINT('Origin',(-10.474329659,-1.77635683940025E-14,0.942706731999998));
#152228=CARTESIAN_POINT('Origin',(-10.466566667,-1.77635683940025E-14,1.028960636));
#152229=CARTESIAN_POINT('Origin',(-10.4429559,-1.77635683940025E-14,1.291297735));
#152230=CARTESIAN_POINT('Origin',(-10.363122987,-1.77635683940025E-14,1.792612542));
#152231=CARTESIAN_POINT('Origin',(-10.363122987,-1.77635683940025E-14,1.792612542));
#152232=CARTESIAN_POINT('Origin',(-10.347659507,-1.77635683940025E-14,1.877823344));
#152233=CARTESIAN_POINT('Origin',(-10.332196026,-1.77635683940025E-14,1.963034146));
#152234=CARTESIAN_POINT('Origin',(-10.285164594,-1.77635683940025E-14,2.2221987));
#152235=CARTESIAN_POINT('Origin',(-10.160715552,-1.77635683940025E-14,2.714339193));
#152236=CARTESIAN_POINT('Origin',(-10.160715552,-1.77635683940025E-14,2.714339193));
#152237=CARTESIAN_POINT('Origin',(-10.137676085,-1.77635683940025E-14,2.797820826));
#152238=CARTESIAN_POINT('Origin',(-10.114636618,-1.77635683940025E-14,2.881302458));
#152239=CARTESIAN_POINT('Origin',(-10.044563189,-1.77635683940025E-14,3.135207827));
#152240=CARTESIAN_POINT('Origin',(-9.876500009,-1.77635683940025E-14,3.614211582));
#152241=CARTESIAN_POINT('Origin',(-9.876500009,-1.77635683940025E-14,3.614211582));
#152242=CARTESIAN_POINT('Origin',(-9.846070056,-1.77635683940025E-14,3.6952919));
#152243=CARTESIAN_POINT('Origin',(-9.815640104,-1.77635683940025E-14,3.776372218));
#152244=CARTESIAN_POINT('Origin',(-9.723088868,-1.77635683940025E-14,4.022974105));
#152245=CARTESIAN_POINT('Origin',(-9.512764695,-1.77635683940025E-14,4.484984464));
#152246=CARTESIAN_POINT('Origin',(-9.512764695,-1.77635683940025E-14,4.484984464));
#152247=CARTESIAN_POINT('Origin',(-9.475189261,-1.77635683940025E-14,4.563010656));
#152248=CARTESIAN_POINT('Origin',(-9.437613827,-1.77635683940025E-14,4.641036849));
#152249=CARTESIAN_POINT('Origin',(-9.323329952,-1.77635683940025E-14,4.87834976));
#152250=CARTESIAN_POINT('Origin',(-9.072438193,-1.77635683940025E-14,5.319646888));
#152251=CARTESIAN_POINT('Origin',(-9.072438193,-1.77635683940025E-14,5.319646888));
#152252=CARTESIAN_POINT('Origin',(-9.028019813,-1.77635683940025E-14,5.393990734));
#152253=CARTESIAN_POINT('Origin',(-8.983601433,-1.77635683940025E-14,5.46833458));
#152254=CARTESIAN_POINT('Origin',(-8.848505066,-1.77635683940025E-14,5.694447812));
#152255=CARTESIAN_POINT('Origin',(-8.559065754,-1.77635683940025E-14,6.111478643));
#152256=CARTESIAN_POINT('Origin',(-8.559065754,-1.77635683940025E-14,6.111478643));
#152257=CARTESIAN_POINT('Origin',(-8.508162058,-1.77635683940025E-14,6.18154157));
#152258=CARTESIAN_POINT('Origin',(-8.457258362,-1.77635683940025E-14,6.251604497));
#152259=CARTESIAN_POINT('Origin',(-8.302437219,-1.77635683940025E-14,6.464697518));
#152260=CARTESIAN_POINT('Origin',(-7.976780749,-1.77635683940025E-14,6.854104366));
#152261=CARTESIAN_POINT('Origin',(-7.976780749,-1.77635683940025E-14,6.854104366));
#152262=CARTESIAN_POINT('Origin',(-7.919801584,-1.77635683940025E-14,6.919322268));
#152263=CARTESIAN_POINT('Origin',(-7.862822419,-1.77635683940025E-14,6.98454017));
#152264=CARTESIAN_POINT('Origin',(-7.68952303,-1.77635683940025E-14,7.182897281));
#152265=CARTESIAN_POINT('Origin',(-7.330271397,-1.77635683940025E-14,7.54154487));
#152266=CARTESIAN_POINT('Origin',(-7.330271397,-1.77635683940025E-14,7.54154487));
#152267=CARTESIAN_POINT('Origin',(-7.267675525,-1.77635683940025E-14,7.601392651));
#152268=CARTESIAN_POINT('Origin',(-7.205079654,-1.77635683940025E-14,7.661240432));
#152269=CARTESIAN_POINT('Origin',(-7.014697323,-1.77635683940025E-14,7.843264578));
#152270=CARTESIAN_POINT('Origin',(-6.624743009,-1.77635683940025E-14,8.16826529));
#152271=CARTESIAN_POINT('Origin',(-6.624743009,-1.77635683940025E-14,8.16826529));
#152272=CARTESIAN_POINT('Origin',(-6.557034416,-1.77635683940025E-14,8.222261091));
#152273=CARTESIAN_POINT('Origin',(-6.489325824,-1.77635683940025E-14,8.276256891));
#152274=CARTESIAN_POINT('Origin',(-6.283393397,-1.77635683940025E-14,8.440482521));
#152275=CARTESIAN_POINT('Origin',(-5.865876086,-1.77635683940025E-14,8.72921964));
#152276=CARTESIAN_POINT('Origin',(-5.865876086,-1.77635683940025E-14,8.72921964));
#152277=CARTESIAN_POINT('Origin',(-5.793599922,-1.77635683940025E-14,8.776928718));
#152278=CARTESIAN_POINT('Origin',(-5.721323758,-1.77635683940025E-14,8.824637796));
#152279=CARTESIAN_POINT('Origin',(-5.501499283,-1.77635683940025E-14,8.969742662));
#152280=CARTESIAN_POINT('Origin',(-5.059780577,-1.77635683940025E-14,9.219891447));
#152281=CARTESIAN_POINT('Origin',(-5.059780577,-1.77635683940025E-14,9.219891447));
#152282=CARTESIAN_POINT('Origin',(-4.983518767,-1.77635683940025E-14,9.260929677));
#152283=CARTESIAN_POINT('Origin',(-4.907256957,-1.77635683940025E-14,9.301967907));
#152284=CARTESIAN_POINT('Origin',(-4.675310331,-1.77635683940025E-14,9.426783709));
#152285=CARTESIAN_POINT('Origin',(-4.212946691,-1.77635683940025E-14,9.636330108));
#152286=CARTESIAN_POINT('Origin',(-4.212946691,-1.77635683940025E-14,9.636330108));
#152287=CARTESIAN_POINT('Origin',(-4.13331325,-1.77635683940025E-14,9.670367075));
#152288=CARTESIAN_POINT('Origin',(-4.053679809,-1.77635683940025E-14,9.704404041));
#152289=CARTESIAN_POINT('Origin',(-3.811478529,-1.77635683940025E-14,9.807925836));
#152290=CARTESIAN_POINT('Origin',(-3.332192635,-1.77635683940025E-14,9.975182706));
#152291=CARTESIAN_POINT('Origin',(-3.332192635,-1.77635683940025E-14,9.975182706));
#152292=CARTESIAN_POINT('Origin',(-3.249828724,-1.77635683940025E-14,10.001944363));
#152293=CARTESIAN_POINT('Origin',(-3.167464814,-1.77635683940025E-14,10.02870602));
#152294=CARTESIAN_POINT('Origin',(-2.916958943,-1.77635683940025E-14,10.110100311));
#152295=CARTESIAN_POINT('Origin',(-2.424609723,-1.77635683940025E-14,10.233720998));
#152296=CARTESIAN_POINT('Origin',(-2.424609723,-1.77635683940025E-14,10.233720998));
#152297=CARTESIAN_POINT('Origin',(-2.340178489,-1.77635683940025E-14,10.252991876));
#152298=CARTESIAN_POINT('Origin',(-2.255747255,-1.77635683940025E-14,10.272262754));
#152299=CARTESIAN_POINT('Origin',(-1.99895372,-1.77635683940025E-14,10.330874203));
#152300=CARTESIAN_POINT('Origin',(-1.497505279,-1.77635683940025E-14,10.409863386));
#152301=CARTESIAN_POINT('Origin',(-1.497505279,-1.77635683940025E-14,10.409863386));
#152302=CARTESIAN_POINT('Origin',(-1.411686512,-1.77635683940025E-14,10.421488328));
#152303=CARTESIAN_POINT('Origin',(-1.325867745,-1.77635683940025E-14,10.43311327));
#152304=CARTESIAN_POINT('Origin',(-1.064854096,-1.77635683940025E-14,10.468469971));
#152305=CARTESIAN_POINT('Origin',(-0.558343802999999,-1.77635683940025E-14,
10.502191675));
#152306=CARTESIAN_POINT('Origin',(-0.558343802999999,-1.77635683940025E-14,
10.502191675));
#152307=CARTESIAN_POINT('Origin',(-0.471828465999998,-1.77635683940025E-14,
10.506077083));
#152308=CARTESIAN_POINT('Origin',(-0.385313128999999,-1.77635683940025E-14,
10.509962491));
#152309=CARTESIAN_POINT('Origin',(-0.122180893,-1.77635683940025E-14,10.521779774));
#152310=CARTESIAN_POINT('Origin',(0.385313128000001,-1.77635683940025E-14,
10.509962491));
#152311=CARTESIAN_POINT('Origin',(0.385313128000001,-1.77635683940025E-14,
10.509962491));
#152312=CARTESIAN_POINT('Origin',(0.471828466000001,-1.77635683940025E-14,
10.506077083));
#152313=CARTESIAN_POINT('Origin',(0.558343803000001,-1.77635683940025E-14,
10.502191675));
#152314=CARTESIAN_POINT('Origin',(0.821476039000001,-1.77635683940025E-14,
10.490374393));
#152315=CARTESIAN_POINT('Origin',(1.325867745,-1.77635683940025E-14,10.43311327));
#152316=CARTESIAN_POINT('Origin',(1.325867745,-1.77635683940025E-14,10.43311327));
#152317=CARTESIAN_POINT('Origin',(1.411686512,-1.77635683940025E-14,10.421488328));
#152318=CARTESIAN_POINT('Origin',(1.497505279,-1.77635683940025E-14,10.409863386));
#152319=CARTESIAN_POINT('Origin',(1.758518929,-1.77635683940025E-14,10.374506685));
#152320=CARTESIAN_POINT('Origin',(2.255747255,-1.77635683940025E-14,10.272262755));
#152321=CARTESIAN_POINT('Origin',(2.255747255,-1.77635683940025E-14,10.272262755));
#152322=CARTESIAN_POINT('Origin',(2.340178489,-1.77635683940025E-14,10.252991876));
#152323=CARTESIAN_POINT('Origin',(2.424609723,-1.77635683940025E-14,10.233720998));
#152324=CARTESIAN_POINT('Origin',(2.681403258,-1.77635683940025E-14,10.17510955));
#152325=CARTESIAN_POINT('Origin',(3.167464814,-1.77635683940025E-14,10.02870602));
#152326=CARTESIAN_POINT('Origin',(3.167464814,-1.77635683940025E-14,10.02870602));
#152327=CARTESIAN_POINT('Origin',(3.249828724,-1.77635683940025E-14,10.001944363));
#152328=CARTESIAN_POINT('Origin',(3.332192634,-1.77635683940025E-14,9.975182706));
#152329=CARTESIAN_POINT('Origin',(3.582698505,-1.77635683940025E-14,9.893788415));
#152330=CARTESIAN_POINT('Origin',(4.053679809,-1.77635683940025E-14,9.704404041));
#152331=CARTESIAN_POINT('Origin',(4.053679809,-1.77635683940025E-14,9.704404041));
#152332=CARTESIAN_POINT('Origin',(4.13331325,-1.77635683940025E-14,9.670367075));
#152333=CARTESIAN_POINT('Origin',(4.212946691,-1.77635683940025E-14,9.636330109));
#152334=CARTESIAN_POINT('Origin',(4.45514797,-1.77635683940025E-14,9.532808314));
#152335=CARTESIAN_POINT('Origin',(4.907256957,-1.77635683940025E-14,9.301967907));
#152336=CARTESIAN_POINT('Origin',(4.907256957,-1.77635683940025E-14,9.301967907));
#152337=CARTESIAN_POINT('Origin',(4.983518767,-1.77635683940025E-14,9.260929677));
#152338=CARTESIAN_POINT('Origin',(5.059780577,-1.77635683940025E-14,9.219891447));
#152339=CARTESIAN_POINT('Origin',(5.291727203,-1.77635683940025E-14,9.095075645));
#152340=CARTESIAN_POINT('Origin',(5.721323758,-1.77635683940025E-14,8.824637796));
#152341=CARTESIAN_POINT('Origin',(5.721323758,-1.77635683940025E-14,8.824637796));
#152342=CARTESIAN_POINT('Origin',(5.793599922,-1.77635683940025E-14,8.776928718));
#152343=CARTESIAN_POINT('Origin',(5.865876086,-1.77635683940025E-14,8.72921964));
#152344=CARTESIAN_POINT('Origin',(6.08570056,-1.77635683940025E-14,8.584114775));
#152345=CARTESIAN_POINT('Origin',(6.489325824,-1.77635683940025E-14,8.276256891));
#152346=CARTESIAN_POINT('Origin',(6.489325824,-1.77635683940025E-14,8.276256891));
#152347=CARTESIAN_POINT('Origin',(6.557034416,-1.77635683940025E-14,8.222261091));
#152348=CARTESIAN_POINT('Origin',(6.624743009,-1.77635683940025E-14,8.16826529));
#152349=CARTESIAN_POINT('Origin',(6.830675435,-1.77635683940025E-14,8.00403966));
#152350=CARTESIAN_POINT('Origin',(7.205079654,-1.77635683940025E-14,7.661240432));
#152351=CARTESIAN_POINT('Origin',(7.205079654,-1.77635683940025E-14,7.661240432));
#152352=CARTESIAN_POINT('Origin',(7.267675525,-1.77635683940025E-14,7.601392651));
#152353=CARTESIAN_POINT('Origin',(7.330271396,-1.77635683940025E-14,7.54154487));
#152354=CARTESIAN_POINT('Origin',(7.520653728,-1.77635683940025E-14,7.359520724));
#152355=CARTESIAN_POINT('Origin',(7.862822419,-1.77635683940025E-14,6.98454017));
#152356=CARTESIAN_POINT('Origin',(7.862822419,-1.77635683940025E-14,6.98454017));
#152357=CARTESIAN_POINT('Origin',(7.919801584,-1.77635683940025E-14,6.919322268));
#152358=CARTESIAN_POINT('Origin',(7.976780749,-1.77635683940025E-14,6.854104366));
#152359=CARTESIAN_POINT('Origin',(8.150080138,-1.77635683940025E-14,6.655747255));
#152360=CARTESIAN_POINT('Origin',(8.457258361,-1.77635683940025E-14,6.251604497));
#152361=CARTESIAN_POINT('Origin',(8.457258361,-1.77635683940025E-14,6.251604497));
#152362=CARTESIAN_POINT('Origin',(8.508162058,-1.77635683940025E-14,6.18154157));
#152363=CARTESIAN_POINT('Origin',(8.559065754,-1.77635683940025E-14,6.111478643));
#152364=CARTESIAN_POINT('Origin',(8.713886896,-1.77635683940025E-14,5.898385622));
#152365=CARTESIAN_POINT('Origin',(8.983601432,-1.77635683940025E-14,5.46833458));
#152366=CARTESIAN_POINT('Origin',(8.983601432,-1.77635683940025E-14,5.46833458));
#152367=CARTESIAN_POINT('Origin',(9.028019813,-1.77635683940025E-14,5.393990734));
#152368=CARTESIAN_POINT('Origin',(9.072438193,-1.77635683940025E-14,5.319646888));
#152369=CARTESIAN_POINT('Origin',(9.20753456,-1.77635683940025E-14,5.093533656));
#152370=CARTESIAN_POINT('Origin',(9.437613827,-1.77635683940025E-14,4.641036849));
#152371=CARTESIAN_POINT('Origin',(9.437613827,-1.77635683940025E-14,4.641036849));
#152372=CARTESIAN_POINT('Origin',(9.475189261,-1.77635683940025E-14,4.563010656));
#152373=CARTESIAN_POINT('Origin',(9.512764695,-1.77635683940025E-14,4.484984463));
#152374=CARTESIAN_POINT('Origin',(9.627048569,-1.77635683940025E-14,4.247671553));
#152375=CARTESIAN_POINT('Origin',(9.815640104,-1.77635683940025E-14,3.776372218));
#152376=CARTESIAN_POINT('Origin',(9.815640104,-1.77635683940025E-14,3.776372218));
#152377=CARTESIAN_POINT('Origin',(9.846070056,-1.77635683940025E-14,3.6952919));
#152378=CARTESIAN_POINT('Origin',(9.876500008,-1.77635683940025E-14,3.614211582));
#152379=CARTESIAN_POINT('Origin',(9.969051245,-1.77635683940025E-14,3.367609695));
#152380=CARTESIAN_POINT('Origin',(10.114636618,-1.77635683940025E-14,2.881302458));
#152381=CARTESIAN_POINT('Origin',(10.114636618,-1.77635683940025E-14,2.881302458));
#152382=CARTESIAN_POINT('Origin',(10.137676085,-1.77635683940025E-14,2.797820826));
#152383=CARTESIAN_POINT('Origin',(10.160715552,-1.77635683940025E-14,2.714339193));
#152384=CARTESIAN_POINT('Origin',(10.230788981,-1.77635683940025E-14,2.460433825));
#152385=CARTESIAN_POINT('Origin',(10.332196026,-1.77635683940025E-14,1.963034146));
#152386=CARTESIAN_POINT('Origin',(10.332196026,-1.77635683940025E-14,1.963034146));
#152387=CARTESIAN_POINT('Origin',(10.347659507,-1.77635683940025E-14,1.877823344));
#152388=CARTESIAN_POINT('Origin',(10.363122988,-1.77635683940025E-14,1.792612542));
#152389=CARTESIAN_POINT('Origin',(10.41015442,-1.77635683940025E-14,1.533447988));
#152390=CARTESIAN_POINT('Origin',(10.466566667,-1.77635683940025E-14,1.028960636));
#152391=CARTESIAN_POINT('Origin',(10.466566667,-1.77635683940025E-14,1.028960636));
#152392=CARTESIAN_POINT('Origin',(10.474329659,-1.77635683940025E-14,0.942706731999998));
#152393=CARTESIAN_POINT('Origin',(10.482092651,-1.77635683940025E-14,0.856452828000001));
#152394=CARTESIAN_POINT('Origin',(10.505703417,-1.77635683940025E-14,0.594115729));
#152395=CARTESIAN_POINT('Origin',(-6.,4.49999999999998,2.22044604925031E-15));
#152396=CARTESIAN_POINT('',(-7.,4.49999999999998,2.34291072916505E-15));
#152397=CARTESIAN_POINT('Origin',(-6.,4.49999999999998,2.22044604925031E-15));
#152398=CARTESIAN_POINT('',(-7.,7.49999999999998,2.34291072916505E-15));
#152399=CARTESIAN_POINT('',(-7.,4.49999999999998,2.34291072916505E-15));
#152400=CARTESIAN_POINT('Origin',(-6.,7.49999999999998,2.22044604925031E-15));
#152401=CARTESIAN_POINT('Origin',(6.,4.49999999999998,2.22044604925031E-15));
#152402=CARTESIAN_POINT('',(5.,4.49999999999998,2.34291072916505E-15));
#152403=CARTESIAN_POINT('Origin',(6.,4.49999999999998,2.22044604925031E-15));
#152404=CARTESIAN_POINT('',(5.,7.49999999999998,2.34291072916505E-15));
#152405=CARTESIAN_POINT('',(5.,4.49999999999998,2.34291072916505E-15));
#152406=CARTESIAN_POINT('Origin',(6.,7.49999999999998,2.22044604925031E-15));
#152407=CARTESIAN_POINT('Origin',(-6.,2.39999999999998,2.22044604925031E-15));
#152408=CARTESIAN_POINT('',(-7.6,2.49999999999998,2.41638953711389E-15));
#152409=CARTESIAN_POINT('Origin',(-6.,2.49999999999998,2.22044604925031E-15));
#152410=CARTESIAN_POINT('',(-7.5,2.39999999999998,2.40414306912242E-15));
#152411=CARTESIAN_POINT('Origin',(-7.6,2.39999999999998,2.41638953711389E-15));
#152412=CARTESIAN_POINT('Origin',(-6.,2.39999999999998,2.22044604925031E-15));
#152413=CARTESIAN_POINT('Origin',(6.,2.39999999999998,2.22044604925031E-15));
#152414=CARTESIAN_POINT('',(4.4,2.49999999999998,2.41638953711389E-15));
#152415=CARTESIAN_POINT('Origin',(6.,2.49999999999998,2.22044604925031E-15));
#152416=CARTESIAN_POINT('',(4.5,2.39999999999998,2.40414306912242E-15));
#152417=CARTESIAN_POINT('Origin',(4.4,2.39999999999998,2.41638953711389E-15));
#152418=CARTESIAN_POINT('Origin',(6.,2.39999999999998,2.22044604925031E-15));
#152419=CARTESIAN_POINT('Origin',(2.22044604925031E-15,5.39999999999998,
2.22044604925031E-15));
#152420=CARTESIAN_POINT('',(1.5,5.39999999999998,2.40414306912242E-15));
#152421=CARTESIAN_POINT('',(-1.5,5.39999999999998,2.40414306912242E-15));
#152422=CARTESIAN_POINT('Origin',(2.22044604925031E-15,5.39999999999998,
2.22044604925031E-15));
#152423=CARTESIAN_POINT('',(1.7,5.19999999999998,2.42863600510536E-15));
#152424=CARTESIAN_POINT('Origin',(1.7,5.39999999999998,2.42863600510536E-15));
#152425=CARTESIAN_POINT('Origin',(2.22044604925031E-15,5.19999999999998,
2.22044604925031E-15));
#152426=CARTESIAN_POINT('Origin',(2.22044604925031E-15,5.39999999999998,
2.22044604925031E-15));
#152427=CARTESIAN_POINT('Origin',(2.22044604925031E-15,7.50005079999998,
2.22044604925031E-15));
#152428=CARTESIAN_POINT('',(-1.5,7.50005079999998,2.40414306912242E-15));
#152429=CARTESIAN_POINT('Origin',(2.22044604925031E-15,7.50005079999998,
2.22044604925031E-15));
#152430=CARTESIAN_POINT('',(-1.7,7.70005079999998,2.42863600510536E-15));
#152431=CARTESIAN_POINT('Origin',(-1.7,7.50005079999998,2.42863600510536E-15));
#152432=CARTESIAN_POINT('Origin',(2.22044604925031E-15,7.70005079999998,
2.22044604925031E-15));
#152433=CARTESIAN_POINT('Origin',(2.22044604925031E-15,7.50005079999998,
2.22044604925031E-15));
#152434=CARTESIAN_POINT('',(-2.8,7.70005079999998,2.56334715301157E-15));
#152435=CARTESIAN_POINT('Origin',(2.22044604925031E-15,7.70005079999998,
2.22044604925031E-15));
#152436=CARTESIAN_POINT('',(-3.,7.50005079999998,2.58784008899452E-15));
#152437=CARTESIAN_POINT('Origin',(-2.8,7.50005079999998,2.56334715301157E-15));
#152438=CARTESIAN_POINT('',(3.,7.50005079999998,2.58784008899452E-15));
#152439=CARTESIAN_POINT('Origin',(2.22044604925031E-15,7.50005079999998,
2.22044604925031E-15));
#152440=CARTESIAN_POINT('Origin',(2.22044604925031E-15,7.50005079999998,
2.22044604925031E-15));
#152441=CARTESIAN_POINT('Origin',(6.266666667,2.69999999999998,2.639865316));
#152442=CARTESIAN_POINT('',(6.4000000003749,2.69999999999998,2.26274169893964));
#152443=CARTESIAN_POINT('',(6.63529411786042,2.69999999999998,2.79515151133333));
#152444=CARTESIAN_POINT('Origin',(6.266666667,2.69999999999998,2.639865316));
#152445=CARTESIAN_POINT('',(6.466666667,2.49999999999998,2.074179891));
#152446=CARTESIAN_POINT('Origin',(6.466666667,2.69999999999998,2.074179891));
#152447=CARTESIAN_POINT('',(6.819607843,2.49999999999998,2.872794609));
#152448=CARTESIAN_POINT('Origin',(6.266666667,2.49999999999998,2.639865316));
#152449=CARTESIAN_POINT('Origin',(6.819607843,2.69999999999998,2.872794609));
#152450=CARTESIAN_POINT('Origin',(6.266666667,2.69999999999998,-2.639865316));
#152451=CARTESIAN_POINT('',(6.63529411787831,2.69999999999998,-2.79515151154086));
#152452=CARTESIAN_POINT('',(6.400000001,2.69999999999998,-2.262741699));
#152453=CARTESIAN_POINT('Origin',(6.266666667,2.69999999999998,-2.639865316));
#152454=CARTESIAN_POINT('',(6.819607843,2.49999999999998,-2.872794609));
#152455=CARTESIAN_POINT('Origin',(6.819607843,2.69999999999998,-2.87279461));
#152456=CARTESIAN_POINT('',(6.466666667,2.49999999999998,-2.07417989));
#152457=CARTESIAN_POINT('Origin',(6.266666667,2.49999999999998,-2.639865316));
#152458=CARTESIAN_POINT('Origin',(6.466666668,2.69999999999998,-2.074179889));
#152459=CARTESIAN_POINT('Origin',(2.22044604925031E-15,2.89999999999998,
2.22044604925031E-15));
#152460=CARTESIAN_POINT('',(-3.9,2.49999999999998,2.69805830091778E-15));
#152461=CARTESIAN_POINT('Origin',(2.22044604925031E-15,2.49999999999998,
2.22044604925031E-15));
#152462=CARTESIAN_POINT('',(-3.5,2.89999999999998,2.64907242895189E-15));
#152463=CARTESIAN_POINT('Origin',(-3.9,2.89999999999998,2.69805830091778E-15));
#152464=CARTESIAN_POINT('',(3.5,2.89999999999998,2.64907242895189E-15));
#152465=CARTESIAN_POINT('Origin',(2.22044604925031E-15,2.89999999999998,
2.22044604925031E-15));
#152466=CARTESIAN_POINT('Origin',(2.22044604925031E-15,2.89999999999998,
2.22044604925031E-15));
#152467=CARTESIAN_POINT('Origin',(-6.,-0.900000000000018,2.22044604925031E-15));
#152468=CARTESIAN_POINT('',(-4.9,-1.30000000000002,2.35515719715652E-15));
#152469=CARTESIAN_POINT('Origin',(-6.,-1.30000000000002,2.22044604925031E-15));
#152470=CARTESIAN_POINT('',(-4.5,-0.900000000000018,2.40414306912242E-15));
#152471=CARTESIAN_POINT('Origin',(-4.9,-0.900000000000018,2.35515719715652E-15));
#152472=CARTESIAN_POINT('',(-7.5,-0.900000000000018,2.40414306912242E-15));
#152473=CARTESIAN_POINT('Origin',(-6.,-0.900000000000018,2.22044604925031E-15));
#152474=CARTESIAN_POINT('Origin',(-6.,-0.900000000000018,2.22044604925031E-15));
#152475=CARTESIAN_POINT('Origin',(6.,-0.900000000000018,2.22044604925031E-15));
#152476=CARTESIAN_POINT('',(7.1,-1.30000000000002,2.35515719715652E-15));
#152477=CARTESIAN_POINT('Origin',(6.,-1.30000000000002,2.22044604925031E-15));
#152478=CARTESIAN_POINT('',(7.5,-0.900000000000018,2.40414306912242E-15));
#152479=CARTESIAN_POINT('Origin',(7.1,-0.900000000000018,2.35515719715652E-15));
#152480=CARTESIAN_POINT('',(4.5,-0.900000000000018,2.40414306912242E-15));
#152481=CARTESIAN_POINT('Origin',(6.,-0.900000000000018,2.22044604925031E-15));
#152482=CARTESIAN_POINT('Origin',(6.,-0.900000000000018,2.22044604925031E-15));
#152483=CARTESIAN_POINT('Origin',(-6.266666667,4.99999999999998,2.639865316));
#152484=CARTESIAN_POINT('',(-6.6352941178783,2.69999999999998,2.79515151154086));
#152485=CARTESIAN_POINT('',(-6.40000000011872,2.69999999999998,2.2627416986642));
#152486=CARTESIAN_POINT('Origin',(-6.266666667,2.69999999999998,2.639865316));
#152487=CARTESIAN_POINT('',(-6.4,4.99999999999998,2.262741699));
#152488=CARTESIAN_POINT('',(-6.4,4.99999999999998,2.262741699));
#152489=CARTESIAN_POINT('',(-6.63529411796584,4.99999999999998,2.79515151131895));
#152490=CARTESIAN_POINT('Origin',(-6.266666667,4.99999999999998,2.639865316));
#152491=CARTESIAN_POINT('',(-6.635294118,4.99999999999998,2.795151512));
#152492=CARTESIAN_POINT('Origin',(-6.266666667,4.99999999999998,-2.639865316));
#152493=CARTESIAN_POINT('',(-6.40000000060197,2.70000000049998,-2.26274169880154));
#152494=CARTESIAN_POINT('',(-6.63529411786042,2.69999999999998,-2.79515151133332));
#152495=CARTESIAN_POINT('Origin',(-6.266666667,2.69999999999998,-2.639865316));
#152496=CARTESIAN_POINT('',(-6.63529411796585,4.99999999999998,-2.79515151131894));
#152497=CARTESIAN_POINT('',(-6.635294118,4.99999999999998,-2.795151512));
#152498=CARTESIAN_POINT('',(-6.4,4.99999999999998,-2.262741699));
#152499=CARTESIAN_POINT('Origin',(-6.266666667,4.99999999999998,-2.639865316));
#152500=CARTESIAN_POINT('',(-6.4,4.99999999999998,-2.262741699));
#152501=CARTESIAN_POINT('Origin',(2.22044604925031E-15,5.19999999999998,
2.22044604925031E-15));
#152502=CARTESIAN_POINT('',(3.5,5.19999999999998,2.64907242895189E-15));
#152503=CARTESIAN_POINT('Origin',(2.22044604925031E-15,5.19999999999998,
2.22044604925031E-15));
#152504=CARTESIAN_POINT('',(3.5,5.19999999999998,2.64907242895189E-15));
#152505=CARTESIAN_POINT('Origin',(-6.,-1.30000000000002,2.22044604925031E-15));
#152506=CARTESIAN_POINT('',(-7.5,-1.30000000000002,2.40414306912242E-15));
#152507=CARTESIAN_POINT('Origin',(6.,-1.30000000000002,2.22044604925031E-15));
#152508=CARTESIAN_POINT('',(4.5,-1.30000000000002,2.40414306912242E-15));
#152509=CARTESIAN_POINT('Origin',(2.22044604925031E-15,7.70005079999998,
2.22044604925031E-15));
#152510=CARTESIAN_POINT('',(3.,7.49999999999998,2.58784008899452E-15));
#152511=CARTESIAN_POINT('Origin',(2.22044604925031E-15,7.49999999999998,
2.22044604925031E-15));
#152512=CARTESIAN_POINT('',(3.,7.70005079999998,2.58784008899452E-15));
#152513=CARTESIAN_POINT('Origin',(-1.016576292,2.49999999999998,-8.632506096));
#152514=CARTESIAN_POINT('',(2.65852674,2.49999999999998,-8.20399973));
#152515=CARTESIAN_POINT('',(2.60381795543899,2.49999999999998,-9.3958837827716));
#152516=CARTESIAN_POINT('Origin',(-1.016576292,2.49999999999998,-8.632506096));
#152517=CARTESIAN_POINT('',(2.60381795543899,7.49999999999998,-9.3958837827716));
#152518=CARTESIAN_POINT('',(2.603817955,2.49999999999998,-9.395883783));
#152519=CARTESIAN_POINT('',(2.65852674,7.49999999999998,-8.20399973));
#152520=CARTESIAN_POINT('Origin',(-1.016576292,7.49999999999998,-8.632506096));
#152521=CARTESIAN_POINT('',(2.65852674,2.49999999999998,-8.20399973));
#152522=CARTESIAN_POINT('Origin',(0.456946844000001,2.49999999999998,-8.680137582));
#152523=CARTESIAN_POINT('',(4.006768937,2.49999999999998,-7.636699463));
#152524=CARTESIAN_POINT('',(4.154276471,2.49999999999998,-8.820685177));
#152525=CARTESIAN_POINT('Origin',(0.456946844000001,2.49999999999998,-8.680137582));
#152526=CARTESIAN_POINT('',(4.154276471,7.49999999999998,-8.820685177));
#152527=CARTESIAN_POINT('',(4.154276471,2.49999999999998,-8.820685177));
#152528=CARTESIAN_POINT('',(4.006768937,7.49999999999998,-7.636699463));
#152529=CARTESIAN_POINT('Origin',(0.456946844000001,7.49999999999998,-8.680137582));
#152530=CARTESIAN_POINT('',(4.006768937,2.49999999999998,-7.636699463));
#152531=CARTESIAN_POINT('Origin',(-0.280826403999999,2.49999999999998,8.687619086));
#152532=CARTESIAN_POINT('',(3.391264282,2.49999999999998,9.141215815));
#152533=CARTESIAN_POINT('',(3.34469714851111,2.49999999999998,7.94898590903151));
#152534=CARTESIAN_POINT('Origin',(-0.280826403999999,2.49999999999998,8.687619086));
#152535=CARTESIAN_POINT('',(3.34469714851111,7.49999999999998,7.94898590903151));
#152536=CARTESIAN_POINT('',(3.344697148,2.49999999999998,7.948985909));
#152537=CARTESIAN_POINT('',(3.391264282,7.49999999999998,9.141215815));
#152538=CARTESIAN_POINT('Origin',(-0.280826403999999,7.49999999999998,8.687619086));
#152539=CARTESIAN_POINT('',(3.391264282,7.49999999999998,9.141215815));
#152540=CARTESIAN_POINT('Origin',(-1.745001724,2.49999999999998,8.515195702));
#152541=CARTESIAN_POINT('',(1.797611062,2.49999999999998,9.582854192));
#152542=CARTESIAN_POINT('',(1.953201586,2.49999999999998,8.399903545));
#152543=CARTESIAN_POINT('Origin',(-1.745001724,2.49999999999998,8.515195702));
#152544=CARTESIAN_POINT('',(1.953201586,7.49999999999998,8.399903545));
#152545=CARTESIAN_POINT('',(1.953201586,2.49999999999998,8.399903545));
#152546=CARTESIAN_POINT('',(1.797611062,7.49999999999998,9.582854192));
#152547=CARTESIAN_POINT('Origin',(-1.745001724,7.49999999999998,8.515195702));
#152548=CARTESIAN_POINT('',(1.797611062,7.49999999999998,9.582854192));
#152549=CARTESIAN_POINT('Origin',(2.22044604925031E-15,2.29994919999998,
2.22044604925031E-15));
#152550=CARTESIAN_POINT('',(-1.5,2.29994919999998,2.40414306912242E-15));
#152551=CARTESIAN_POINT('Origin',(2.22044604925031E-15,2.49999999999998,
2.22044604925031E-15));
#152552=CARTESIAN_POINT('',(8.603650246,2.49999999999998,-0.592096652999998));
#152553=CARTESIAN_POINT('',(9.689187855,2.49999999999998,-1.087262023));
#152554=CARTESIAN_POINT('Origin',(7.630970629,2.49999999999998,-4.161955804));
#152555=CARTESIAN_POINT('',(8.622868801,2.49999999999998,-0.139676895));
#152556=CARTESIAN_POINT('Origin',(2.22044604925031E-15,2.49999999999998,
2.22044604925031E-15));
#152557=CARTESIAN_POINT('',(9.746488706,2.49999999999998,0.261644615999999));
#152558=CARTESIAN_POINT('Origin',(7.956438479,2.49999999999998,3.499810792));
#152559=CARTESIAN_POINT('',(9.733565882,2.49999999999998,0.565857946999999));
#152560=CARTESIAN_POINT('Origin',(2.22044604925031E-15,2.49999999999998,
2.22044604925031E-15));
#152561=CARTESIAN_POINT('',(8.579959389,2.49999999999998,0.870444068000003));
#152562=CARTESIAN_POINT('Origin',(8.224580008,2.49999999999998,-2.812449563));
#152563=CARTESIAN_POINT('',(8.522442193,2.49999999999998,1.31960413));
#152564=CARTESIAN_POINT('Origin',(2.22044604925031E-15,2.49999999999998,
2.22044604925031E-15));
#152565=CARTESIAN_POINT('',(9.562076184,2.49999999999998,1.905045682));
#152566=CARTESIAN_POINT('Origin',(7.25052146,2.49999999999998,4.794113829));
#152567=CARTESIAN_POINT('',(9.497926941,2.49999999999998,2.202699214));
#152568=CARTESIAN_POINT('Origin',(2.22044604925031E-15,2.49999999999998,
2.22044604925031E-15));
#152569=CARTESIAN_POINT('',(8.309438723,2.49999999999998,2.307943698));
#152570=CARTESIAN_POINT('Origin',(8.581583195,2.49999999999998,-1.382034268));
#152571=CARTESIAN_POINT('',(8.17684044,2.49999999999998,2.740922548));
#152572=CARTESIAN_POINT('Origin',(2.22044604925031E-15,2.49999999999998,
2.22044604925031E-15));
#152573=CARTESIAN_POINT('',(9.10258013994849,2.49999999999998,3.49364205338694));
#152574=CARTESIAN_POINT('Origin',(6.33602014,2.49999999999998,5.950498941));
#152575=CARTESIAN_POINT('',(8.989049934,2.49999999999998,3.776172836));
#152576=CARTESIAN_POINT('Origin',(2.22044604925031E-15,2.49999999999998,
2.22044604925031E-15));
#152577=CARTESIAN_POINT('',(7.799870633,2.49999999999998,3.679047989));
#152578=CARTESIAN_POINT('Origin',(8.691709858,2.49999999999998,0.088139637000002));
#152579=CARTESIAN_POINT('',(7.596005875,2.49999999999998,4.083389615));
#152580=CARTESIAN_POINT('Origin',(2.22044604925031E-15,2.49999999999998,
2.22044604925031E-15));
#152581=CARTESIAN_POINT('',(8.381219438,2.49999999999998,4.981732704));
#152582=CARTESIAN_POINT('Origin',(5.239243055,2.49999999999998,6.935699032));
#152583=CARTESIAN_POINT('',(8.221574327,2.49999999999998,5.24101284));
#152584=CARTESIAN_POINT('Origin',(2.22044604925031E-15,2.49999999999998,
2.22044604925031E-15));
#152585=CARTESIAN_POINT('',(7.065914466,2.49999999999998,4.944312769));
#152586=CARTESIAN_POINT('Origin',(8.551791853,2.49999999999998,1.555777924));
#152587=CARTESIAN_POINT('',(6.796648051,2.49999999999998,5.308384996));
#152588=CARTESIAN_POINT('Origin',(2.22044604925031E-15,2.49999999999998,
2.22044604925031E-15));
#152589=CARTESIAN_POINT('',(7.418746313,2.49999999999998,6.326507974));
#152590=CARTESIAN_POINT('Origin',(3.991742488,2.49999999999998,7.721371689));
#152591=CARTESIAN_POINT('',(7.217578995,2.49999999999998,6.555078448));
#152592=CARTESIAN_POINT('Origin',(2.22044604925031E-15,2.49999999999998,
2.22044604925031E-15));
#152593=CARTESIAN_POINT('',(6.128684805,2.49999999999998,6.067338672));
#152594=CARTESIAN_POINT('Origin',(8.165854367,2.49999999999998,2.978659314));
#152595=CARTESIAN_POINT('',(5.801763037,2.49999999999998,6.380667807));
#152596=CARTESIAN_POINT('Origin',(2.22044604925031E-15,2.49999999999998,
2.22044604925031E-15));
#152597=CARTESIAN_POINT('',(6.242849363,2.49999999999998,7.489281129));
#152598=CARTESIAN_POINT('Origin',(2.629406756,2.49999999999998,8.284914542));
#152599=CARTESIAN_POINT('',(6.005947057,2.49999999999998,7.680566382));
#152600=CARTESIAN_POINT('Origin',(2.22044604925031E-15,2.49999999999998,
2.22044604925031E-15));
#152601=CARTESIAN_POINT('',(5.015144041,2.49999999999998,7.015818288));
#152602=CARTESIAN_POINT('Origin',(7.545000119,2.49999999999998,4.315850098));
#152603=CARTESIAN_POINT('',(4.639971864,2.49999999999998,7.269390422));
#152604=CARTESIAN_POINT('Origin',(2.22044604925031E-15,2.49999999999998,
2.22044604925031E-15));
#152605=CARTESIAN_POINT('',(4.887357004,2.49999999999998,8.436601301));
#152606=CARTESIAN_POINT('Origin',(1.19142778,2.49999999999998,8.610115487));
#152607=CARTESIAN_POINT('',(4.621534957,2.49999999999998,8.585098406));
#152608=CARTESIAN_POINT('Origin',(2.22044604925031E-15,2.49999999999998,
2.22044604925031E-15));
#152609=CARTESIAN_POINT('',(3.757326714,2.49999999999998,7.762465586));
#152610=CARTESIAN_POINT('Origin',(6.707089953,2.49999999999998,5.528881732));
#152611=CARTESIAN_POINT('Origin',(2.22044604925031E-15,2.49999999999998,
2.22044604925031E-15));
#152612=CARTESIAN_POINT('',(3.104169711,2.49999999999998,9.24265278));
#152613=CARTESIAN_POINT('Origin',(2.22044604925031E-15,2.49999999999998,
2.22044604925031E-15));
#152614=CARTESIAN_POINT('',(2.391417938,2.49999999999998,8.285800881));
#152615=CARTESIAN_POINT('Origin',(5.676229022,2.49999999999998,6.582857506));
#152616=CARTESIAN_POINT('Origin',(2.22044604925031E-15,2.49999999999998,
2.22044604925031E-15));
#152617=CARTESIAN_POINT('',(1.497503154,2.49999999999998,9.634312861));
#152618=CARTESIAN_POINT('Origin',(2.22044604925031E-15,2.49999999999998,
2.22044604925031E-15));
#152619=CARTESIAN_POINT('',(0.956712422000002,2.49999999999998,8.570768772));
#152620=CARTESIAN_POINT('Origin',(4.482073316,2.49999999999998,7.447456454));
#152621=CARTESIAN_POINT('',(0.505515969000001,2.49999999999998,8.60917125));
#152622=CARTESIAN_POINT('Origin',(2.22044604925031E-15,2.49999999999998,
2.22044604925031E-15));
#152623=CARTESIAN_POINT('',(0.152243842000002,2.49999999999998,9.748811303));
#152624=CARTESIAN_POINT('Origin',(-3.158976522,2.49999999999998,8.09780564));
#152625=CARTESIAN_POINT('',(-0.152243841999998,2.49999999999998,9.748811303));
#152626=CARTESIAN_POINT('Origin',(2.22044604925031E-15,2.49999999999998,
2.22044604925031E-15));
#152627=CARTESIAN_POINT('',(-0.505515968999999,2.49999999999998,8.60917125));
#152628=CARTESIAN_POINT('Origin',(3.158976522,2.49999999999998,8.09780564));
#152629=CARTESIAN_POINT('',(-0.956712421999999,2.49999999999998,8.570768772));
#152630=CARTESIAN_POINT('Origin',(2.22044604925031E-15,2.49999999999998,
2.22044604925031E-15));
#152631=CARTESIAN_POINT('',(-1.497503154,2.49999999999998,9.634312861));
#152632=CARTESIAN_POINT('Origin',(-4.482073316,2.49999999999998,7.447456454));
#152633=CARTESIAN_POINT('',(-1.797611062,2.49999999999998,9.582854192));
#152634=CARTESIAN_POINT('Origin',(2.22044604925031E-15,2.49999999999998,
2.22044604925031E-15));
#152635=CARTESIAN_POINT('',(-1.953201585,2.49999999999998,8.399903545));
#152636=CARTESIAN_POINT('Origin',(1.745001724,2.49999999999998,8.515195702));
#152637=CARTESIAN_POINT('',(-2.391417938,2.49999999999998,8.285800881));
#152638=CARTESIAN_POINT('Origin',(2.22044604925031E-15,2.49999999999998,
2.22044604925031E-15));
#152639=CARTESIAN_POINT('',(-3.104169711,2.49999999999998,9.24265278));
#152640=CARTESIAN_POINT('Origin',(-5.676229022,2.49999999999998,6.582857506));
#152641=CARTESIAN_POINT('',(-3.391264282,2.49999999999998,9.141215815));
#152642=CARTESIAN_POINT('Origin',(2.22044604925031E-15,2.49999999999998,
2.22044604925031E-15));
#152643=CARTESIAN_POINT('',(-3.344697148,2.49999999999998,7.948985909));
#152644=CARTESIAN_POINT('Origin',(0.280826404000001,2.49999999999998,8.687619086));
#152645=CARTESIAN_POINT('',(-3.757326714,2.49999999999998,7.762465586));
#152646=CARTESIAN_POINT('Origin',(2.22044604925031E-15,2.49999999999998,
2.22044604925031E-15));
#152647=CARTESIAN_POINT('',(-4.621534957,2.49999999999998,8.585098406));
#152648=CARTESIAN_POINT('Origin',(-6.707089953,2.49999999999998,5.528881732));
#152649=CARTESIAN_POINT('',(-4.887357004,2.49999999999998,8.436601301));
#152650=CARTESIAN_POINT('Origin',(2.22044604925031E-15,2.49999999999998,
2.22044604925031E-15));
#152651=CARTESIAN_POINT('',(-4.639971864,2.49999999999998,7.269390422));
#152652=CARTESIAN_POINT('Origin',(-1.19142778,2.49999999999998,8.610115487));
#152653=CARTESIAN_POINT('',(-5.015144041,2.49999999999998,7.015818288));
#152654=CARTESIAN_POINT('Origin',(2.22044604925031E-15,2.49999999999998,
2.22044604925031E-15));
#152655=CARTESIAN_POINT('',(-6.005947057,2.49999999999998,7.680566382));
#152656=CARTESIAN_POINT('Origin',(-7.545000119,2.49999999999998,4.315850098));
#152657=CARTESIAN_POINT('',(-6.242849363,2.49999999999998,7.489281129));
#152658=CARTESIAN_POINT('Origin',(2.22044604925031E-15,2.49999999999998,
2.22044604925031E-15));
#152659=CARTESIAN_POINT('',(-5.801763037,2.49999999999998,6.380667807));
#152660=CARTESIAN_POINT('Origin',(-2.629406756,2.49999999999998,8.284914542));
#152661=CARTESIAN_POINT('',(-6.128684805,2.49999999999998,6.067338672));
#152662=CARTESIAN_POINT('Origin',(2.22044604925031E-15,2.49999999999998,
2.22044604925031E-15));
#152663=CARTESIAN_POINT('',(-7.217578995,2.49999999999998,6.555078448));
#152664=CARTESIAN_POINT('Origin',(-8.165854367,2.49999999999998,2.978659314));
#152665=CARTESIAN_POINT('',(-7.418746313,2.49999999999998,6.326507974));
#152666=CARTESIAN_POINT('Origin',(2.22044604925031E-15,2.49999999999998,
2.22044604925031E-15));
#152667=CARTESIAN_POINT('',(-6.796648051,2.49999999999998,5.308384996));
#152668=CARTESIAN_POINT('Origin',(-3.991742488,2.49999999999998,7.721371689));
#152669=CARTESIAN_POINT('',(-7.065914466,2.49999999999998,4.944312768));
#152670=CARTESIAN_POINT('Origin',(2.22044604925031E-15,2.49999999999998,
2.22044604925031E-15));
#152671=CARTESIAN_POINT('',(-8.221574327,2.49999999999998,5.24101284));
#152672=CARTESIAN_POINT('Origin',(-8.551791853,2.49999999999998,1.555777924));
#152673=CARTESIAN_POINT('',(-8.381219438,2.49999999999998,4.981732704));
#152674=CARTESIAN_POINT('Origin',(2.22044604925031E-15,2.49999999999998,
2.22044604925031E-15));
#152675=CARTESIAN_POINT('',(-7.596005875,2.49999999999998,4.083389615));
#152676=CARTESIAN_POINT('Origin',(-5.239243055,2.49999999999998,6.935699032));
#152677=CARTESIAN_POINT('',(-7.799870633,2.49999999999998,3.67904799));
#152678=CARTESIAN_POINT('Origin',(2.22044604925031E-15,2.49999999999998,
2.22044604925031E-15));
#152679=CARTESIAN_POINT('',(-8.989049934,2.49999999999998,3.776172836));
#152680=CARTESIAN_POINT('Origin',(-8.691709858,2.49999999999998,0.088139637000002));
#152681=CARTESIAN_POINT('',(-9.10258013994848,2.49999999999998,3.49364205338694));
#152682=CARTESIAN_POINT('Origin',(2.22044604925031E-15,2.49999999999998,
2.22044604925031E-15));
#152683=CARTESIAN_POINT('',(-8.17684044,2.49999999999998,2.740922548));
#152684=CARTESIAN_POINT('Origin',(-6.33602014,2.49999999999998,5.950498941));
#152685=CARTESIAN_POINT('',(-8.309438723,2.49999999999998,2.307943698));
#152686=CARTESIAN_POINT('Origin',(2.22044604925031E-15,2.49999999999998,
2.22044604925031E-15));
#152687=CARTESIAN_POINT('',(-9.497926941,2.49999999999998,2.202699214));
#152688=CARTESIAN_POINT('Origin',(-8.581583195,2.49999999999998,-1.382034268));
#152689=CARTESIAN_POINT('',(-9.562076184,2.49999999999998,1.905045682));
#152690=CARTESIAN_POINT('Origin',(2.22044604925031E-15,2.49999999999998,
2.22044604925031E-15));
#152691=CARTESIAN_POINT('',(-8.522442193,2.49999999999998,1.31960413));
#152692=CARTESIAN_POINT('Origin',(-7.25052146,2.49999999999998,4.794113829));
#152693=CARTESIAN_POINT('',(-8.579959389,2.49999999999998,0.870444068000003));
#152694=CARTESIAN_POINT('Origin',(2.22044604925031E-15,2.49999999999998,
2.22044604925031E-15));
#152695=CARTESIAN_POINT('',(-9.733565882,2.49999999999998,0.565857946999999));
#152696=CARTESIAN_POINT('Origin',(-8.224580008,2.49999999999998,-2.812449563));
#152697=CARTESIAN_POINT('',(-9.746488706,2.49999999999998,0.261644615999999));
#152698=CARTESIAN_POINT('Origin',(2.22044604925031E-15,2.49999999999998,
2.22044604925031E-15));
#152699=CARTESIAN_POINT('',(-8.622868801,2.49999999999998,-0.139676895));
#152700=CARTESIAN_POINT('Origin',(-7.956438479,2.49999999999998,3.499810792));
#152701=CARTESIAN_POINT('',(-8.603650246,2.49999999999998,-0.592096651999998));
#152702=CARTESIAN_POINT('Origin',(2.22044604925031E-15,2.49999999999998,
2.22044604925031E-15));
#152703=CARTESIAN_POINT('',(-9.689187855,2.49999999999998,-1.087262023));
#152704=CARTESIAN_POINT('Origin',(-7.630970629,2.49999999999998,-4.161955804));
#152705=CARTESIAN_POINT('',(-9.650512493,2.49999999999998,-1.389283491));
#152706=CARTESIAN_POINT('Origin',(2.22044604925031E-15,2.49999999999998,
2.22044604925031E-15));
#152707=CARTESIAN_POINT('',(-8.475231174,2.49999999999998,-1.594939671));
#152708=CARTESIAN_POINT('Origin',(-8.43346325,2.49999999999998,2.10482457));
#152709=CARTESIAN_POINT('',(-8.37982974917112,2.49999999999998,-2.03760383055369));
#152710=CARTESIAN_POINT('Origin',(2.22044604925031E-15,2.49999999999998,
2.22044604925031E-15));
#152711=CARTESIAN_POINT('',(-9.366069535,2.49999999999998,-2.709103444));
#152712=CARTESIAN_POINT('Origin',(-6.817832118,2.49999999999998,-5.391730155));
#152713=CARTESIAN_POINT('',(-9.276908607,2.49999999999998,-3.00024444));
#152714=CARTESIAN_POINT('Origin',(2.22044604925031E-15,2.49999999999998,
2.22044604925031E-15));
#152715=CARTESIAN_POINT('',(-8.083776576,2.49999999999998,-3.004318937));
#152716=CARTESIAN_POINT('Origin',(-8.667872637,2.49999999999998,0.649286377));
#152717=CARTESIAN_POINT('',(-7.914936808,2.49999999999998,-3.424492856));
#152718=CARTESIAN_POINT('Origin',(2.22044604925031E-15,2.49999999999998,
2.22044604925031E-15));
#152719=CARTESIAN_POINT('',(-8.773506446,2.49999999999998,-4.253008892));
#152720=CARTESIAN_POINT('Origin',(-5.808556991,2.49999999999998,-6.466394246));
#152721=CARTESIAN_POINT('',(-8.63642495,2.49999999999998,-4.524893819));
#152722=CARTESIAN_POINT('Origin',(2.22044604925031E-15,2.49999999999998,
2.22044604925031E-15));
#152723=CARTESIAN_POINT('',(-7.459766444,2.49999999999998,-4.327269417));
#152724=CARTESIAN_POINT('Origin',(-8.65292311,2.49999999999998,-0.824930601999998));
#152725=CARTESIAN_POINT('',(-7.222345546,2.49999999999998,-4.712865457));
#152726=CARTESIAN_POINT('Origin',(2.22044604925031E-15,2.49999999999998,
2.22044604925031E-15));
#152727=CARTESIAN_POINT('',(-7.928545552,2.49999999999998,-5.674563017));
#152728=CARTESIAN_POINT('Origin',(-4.632180254,2.49999999999998,-7.355031947));
#152729=CARTESIAN_POINT('',(-7.747487072,2.49999999999998,-5.919370243));
#152730=CARTESIAN_POINT('Origin',(2.22044604925031E-15,2.49999999999998,
2.22044604925031E-15));
#152731=CARTESIAN_POINT('',(-6.621152413,2.49999999999998,-5.525732234));
#152732=CARTESIAN_POINT('Origin',(-8.38904474,2.49999999999998,-2.275415831));
#152733=CARTESIAN_POINT('',(-6.321980552,2.49999999999998,-5.8656575));
#152734=CARTESIAN_POINT('Origin',(2.22044604925031E-15,2.49999999999998,
2.22044604925031E-15));
#152735=CARTESIAN_POINT('',(-6.855494836,2.49999999999998,-6.932870296));
#152736=CARTESIAN_POINT('Origin',(-3.322544125,2.49999999999998,-8.032078771));
#152737=CARTESIAN_POINT('',(-6.635668096,2.49999999999998,-7.143557161));
#152738=CARTESIAN_POINT('Origin',(2.22044604925031E-15,2.49999999999998,
2.22044604925031E-15));
#152739=CARTESIAN_POINT('',(-5.592059883,2.49999999999998,-6.565229795));
#152740=CARTESIAN_POINT('Origin',(-7.883828827,2.49999999999998,-3.660441488));
#152741=CARTESIAN_POINT('',(-5.239743688,2.49999999999998,-6.849705256));
#152742=CARTESIAN_POINT('Origin',(2.22044604925031E-15,2.49999999999998,
2.22044604925031E-15));
#152743=CARTESIAN_POINT('',(-5.585224017,2.49999999999998,-7.991731519));
#152744=CARTESIAN_POINT('Origin',(-1.917324452,2.49999999999998,-8.478057313));
#152745=CARTESIAN_POINT('',(-5.3329530316541,2.49999999999998,-8.16223694556031));
#152746=CARTESIAN_POINT('Origin',(2.22044604925031E-15,2.49999999999998,
2.22044604925031E-15));
#152747=CARTESIAN_POINT('',(-4.402093971,2.49999999999998,-7.415857649));
#152748=CARTESIAN_POINT('Origin',(-7.151809512,2.49999999999998,-4.940162908));
#152749=CARTESIAN_POINT('',(-4.006768937,2.49999999999998,-7.636699463));
#152750=CARTESIAN_POINT('Origin',(2.22044604925031E-15,2.49999999999998,
2.22044604925031E-15));
#152751=CARTESIAN_POINT('',(-4.154276471,2.49999999999998,-8.820685177));
#152752=CARTESIAN_POINT('Origin',(-0.456946843999999,2.49999999999998,-8.680137582));
#152753=CARTESIAN_POINT('',(-3.876818617,2.49999999999998,-8.946104035));
#152754=CARTESIAN_POINT('Origin',(2.22044604925031E-15,2.49999999999998,
2.22044604925031E-15));
#152755=CARTESIAN_POINT('',(-3.085487831,2.49999999999998,-8.05314478));
#152756=CARTESIAN_POINT('Origin',(-6.214045658,2.49999999999998,-6.077764837));
#152757=CARTESIAN_POINT('',(-2.65852674,2.49999999999998,-8.20399973));
#152758=CARTESIAN_POINT('Origin',(2.22044604925031E-15,2.49999999999998,
2.22044604925031E-15));
#152759=CARTESIAN_POINT('',(-2.60381795543899,2.49999999999998,-9.3958837827716));
#152760=CARTESIAN_POINT('Origin',(1.016576292,2.49999999999998,-8.632506096));
#152761=CARTESIAN_POINT('',(-2.30915519,2.49999999999998,-9.472607999));
#152762=CARTESIAN_POINT('Origin',(2.22044604925031E-15,2.49999999999998,
2.22044604925031E-15));
#152763=CARTESIAN_POINT('',(-1.680117823,2.49999999999998,-8.458757598));
#152764=CARTESIAN_POINT('Origin',(-5.097515025,2.49999999999998,-7.040520536));
#152765=CARTESIAN_POINT('',(-1.233803569,2.49999999999998,-8.535285862));
#152766=CARTESIAN_POINT('Origin',(2.22044604925031E-15,2.49999999999998,
2.22044604925031E-15));
#152767=CARTESIAN_POINT('',(-0.978452337999998,2.49999999999998,-9.700779918));
#152768=CARTESIAN_POINT('Origin',(2.460854379,2.49999999999998,-8.336533127));
#152769=CARTESIAN_POINT('',(-0.675061571999999,2.49999999999998,-9.726602278));
#152770=CARTESIAN_POINT('Origin',(2.22044604925031E-15,2.49999999999998,
2.22044604925031E-15));
#152771=CARTESIAN_POINT('',(-0.226413884999999,2.49999999999998,-8.621027361));
#152772=CARTESIAN_POINT('Origin',(-3.834338166,2.49999999999998,-7.800733278));
#152773=CARTESIAN_POINT('',(0.226413885000002,2.49999999999998,-8.621027361));
#152774=CARTESIAN_POINT('Origin',(2.22044604925031E-15,2.49999999999998,
2.22044604925031E-15));
#152775=CARTESIAN_POINT('',(0.675061572000001,2.49999999999998,-9.726602278));
#152776=CARTESIAN_POINT('Origin',(3.834338166,2.49999999999998,-7.800733278));
#152777=CARTESIAN_POINT('',(0.978452338000002,2.49999999999998,-9.700779918));
#152778=CARTESIAN_POINT('Origin',(2.22044604925031E-15,2.49999999999998,
2.22044604925031E-15));
#152779=CARTESIAN_POINT('',(1.233803568,2.49999999999998,-8.535285863));
#152780=CARTESIAN_POINT('Origin',(-2.460854379,2.49999999999998,-8.336533127));
#152781=CARTESIAN_POINT('',(1.680117823,2.49999999999998,-8.458757598));
#152782=CARTESIAN_POINT('Origin',(2.22044604925031E-15,2.49999999999998,
2.22044604925031E-15));
#152783=CARTESIAN_POINT('',(2.30915519,2.49999999999998,-9.472607999));
#152784=CARTESIAN_POINT('Origin',(5.097515025,2.49999999999998,-7.040520536));
#152785=CARTESIAN_POINT('Origin',(2.22044604925031E-15,2.49999999999998,
2.22044604925031E-15));
#152786=CARTESIAN_POINT('',(3.08548783,2.49999999999998,-8.05314478));
#152787=CARTESIAN_POINT('Origin',(2.22044604925031E-15,2.49999999999998,
2.22044604925031E-15));
#152788=CARTESIAN_POINT('',(3.876818617,2.49999999999998,-8.946104035));
#152789=CARTESIAN_POINT('Origin',(6.214045658,2.49999999999998,-6.077764837));
#152790=CARTESIAN_POINT('Origin',(2.22044604925031E-15,2.49999999999998,
2.22044604925031E-15));
#152791=CARTESIAN_POINT('',(4.402093972,2.49999999999998,-7.415857648));
#152792=CARTESIAN_POINT('Origin',(2.22044604925031E-15,2.49999999999998,
2.22044604925031E-15));
#152793=CARTESIAN_POINT('',(5.33295303165411,2.49999999999998,-8.16223694556031));
#152794=CARTESIAN_POINT('Origin',(7.151809512,2.49999999999998,-4.940162908));
#152795=CARTESIAN_POINT('',(5.585224017,2.49999999999998,-7.991731519));
#152796=CARTESIAN_POINT('Origin',(2.22044604925031E-15,2.49999999999998,
2.22044604925031E-15));
#152797=CARTESIAN_POINT('',(5.239743687,2.49999999999998,-6.849705256));
#152798=CARTESIAN_POINT('Origin',(1.917324452,2.49999999999998,-8.478057313));
#152799=CARTESIAN_POINT('',(5.592059883,2.49999999999998,-6.565229795));
#152800=CARTESIAN_POINT('Origin',(2.22044604925031E-15,2.49999999999998,
2.22044604925031E-15));
#152801=CARTESIAN_POINT('',(6.635668096,2.49999999999998,-7.143557161));
#152802=CARTESIAN_POINT('Origin',(7.883828827,2.49999999999998,-3.660441488));
#152803=CARTESIAN_POINT('',(6.855494836,2.49999999999998,-6.932870296));
#152804=CARTESIAN_POINT('Origin',(2.22044604925031E-15,2.49999999999998,
2.22044604925031E-15));
#152805=CARTESIAN_POINT('',(6.321980552,2.49999999999998,-5.8656575));
#152806=CARTESIAN_POINT('Origin',(3.322544125,2.49999999999998,-8.032078771));
#152807=CARTESIAN_POINT('',(6.621152413,2.49999999999998,-5.525732234));
#152808=CARTESIAN_POINT('Origin',(2.22044604925031E-15,2.49999999999998,
2.22044604925031E-15));
#152809=CARTESIAN_POINT('',(7.747487072,2.49999999999998,-5.919370243));
#152810=CARTESIAN_POINT('Origin',(8.38904474,2.49999999999998,-2.275415831));
#152811=CARTESIAN_POINT('',(7.928545552,2.49999999999998,-5.674563017));
#152812=CARTESIAN_POINT('Origin',(2.22044604925031E-15,2.49999999999998,
2.22044604925031E-15));
#152813=CARTESIAN_POINT('',(7.222345546,2.49999999999998,-4.712865457));
#152814=CARTESIAN_POINT('Origin',(4.632180254,2.49999999999998,-7.355031947));
#152815=CARTESIAN_POINT('',(7.459766444,2.49999999999998,-4.327269416));
#152816=CARTESIAN_POINT('Origin',(2.22044604925031E-15,2.49999999999998,
2.22044604925031E-15));
#152817=CARTESIAN_POINT('',(8.63642495,2.49999999999998,-4.524893819));
#152818=CARTESIAN_POINT('Origin',(8.65292311,2.49999999999998,-0.824930601999998));
#152819=CARTESIAN_POINT('',(8.773506446,2.49999999999998,-4.253008892));
#152820=CARTESIAN_POINT('Origin',(2.22044604925031E-15,2.49999999999998,
2.22044604925031E-15));
#152821=CARTESIAN_POINT('',(7.914936808,2.49999999999998,-3.424492856));
#152822=CARTESIAN_POINT('Origin',(5.808556991,2.49999999999998,-6.466394246));
#152823=CARTESIAN_POINT('',(8.083776576,2.49999999999998,-3.004318937));
#152824=CARTESIAN_POINT('Origin',(2.22044604925031E-15,2.49999999999998,
2.22044604925031E-15));
#152825=CARTESIAN_POINT('',(9.276908607,2.49999999999998,-3.00024444));
#152826=CARTESIAN_POINT('Origin',(8.667872637,2.49999999999998,0.649286377));
#152827=CARTESIAN_POINT('',(9.366069535,2.49999999999998,-2.709103444));
#152828=CARTESIAN_POINT('Origin',(2.22044604925031E-15,2.49999999999998,
2.22044604925031E-15));
#152829=CARTESIAN_POINT('',(8.37982974945342,2.49999999999998,-2.03760383017956));
#152830=CARTESIAN_POINT('Origin',(6.817832118,2.49999999999998,-5.391730155));
#152831=CARTESIAN_POINT('',(8.475231174,2.49999999999998,-1.594939671));
#152832=CARTESIAN_POINT('Origin',(2.22044604925031E-15,2.49999999999998,
2.22044604925031E-15));
#152833=CARTESIAN_POINT('',(9.650512493,2.49999999999998,-1.389283491));
#152834=CARTESIAN_POINT('Origin',(8.43346325,2.49999999999998,2.10482457));
#152835=CARTESIAN_POINT('Origin',(2.22044604925031E-15,2.49999999999998,
2.22044604925031E-15));
#152836=CARTESIAN_POINT('',(-4.394532211,2.49999999999998,-1.93082538));
#152837=CARTESIAN_POINT('',(4.394532211,2.49999999999998,-1.93082538));
#152838=CARTESIAN_POINT('Origin',(2.22044604925031E-15,2.49999999999998,
2.22044604925031E-15));
#152839=CARTESIAN_POINT('',(5.143848737,2.49999999999998,-1.606493127));
#152840=CARTESIAN_POINT('Origin',(4.943848737,2.49999999999998,-2.172178552));
#152841=CARTESIAN_POINT('',(5.143848737,2.49999999999998,-1.606493127));
#152842=CARTESIAN_POINT('',(-6.819607843,2.49999999999998,-2.872794609));
#152843=CARTESIAN_POINT('Origin',(2.22044604925031E-15,2.49999999999998,
2.22044604925031E-15));
#152844=CARTESIAN_POINT('',(-6.466666667,2.49999999999998,-2.074179891));
#152845=CARTESIAN_POINT('Origin',(-6.266666667,2.49999999999998,-2.639865316));
#152846=CARTESIAN_POINT('',(-5.143848737,2.49999999999998,-1.606493127));
#152847=CARTESIAN_POINT('',(-6.466666667,2.49999999999998,-2.074179891));
#152848=CARTESIAN_POINT('Origin',(-4.943848737,2.49999999999998,-2.172178552));
#152849=CARTESIAN_POINT('',(-5.143848737,2.49999999999998,1.606493127));
#152850=CARTESIAN_POINT('',(-6.466666667,2.49999999999998,2.074179891));
#152851=CARTESIAN_POINT('',(-5.143848737,2.49999999999998,1.606493127));
#152852=CARTESIAN_POINT('',(-6.819607843,2.49999999999998,2.872794609));
#152853=CARTESIAN_POINT('Origin',(-6.266666667,2.49999999999998,2.639865316));
#152854=CARTESIAN_POINT('Origin',(2.22044604925031E-15,2.49999999999998,
2.22044604925031E-15));
#152855=CARTESIAN_POINT('',(5.143848737,2.49999999999998,1.606493127));
#152856=CARTESIAN_POINT('',(6.466666667,2.49999999999998,2.074179891));
#152857=CARTESIAN_POINT('',(4.394532211,2.49999999999998,1.93082538));
#152858=CARTESIAN_POINT('Origin',(4.943848737,2.49999999999998,2.172178552));
#152859=CARTESIAN_POINT('',(-4.394532211,2.49999999999998,1.93082538));
#152860=CARTESIAN_POINT('Origin',(2.22044604925031E-15,2.49999999999998,
2.22044604925031E-15));
#152861=CARTESIAN_POINT('Origin',(-4.943848737,2.49999999999998,2.172178552));
#152862=CARTESIAN_POINT('Origin',(2.22044604925031E-15,17.5,2.22044604925031E-15));
#152863=CARTESIAN_POINT('',(9.689187855,7.49999999999998,-1.087262023));
#152864=CARTESIAN_POINT('',(9.689187855,2.49999999999998,-1.087262023));
#152865=CARTESIAN_POINT('',(9.650512493,7.49999999999998,-1.389283491));
#152866=CARTESIAN_POINT('',(9.650512493,7.49999999999998,-1.389283491));
#152867=CARTESIAN_POINT('Origin',(2.22044604925031E-15,7.49999999999998,
2.22044604925031E-15));
#152868=CARTESIAN_POINT('Origin',(2.22044604925031E-15,17.5,2.22044604925031E-15));
#152869=CARTESIAN_POINT('',(9.746488706,7.49999999999998,0.261644615999999));
#152870=CARTESIAN_POINT('',(9.746488706,7.49999999999998,0.261644615999999));
#152871=CARTESIAN_POINT('',(9.733565882,7.49999999999998,0.565857946999999));
#152872=CARTESIAN_POINT('Origin',(2.22044604925031E-15,7.49999999999998,
2.22044604925031E-15));
#152873=CARTESIAN_POINT('',(9.733565882,2.49999999999998,0.565857946999999));
#152874=CARTESIAN_POINT('Origin',(2.22044604925031E-15,17.5,2.22044604925031E-15));
#152875=CARTESIAN_POINT('',(9.366069535,7.49999999999998,-2.709103444));
#152876=CARTESIAN_POINT('',(9.366069535,2.49999999999998,-2.709103444));
#152877=CARTESIAN_POINT('',(9.276908607,7.49999999999998,-3.00024444));
#152878=CARTESIAN_POINT('',(9.276908607,7.49999999999998,-3.00024444));
#152879=CARTESIAN_POINT('Origin',(2.22044604925031E-15,7.49999999999998,
2.22044604925031E-15));
#152880=CARTESIAN_POINT('Origin',(2.22044604925031E-15,17.5,2.22044604925031E-15));
#152881=CARTESIAN_POINT('',(8.773506446,7.49999999999998,-4.253008892));
#152882=CARTESIAN_POINT('',(8.773506446,2.49999999999998,-4.253008892));
#152883=CARTESIAN_POINT('',(8.63642495,7.49999999999998,-4.524893819));
#152884=CARTESIAN_POINT('',(8.63642495,7.49999999999998,-4.524893819));
#152885=CARTESIAN_POINT('Origin',(2.22044604925031E-15,7.49999999999998,
2.22044604925031E-15));
#152886=CARTESIAN_POINT('Origin',(2.22044604925031E-15,17.5,2.22044604925031E-15));
#152887=CARTESIAN_POINT('',(7.928545552,7.49999999999998,-5.674563017));
#152888=CARTESIAN_POINT('',(7.928545552,2.49999999999998,-5.674563017));
#152889=CARTESIAN_POINT('',(7.747487072,7.49999999999998,-5.919370243));
#152890=CARTESIAN_POINT('',(7.747487072,7.49999999999998,-5.919370243));
#152891=CARTESIAN_POINT('Origin',(2.22044604925031E-15,7.49999999999998,
2.22044604925031E-15));
#152892=CARTESIAN_POINT('Origin',(2.22044604925031E-15,17.5,2.22044604925031E-15));
#152893=CARTESIAN_POINT('',(2.30915519,7.49999999999998,-9.472607999));
#152894=CARTESIAN_POINT('',(2.30915519,7.49999999999998,-9.472607999));
#152895=CARTESIAN_POINT('Origin',(2.22044604925031E-15,7.49999999999998,
2.22044604925031E-15));
#152896=CARTESIAN_POINT('Origin',(2.22044604925031E-15,17.5,2.22044604925031E-15));
#152897=CARTESIAN_POINT('',(3.876818617,7.49999999999998,-8.946104035));
#152898=CARTESIAN_POINT('',(3.876818617,7.49999999999998,-8.946104035));
#152899=CARTESIAN_POINT('Origin',(2.22044604925031E-15,7.49999999999998,
2.22044604925031E-15));
#152900=CARTESIAN_POINT('Origin',(2.22044604925031E-15,17.5,2.22044604925031E-15));
#152901=CARTESIAN_POINT('',(5.33295303165411,7.49999999999998,-8.16223694556031));
#152902=CARTESIAN_POINT('',(5.332953031,7.49999999999998,-8.162236945));
#152903=CARTESIAN_POINT('',(5.585224017,7.49999999999998,-7.991731519));
#152904=CARTESIAN_POINT('Origin',(2.22044604925031E-15,7.49999999999998,
2.22044604925031E-15));
#152905=CARTESIAN_POINT('',(5.585224017,2.49999999999998,-7.991731519));
#152906=CARTESIAN_POINT('Origin',(2.22044604925031E-15,17.5,2.22044604925031E-15));
#152907=CARTESIAN_POINT('',(6.855494836,7.49999999999998,-6.932870296));
#152908=CARTESIAN_POINT('',(6.855494836,2.49999999999998,-6.932870296));
#152909=CARTESIAN_POINT('',(6.635668096,7.49999999999998,-7.143557161));
#152910=CARTESIAN_POINT('',(6.635668096,7.49999999999998,-7.143557161));
#152911=CARTESIAN_POINT('Origin',(2.22044604925031E-15,7.49999999999998,
2.22044604925031E-15));
#152912=CARTESIAN_POINT('Origin',(2.22044604925031E-15,17.5,2.22044604925031E-15));
#152913=CARTESIAN_POINT('',(6.005947057,7.49999999999998,7.680566382));
#152914=CARTESIAN_POINT('',(6.005947057,2.49999999999998,7.680566382));
#152915=CARTESIAN_POINT('',(6.242849363,7.49999999999998,7.489281129));
#152916=CARTESIAN_POINT('',(6.242849363,7.49999999999998,7.489281129));
#152917=CARTESIAN_POINT('Origin',(2.22044604925031E-15,7.49999999999998,
2.22044604925031E-15));
#152918=CARTESIAN_POINT('Origin',(2.22044604925031E-15,17.5,2.22044604925031E-15));
#152919=CARTESIAN_POINT('',(4.887357004,7.49999999999998,8.436601301));
#152920=CARTESIAN_POINT('',(4.887357004,7.49999999999998,8.436601301));
#152921=CARTESIAN_POINT('',(4.621534957,7.49999999999998,8.585098406));
#152922=CARTESIAN_POINT('Origin',(2.22044604925031E-15,7.49999999999998,
2.22044604925031E-15));
#152923=CARTESIAN_POINT('',(4.621534957,2.49999999999998,8.585098406));
#152924=CARTESIAN_POINT('Origin',(2.22044604925031E-15,17.5,2.22044604925031E-15));
#152925=CARTESIAN_POINT('',(7.217578995,7.49999999999998,6.555078448));
#152926=CARTESIAN_POINT('',(7.217578995,2.49999999999998,6.555078448));
#152927=CARTESIAN_POINT('',(7.418746313,7.49999999999998,6.326507974));
#152928=CARTESIAN_POINT('',(7.418746313,7.49999999999998,6.326507974));
#152929=CARTESIAN_POINT('Origin',(2.22044604925031E-15,7.49999999999998,
2.22044604925031E-15));
#152930=CARTESIAN_POINT('Origin',(2.22044604925031E-15,17.5,2.22044604925031E-15));
#152931=CARTESIAN_POINT('',(3.104169711,7.49999999999998,9.24265278));
#152932=CARTESIAN_POINT('Origin',(2.22044604925031E-15,7.49999999999998,
2.22044604925031E-15));
#152933=CARTESIAN_POINT('',(3.104169711,2.49999999999998,9.24265278));
#152934=CARTESIAN_POINT('Origin',(2.22044604925031E-15,17.5,2.22044604925031E-15));
#152935=CARTESIAN_POINT('',(1.497503154,7.49999999999998,9.634312861));
#152936=CARTESIAN_POINT('Origin',(2.22044604925031E-15,7.49999999999998,
2.22044604925031E-15));
#152937=CARTESIAN_POINT('',(1.497503154,2.49999999999998,9.634312861));
#152938=CARTESIAN_POINT('Origin',(2.22044604925031E-15,17.5,2.22044604925031E-15));
#152939=CARTESIAN_POINT('',(0.152243842000002,7.49999999999998,9.748811303));
#152940=CARTESIAN_POINT('',(0.152243842000002,7.49999999999998,9.748811303));
#152941=CARTESIAN_POINT('',(-0.152243841999998,7.49999999999998,9.748811303));
#152942=CARTESIAN_POINT('Origin',(2.22044604925031E-15,7.49999999999998,
2.22044604925031E-15));
#152943=CARTESIAN_POINT('',(-0.152243841999998,2.49999999999998,9.748811303));
#152944=CARTESIAN_POINT('Origin',(2.22044604925031E-15,17.5,2.22044604925031E-15));
#152945=CARTESIAN_POINT('',(8.989049934,7.49999999999998,3.776172836));
#152946=CARTESIAN_POINT('',(8.989049934,2.49999999999998,3.776172836));
#152947=CARTESIAN_POINT('',(9.10258013994849,7.49999999999998,3.49364205338695));
#152948=CARTESIAN_POINT('',(9.10258014,7.49999999999998,3.493642054));
#152949=CARTESIAN_POINT('Origin',(2.22044604925031E-15,7.49999999999998,
2.22044604925031E-15));
#152950=CARTESIAN_POINT('Origin',(2.22044604925031E-15,17.5,2.22044604925031E-15));
#152951=CARTESIAN_POINT('',(8.381219438,7.49999999999998,4.981732704));
#152952=CARTESIAN_POINT('',(8.381219438,7.49999999999998,4.981732704));
#152953=CARTESIAN_POINT('',(8.221574327,7.49999999999998,5.24101284));
#152954=CARTESIAN_POINT('Origin',(2.22044604925031E-15,7.49999999999998,
2.22044604925031E-15));
#152955=CARTESIAN_POINT('',(8.221574327,2.49999999999998,5.24101284));
#152956=CARTESIAN_POINT('Origin',(2.22044604925031E-15,17.5,2.22044604925031E-15));
#152957=CARTESIAN_POINT('',(9.497926941,7.49999999999998,2.202699214));
#152958=CARTESIAN_POINT('',(9.497926941,2.49999999999998,2.202699214));
#152959=CARTESIAN_POINT('',(9.562076184,7.49999999999998,1.905045682));
#152960=CARTESIAN_POINT('',(9.562076184,7.49999999999998,1.905045682));
#152961=CARTESIAN_POINT('Origin',(2.22044604925031E-15,7.49999999999998,
2.22044604925031E-15));
#152962=CARTESIAN_POINT('Origin',(2.22044604925031E-15,17.5,2.22044604925031E-15));
#152963=CARTESIAN_POINT('',(-7.418746313,7.49999999999998,6.326507974));
#152964=CARTESIAN_POINT('',(-7.418746313,2.49999999999998,6.326507974));
#152965=CARTESIAN_POINT('',(-7.217578995,7.49999999999998,6.555078448));
#152966=CARTESIAN_POINT('',(-7.217578995,7.49999999999998,6.555078448));
#152967=CARTESIAN_POINT('Origin',(2.22044604925031E-15,7.49999999999998,
2.22044604925031E-15));
#152968=CARTESIAN_POINT('Origin',(2.22044604925031E-15,17.5,2.22044604925031E-15));
#152969=CARTESIAN_POINT('',(-8.221574327,7.49999999999998,5.24101284));
#152970=CARTESIAN_POINT('',(-8.221574327,7.49999999999998,5.24101284));
#152971=CARTESIAN_POINT('',(-8.381219438,7.49999999999998,4.981732704));
#152972=CARTESIAN_POINT('Origin',(2.22044604925031E-15,7.49999999999998,
2.22044604925031E-15));
#152973=CARTESIAN_POINT('',(-8.381219438,2.49999999999998,4.981732704));
#152974=CARTESIAN_POINT('Origin',(2.22044604925031E-15,17.5,2.22044604925031E-15));
#152975=CARTESIAN_POINT('',(-6.242849363,7.49999999999998,7.489281129));
#152976=CARTESIAN_POINT('',(-6.242849363,2.49999999999998,7.489281129));
#152977=CARTESIAN_POINT('',(-6.005947057,7.49999999999998,7.680566382));
#152978=CARTESIAN_POINT('',(-6.005947057,7.49999999999998,7.680566382));
#152979=CARTESIAN_POINT('Origin',(2.22044604925031E-15,7.49999999999998,
2.22044604925031E-15));
#152980=CARTESIAN_POINT('Origin',(2.22044604925031E-15,17.5,2.22044604925031E-15));
#152981=CARTESIAN_POINT('',(-8.989049934,7.49999999999998,3.776172836));
#152982=CARTESIAN_POINT('',(-8.989049934,7.49999999999998,3.776172836));
#152983=CARTESIAN_POINT('',(-9.10258013994848,7.49999999999998,3.49364205338695));
#152984=CARTESIAN_POINT('Origin',(2.22044604925031E-15,7.49999999999998,
2.22044604925031E-15));
#152985=CARTESIAN_POINT('',(-9.10258014,2.49999999999998,3.493642054));
#152986=CARTESIAN_POINT('Origin',(2.22044604925031E-15,17.5,2.22044604925031E-15));
#152987=CARTESIAN_POINT('',(-9.497926941,7.49999999999998,2.202699214));
#152988=CARTESIAN_POINT('',(-9.497926941,7.49999999999998,2.202699214));
#152989=CARTESIAN_POINT('',(-9.562076184,7.49999999999998,1.905045682));
#152990=CARTESIAN_POINT('Origin',(2.22044604925031E-15,7.49999999999998,
2.22044604925031E-15));
#152991=CARTESIAN_POINT('',(-9.562076184,2.49999999999998,1.905045682));
#152992=CARTESIAN_POINT('Origin',(2.22044604925031E-15,17.5,2.22044604925031E-15));
#152993=CARTESIAN_POINT('',(-9.733565882,7.49999999999998,0.565857946999999));
#152994=CARTESIAN_POINT('',(-9.733565882,7.49999999999998,0.565857946999999));
#152995=CARTESIAN_POINT('',(-9.746488706,7.49999999999998,0.261644615999999));
#152996=CARTESIAN_POINT('Origin',(2.22044604925031E-15,7.49999999999998,
2.22044604925031E-15));
#152997=CARTESIAN_POINT('',(-9.746488706,2.49999999999998,0.261644615999999));
#152998=CARTESIAN_POINT('Origin',(2.22044604925031E-15,17.5,2.22044604925031E-15));
#152999=CARTESIAN_POINT('',(-3.391264282,7.49999999999998,9.141215815));
#153000=CARTESIAN_POINT('',(-3.391264282,2.49999999999998,9.141215815));
#153001=CARTESIAN_POINT('',(-3.104169711,7.49999999999998,9.24265278));
#153002=CARTESIAN_POINT('',(-3.104169711,7.49999999999998,9.24265278));
#153003=CARTESIAN_POINT('Origin',(2.22044604925031E-15,7.49999999999998,
2.22044604925031E-15));
#153004=CARTESIAN_POINT('Origin',(2.22044604925031E-15,17.5,2.22044604925031E-15));
#153005=CARTESIAN_POINT('',(-4.621534957,7.49999999999998,8.585098406));
#153006=CARTESIAN_POINT('',(-4.621534957,7.49999999999998,8.585098406));
#153007=CARTESIAN_POINT('',(-4.887357004,7.49999999999998,8.436601301));
#153008=CARTESIAN_POINT('Origin',(2.22044604925031E-15,7.49999999999998,
2.22044604925031E-15));
#153009=CARTESIAN_POINT('',(-4.887357004,2.49999999999998,8.436601301));
#153010=CARTESIAN_POINT('Origin',(2.22044604925031E-15,17.5,2.22044604925031E-15));
#153011=CARTESIAN_POINT('',(-1.797611062,7.49999999999998,9.582854192));
#153012=CARTESIAN_POINT('',(-1.797611062,2.49999999999998,9.582854192));
#153013=CARTESIAN_POINT('',(-1.497503154,7.49999999999998,9.634312861));
#153014=CARTESIAN_POINT('',(-1.497503154,7.49999999999998,9.634312861));
#153015=CARTESIAN_POINT('Origin',(2.22044604925031E-15,7.49999999999998,
2.22044604925031E-15));
#153016=CARTESIAN_POINT('Origin',(2.22044604925031E-15,17.5,2.22044604925031E-15));
#153017=CARTESIAN_POINT('',(-6.635668096,7.49999999999998,-7.143557161));
#153018=CARTESIAN_POINT('',(-6.635668096,2.49999999999998,-7.143557161));
#153019=CARTESIAN_POINT('',(-6.855494836,7.49999999999998,-6.932870296));
#153020=CARTESIAN_POINT('',(-6.855494836,7.49999999999998,-6.932870296));
#153021=CARTESIAN_POINT('Origin',(2.22044604925031E-15,7.49999999999998,
2.22044604925031E-15));
#153022=CARTESIAN_POINT('Origin',(2.22044604925031E-15,17.5,2.22044604925031E-15));
#153023=CARTESIAN_POINT('',(-5.585224017,7.49999999999998,-7.991731519));
#153024=CARTESIAN_POINT('',(-5.585224017,7.49999999999998,-7.991731519));
#153025=CARTESIAN_POINT('',(-5.33295303165411,7.49999999999998,-8.16223694556031));
#153026=CARTESIAN_POINT('Origin',(2.22044604925031E-15,7.49999999999998,
2.22044604925031E-15));
#153027=CARTESIAN_POINT('',(-5.332953031,2.49999999999998,-8.162236945));
#153028=CARTESIAN_POINT('Origin',(2.22044604925031E-15,17.5,2.22044604925031E-15));
#153029=CARTESIAN_POINT('',(-7.747487072,7.49999999999998,-5.919370243));
#153030=CARTESIAN_POINT('',(-7.747487072,2.49999999999998,-5.919370243));
#153031=CARTESIAN_POINT('',(-7.928545552,7.49999999999998,-5.674563017));
#153032=CARTESIAN_POINT('',(-7.928545552,7.49999999999998,-5.674563017));
#153033=CARTESIAN_POINT('Origin',(2.22044604925031E-15,7.49999999999998,
2.22044604925031E-15));
#153034=CARTESIAN_POINT('Origin',(2.22044604925031E-15,17.5,2.22044604925031E-15));
#153035=CARTESIAN_POINT('',(-4.154276471,7.49999999999998,-8.820685177));
#153036=CARTESIAN_POINT('',(-4.154276471,7.49999999999998,-8.820685177));
#153037=CARTESIAN_POINT('',(-3.876818617,7.49999999999998,-8.946104035));
#153038=CARTESIAN_POINT('Origin',(2.22044604925031E-15,7.49999999999998,
2.22044604925031E-15));
#153039=CARTESIAN_POINT('',(-3.876818617,2.49999999999998,-8.946104035));
#153040=CARTESIAN_POINT('Origin',(2.22044604925031E-15,17.5,2.22044604925031E-15));
#153041=CARTESIAN_POINT('',(-2.60381795543899,7.49999999999998,-9.3958837827716));
#153042=CARTESIAN_POINT('',(-2.603817955,7.49999999999998,-9.395883783));
#153043=CARTESIAN_POINT('',(-2.30915519,7.49999999999998,-9.472607999));
#153044=CARTESIAN_POINT('Origin',(2.22044604925031E-15,7.49999999999998,
2.22044604925031E-15));
#153045=CARTESIAN_POINT('',(-2.30915519,2.49999999999998,-9.472607999));
#153046=CARTESIAN_POINT('Origin',(2.22044604925031E-15,17.5,2.22044604925031E-15));
#153047=CARTESIAN_POINT('',(-0.978452337999998,7.49999999999998,-9.700779918));
#153048=CARTESIAN_POINT('',(-0.978452337999998,7.49999999999998,-9.700779918));
#153049=CARTESIAN_POINT('',(-0.675061571999999,7.49999999999998,-9.726602278));
#153050=CARTESIAN_POINT('Origin',(2.22044604925031E-15,7.49999999999998,
2.22044604925031E-15));
#153051=CARTESIAN_POINT('',(-0.675061571999999,2.49999999999998,-9.726602278));
#153052=CARTESIAN_POINT('Origin',(2.22044604925031E-15,17.5,2.22044604925031E-15));
#153053=CARTESIAN_POINT('',(-8.63642495,7.49999999999998,-4.524893819));
#153054=CARTESIAN_POINT('',(-8.63642495,2.49999999999998,-4.524893819));
#153055=CARTESIAN_POINT('',(-8.773506446,7.49999999999998,-4.253008892));
#153056=CARTESIAN_POINT('',(-8.773506446,7.49999999999998,-4.253008892));
#153057=CARTESIAN_POINT('Origin',(2.22044604925031E-15,7.49999999999998,
2.22044604925031E-15));
#153058=CARTESIAN_POINT('Origin',(2.22044604925031E-15,17.5,2.22044604925031E-15));
#153059=CARTESIAN_POINT('',(-9.276908607,7.49999999999998,-3.00024444));
#153060=CARTESIAN_POINT('',(-9.276908607,2.49999999999998,-3.00024444));
#153061=CARTESIAN_POINT('',(-9.366069535,7.49999999999998,-2.709103444));
#153062=CARTESIAN_POINT('',(-9.366069535,7.49999999999998,-2.709103444));
#153063=CARTESIAN_POINT('Origin',(2.22044604925031E-15,7.49999999999998,
2.22044604925031E-15));
#153064=CARTESIAN_POINT('Origin',(2.22044604925031E-15,17.5,2.22044604925031E-15));
#153065=CARTESIAN_POINT('',(-9.650512493,7.49999999999998,-1.389283491));
#153066=CARTESIAN_POINT('',(-9.650512493,2.49999999999998,-1.389283491));
#153067=CARTESIAN_POINT('',(-9.689187855,7.49999999999998,-1.087262023));
#153068=CARTESIAN_POINT('',(-9.689187855,7.49999999999998,-1.087262023));
#153069=CARTESIAN_POINT('Origin',(2.22044604925031E-15,7.49999999999998,
2.22044604925031E-15));
#153070=CARTESIAN_POINT('Origin',(2.22044604925031E-15,7.49999999999998,
2.22044604925031E-15));
#153071=CARTESIAN_POINT('',(8.603650246,7.49999999999998,-0.592096652999998));
#153072=CARTESIAN_POINT('Origin',(7.630970629,7.49999999999998,-4.161955804));
#153073=CARTESIAN_POINT('',(8.475231174,7.49999999999998,-1.594939671));
#153074=CARTESIAN_POINT('Origin',(8.43346325,7.49999999999998,2.10482457));
#153075=CARTESIAN_POINT('',(8.37982974945342,7.49999999999998,-2.03760383017956));
#153076=CARTESIAN_POINT('Origin',(2.22044604925031E-15,7.49999999999998,
2.22044604925031E-15));
#153077=CARTESIAN_POINT('Origin',(6.817832118,7.49999999999998,-5.391730155));
#153078=CARTESIAN_POINT('',(8.083776576,7.49999999999998,-3.004318937));
#153079=CARTESIAN_POINT('Origin',(8.667872637,7.49999999999998,0.649286377));
#153080=CARTESIAN_POINT('',(7.914936808,7.49999999999998,-3.424492856));
#153081=CARTESIAN_POINT('Origin',(2.22044604925031E-15,7.49999999999998,
2.22044604925031E-15));
#153082=CARTESIAN_POINT('Origin',(5.808556991,7.49999999999998,-6.466394246));
#153083=CARTESIAN_POINT('',(7.459766444,7.49999999999998,-4.327269416));
#153084=CARTESIAN_POINT('Origin',(8.65292311,7.49999999999998,-0.824930601999998));
#153085=CARTESIAN_POINT('',(7.222345546,7.49999999999998,-4.712865457));
#153086=CARTESIAN_POINT('Origin',(2.22044604925031E-15,7.49999999999998,
2.22044604925031E-15));
#153087=CARTESIAN_POINT('Origin',(4.632180254,7.49999999999998,-7.355031947));
#153088=CARTESIAN_POINT('',(6.621152413,7.49999999999998,-5.525732234));
#153089=CARTESIAN_POINT('Origin',(8.38904474,7.49999999999998,-2.275415831));
#153090=CARTESIAN_POINT('',(6.321980552,7.49999999999998,-5.8656575));
#153091=CARTESIAN_POINT('Origin',(2.22044604925031E-15,7.49999999999998,
2.22044604925031E-15));
#153092=CARTESIAN_POINT('Origin',(3.322544125,7.49999999999998,-8.032078771));
#153093=CARTESIAN_POINT('',(5.592059883,7.49999999999998,-6.565229795));
#153094=CARTESIAN_POINT('Origin',(7.883828827,7.49999999999998,-3.660441488));
#153095=CARTESIAN_POINT('',(5.239743687,7.49999999999998,-6.849705256));
#153096=CARTESIAN_POINT('Origin',(2.22044604925031E-15,7.49999999999998,
2.22044604925031E-15));
#153097=CARTESIAN_POINT('Origin',(1.917324452,7.49999999999998,-8.478057313));
#153098=CARTESIAN_POINT('',(4.402093972,7.49999999999998,-7.415857648));
#153099=CARTESIAN_POINT('Origin',(7.151809512,7.49999999999998,-4.940162908));
#153100=CARTESIAN_POINT('Origin',(2.22044604925031E-15,7.49999999999998,
2.22044604925031E-15));
#153101=CARTESIAN_POINT('',(3.08548783,7.49999999999998,-8.05314478));
#153102=CARTESIAN_POINT('Origin',(6.214045658,7.49999999999998,-6.077764837));
#153103=CARTESIAN_POINT('Origin',(2.22044604925031E-15,7.49999999999998,
2.22044604925031E-15));
#153104=CARTESIAN_POINT('',(1.680117823,7.49999999999998,-8.458757598));
#153105=CARTESIAN_POINT('Origin',(5.097515025,7.49999999999998,-7.040520536));
#153106=CARTESIAN_POINT('',(1.233803568,7.49999999999998,-8.535285863));
#153107=CARTESIAN_POINT('Origin',(2.22044604925031E-15,7.49999999999998,
2.22044604925031E-15));
#153108=CARTESIAN_POINT('',(0.978452338000002,7.49999999999998,-9.700779918));
#153109=CARTESIAN_POINT('Origin',(-2.460854379,7.49999999999998,-8.336533127));
#153110=CARTESIAN_POINT('',(0.675061572000001,7.49999999999998,-9.726602278));
#153111=CARTESIAN_POINT('Origin',(2.22044604925031E-15,7.49999999999998,
2.22044604925031E-15));
#153112=CARTESIAN_POINT('',(0.226413885000002,7.49999999999998,-8.621027361));
#153113=CARTESIAN_POINT('Origin',(3.834338166,7.49999999999998,-7.800733278));
#153114=CARTESIAN_POINT('',(-0.226413884999999,7.49999999999998,-8.621027361));
#153115=CARTESIAN_POINT('Origin',(2.22044604925031E-15,7.49999999999998,
2.22044604925031E-15));
#153116=CARTESIAN_POINT('Origin',(-3.834338166,7.49999999999998,-7.800733278));
#153117=CARTESIAN_POINT('',(-1.233803569,7.49999999999998,-8.535285862));
#153118=CARTESIAN_POINT('Origin',(2.460854379,7.49999999999998,-8.336533127));
#153119=CARTESIAN_POINT('',(-1.680117823,7.49999999999998,-8.458757598));
#153120=CARTESIAN_POINT('Origin',(2.22044604925031E-15,7.49999999999998,
2.22044604925031E-15));
#153121=CARTESIAN_POINT('Origin',(-5.097515025,7.49999999999998,-7.040520536));
#153122=CARTESIAN_POINT('',(-2.65852674,7.49999999999998,-8.20399973));
#153123=CARTESIAN_POINT('Origin',(1.016576292,7.49999999999998,-8.632506096));
#153124=CARTESIAN_POINT('',(-3.085487831,7.49999999999998,-8.05314478));
#153125=CARTESIAN_POINT('Origin',(2.22044604925031E-15,7.49999999999998,
2.22044604925031E-15));
#153126=CARTESIAN_POINT('Origin',(-6.214045658,7.49999999999998,-6.077764837));
#153127=CARTESIAN_POINT('',(-4.006768937,7.49999999999998,-7.636699463));
#153128=CARTESIAN_POINT('Origin',(-0.456946843999999,7.49999999999998,-8.680137582));
#153129=CARTESIAN_POINT('',(-4.402093971,7.49999999999998,-7.415857649));
#153130=CARTESIAN_POINT('Origin',(2.22044604925031E-15,7.49999999999998,
2.22044604925031E-15));
#153131=CARTESIAN_POINT('Origin',(-7.151809512,7.49999999999998,-4.940162908));
#153132=CARTESIAN_POINT('',(-5.239743688,7.49999999999998,-6.849705256));
#153133=CARTESIAN_POINT('Origin',(-1.917324452,7.49999999999998,-8.478057313));
#153134=CARTESIAN_POINT('',(-5.592059883,7.49999999999998,-6.565229795));
#153135=CARTESIAN_POINT('Origin',(2.22044604925031E-15,7.49999999999998,
2.22044604925031E-15));
#153136=CARTESIAN_POINT('Origin',(-7.883828827,7.49999999999998,-3.660441488));
#153137=CARTESIAN_POINT('',(-6.321980552,7.49999999999998,-5.8656575));
#153138=CARTESIAN_POINT('Origin',(-3.322544125,7.49999999999998,-8.032078771));
#153139=CARTESIAN_POINT('',(-6.621152413,7.49999999999998,-5.525732234));
#153140=CARTESIAN_POINT('Origin',(2.22044604925031E-15,7.49999999999998,
2.22044604925031E-15));
#153141=CARTESIAN_POINT('Origin',(-8.38904474,7.49999999999998,-2.275415831));
#153142=CARTESIAN_POINT('',(-7.222345546,7.49999999999998,-4.712865457));
#153143=CARTESIAN_POINT('Origin',(-4.632180254,7.49999999999998,-7.355031947));
#153144=CARTESIAN_POINT('',(-7.459766444,7.49999999999998,-4.327269417));
#153145=CARTESIAN_POINT('Origin',(2.22044604925031E-15,7.49999999999998,
2.22044604925031E-15));
#153146=CARTESIAN_POINT('Origin',(-8.65292311,7.49999999999998,-0.824930601999998));
#153147=CARTESIAN_POINT('',(-7.914936808,7.49999999999998,-3.424492856));
#153148=CARTESIAN_POINT('Origin',(-5.808556991,7.49999999999998,-6.466394246));
#153149=CARTESIAN_POINT('',(-8.083776576,7.49999999999998,-3.004318937));
#153150=CARTESIAN_POINT('Origin',(2.22044604925031E-15,7.49999999999998,
2.22044604925031E-15));
#153151=CARTESIAN_POINT('Origin',(-8.667872637,7.49999999999998,0.649286377));
#153152=CARTESIAN_POINT('',(-8.37982974917112,7.49999999999998,-2.03760383055369));
#153153=CARTESIAN_POINT('Origin',(-6.817832118,7.49999999999998,-5.391730155));
#153154=CARTESIAN_POINT('',(-8.475231174,7.49999999999998,-1.594939671));
#153155=CARTESIAN_POINT('Origin',(2.22044604925031E-15,7.49999999999998,
2.22044604925031E-15));
#153156=CARTESIAN_POINT('Origin',(-8.43346325,7.49999999999998,2.10482457));
#153157=CARTESIAN_POINT('',(-8.603650246,7.49999999999998,-0.592096651999998));
#153158=CARTESIAN_POINT('Origin',(-7.630970629,7.49999999999998,-4.161955804));
#153159=CARTESIAN_POINT('',(-8.622868801,7.49999999999998,-0.139676895));
#153160=CARTESIAN_POINT('Origin',(2.22044604925031E-15,7.49999999999998,
2.22044604925031E-15));
#153161=CARTESIAN_POINT('Origin',(-7.956438479,7.49999999999998,3.499810792));
#153162=CARTESIAN_POINT('',(-8.579959389,7.49999999999998,0.870444068000003));
#153163=CARTESIAN_POINT('Origin',(-8.224580008,7.49999999999998,-2.812449563));
#153164=CARTESIAN_POINT('',(-8.522442193,7.49999999999998,1.31960413));
#153165=CARTESIAN_POINT('Origin',(2.22044604925031E-15,7.49999999999998,
2.22044604925031E-15));
#153166=CARTESIAN_POINT('Origin',(-7.25052146,7.49999999999998,4.794113829));
#153167=CARTESIAN_POINT('',(-8.309438723,7.49999999999998,2.307943698));
#153168=CARTESIAN_POINT('Origin',(-8.581583195,7.49999999999998,-1.382034268));
#153169=CARTESIAN_POINT('',(-8.17684044,7.49999999999998,2.740922548));
#153170=CARTESIAN_POINT('Origin',(2.22044604925031E-15,7.49999999999998,
2.22044604925031E-15));
#153171=CARTESIAN_POINT('Origin',(-6.33602014,7.49999999999998,5.950498941));
#153172=CARTESIAN_POINT('',(-7.799870633,7.49999999999998,3.67904799));
#153173=CARTESIAN_POINT('Origin',(-8.691709858,7.49999999999998,0.088139637000002));
#153174=CARTESIAN_POINT('',(-7.596005875,7.49999999999998,4.083389615));
#153175=CARTESIAN_POINT('Origin',(2.22044604925031E-15,7.49999999999998,
2.22044604925031E-15));
#153176=CARTESIAN_POINT('Origin',(-5.239243055,7.49999999999998,6.935699032));
#153177=CARTESIAN_POINT('',(-7.065914466,7.49999999999998,4.944312768));
#153178=CARTESIAN_POINT('Origin',(-8.551791853,7.49999999999998,1.555777924));
#153179=CARTESIAN_POINT('',(-6.796648051,7.49999999999998,5.308384996));
#153180=CARTESIAN_POINT('Origin',(2.22044604925031E-15,7.49999999999998,
2.22044604925031E-15));
#153181=CARTESIAN_POINT('Origin',(-3.991742488,7.49999999999998,7.721371689));
#153182=CARTESIAN_POINT('',(-6.128684805,7.49999999999998,6.067338672));
#153183=CARTESIAN_POINT('Origin',(-8.165854367,7.49999999999998,2.978659314));
#153184=CARTESIAN_POINT('',(-5.801763037,7.49999999999998,6.380667807));
#153185=CARTESIAN_POINT('Origin',(2.22044604925031E-15,7.49999999999998,
2.22044604925031E-15));
#153186=CARTESIAN_POINT('Origin',(-2.629406756,7.49999999999998,8.284914542));
#153187=CARTESIAN_POINT('',(-5.015144041,7.49999999999998,7.015818288));
#153188=CARTESIAN_POINT('Origin',(-7.545000119,7.49999999999998,4.315850098));
#153189=CARTESIAN_POINT('',(-4.639971864,7.49999999999998,7.269390422));
#153190=CARTESIAN_POINT('Origin',(2.22044604925031E-15,7.49999999999998,
2.22044604925031E-15));
#153191=CARTESIAN_POINT('Origin',(-1.19142778,7.49999999999998,8.610115487));
#153192=CARTESIAN_POINT('',(-3.757326714,7.49999999999998,7.762465586));
#153193=CARTESIAN_POINT('Origin',(-6.707089953,7.49999999999998,5.528881732));
#153194=CARTESIAN_POINT('',(-3.344697148,7.49999999999998,7.948985909));
#153195=CARTESIAN_POINT('Origin',(2.22044604925031E-15,7.49999999999998,
2.22044604925031E-15));
#153196=CARTESIAN_POINT('Origin',(0.280826404000001,7.49999999999998,8.687619086));
#153197=CARTESIAN_POINT('',(-2.391417938,7.49999999999998,8.285800881));
#153198=CARTESIAN_POINT('Origin',(-5.676229022,7.49999999999998,6.582857506));
#153199=CARTESIAN_POINT('',(-1.953201585,7.49999999999998,8.399903545));
#153200=CARTESIAN_POINT('Origin',(2.22044604925031E-15,7.49999999999998,
2.22044604925031E-15));
#153201=CARTESIAN_POINT('Origin',(1.745001724,7.49999999999998,8.515195702));
#153202=CARTESIAN_POINT('',(-0.956712421999999,7.49999999999998,8.570768772));
#153203=CARTESIAN_POINT('Origin',(-4.482073316,7.49999999999998,7.447456454));
#153204=CARTESIAN_POINT('',(-0.505515968999999,7.49999999999998,8.60917125));
#153205=CARTESIAN_POINT('Origin',(2.22044604925031E-15,7.49999999999998,
2.22044604925031E-15));
#153206=CARTESIAN_POINT('Origin',(3.158976522,7.49999999999998,8.09780564));
#153207=CARTESIAN_POINT('',(0.505515969000001,7.49999999999998,8.60917125));
#153208=CARTESIAN_POINT('Origin',(-3.158976522,7.49999999999998,8.09780564));
#153209=CARTESIAN_POINT('',(0.956712422000002,7.49999999999998,8.570768772));
#153210=CARTESIAN_POINT('Origin',(2.22044604925031E-15,7.49999999999998,
2.22044604925031E-15));
#153211=CARTESIAN_POINT('Origin',(4.482073316,7.49999999999998,7.447456454));
#153212=CARTESIAN_POINT('',(2.391417938,7.49999999999998,8.285800881));
#153213=CARTESIAN_POINT('Origin',(2.22044604925031E-15,7.49999999999998,
2.22044604925031E-15));
#153214=CARTESIAN_POINT('Origin',(5.676229022,7.49999999999998,6.582857506));
#153215=CARTESIAN_POINT('',(3.757326714,7.49999999999998,7.762465586));
#153216=CARTESIAN_POINT('Origin',(2.22044604925031E-15,7.49999999999998,
2.22044604925031E-15));
#153217=CARTESIAN_POINT('Origin',(6.707089953,7.49999999999998,5.528881732));
#153218=CARTESIAN_POINT('',(4.639971864,7.49999999999998,7.269390422));
#153219=CARTESIAN_POINT('Origin',(1.19142778,7.49999999999998,8.610115487));
#153220=CARTESIAN_POINT('',(5.015144041,7.49999999999998,7.015818288));
#153221=CARTESIAN_POINT('Origin',(2.22044604925031E-15,7.49999999999998,
2.22044604925031E-15));
#153222=CARTESIAN_POINT('Origin',(7.545000119,7.49999999999998,4.315850098));
#153223=CARTESIAN_POINT('',(5.801763037,7.49999999999998,6.380667807));
#153224=CARTESIAN_POINT('Origin',(2.629406756,7.49999999999998,8.284914542));
#153225=CARTESIAN_POINT('',(6.128684805,7.49999999999998,6.067338672));
#153226=CARTESIAN_POINT('Origin',(2.22044604925031E-15,7.49999999999998,
2.22044604925031E-15));
#153227=CARTESIAN_POINT('Origin',(8.165854367,7.49999999999998,2.978659314));
#153228=CARTESIAN_POINT('',(6.796648051,7.49999999999998,5.308384996));
#153229=CARTESIAN_POINT('Origin',(3.991742488,7.49999999999998,7.721371689));
#153230=CARTESIAN_POINT('',(7.065914466,7.49999999999998,4.944312769));
#153231=CARTESIAN_POINT('Origin',(2.22044604925031E-15,7.49999999999998,
2.22044604925031E-15));
#153232=CARTESIAN_POINT('Origin',(8.551791853,7.49999999999998,1.555777924));
#153233=CARTESIAN_POINT('',(7.596005875,7.49999999999998,4.083389615));
#153234=CARTESIAN_POINT('Origin',(5.239243055,7.49999999999998,6.935699032));
#153235=CARTESIAN_POINT('',(7.799870633,7.49999999999998,3.679047989));
#153236=CARTESIAN_POINT('Origin',(2.22044604925031E-15,7.49999999999998,
2.22044604925031E-15));
#153237=CARTESIAN_POINT('Origin',(8.691709858,7.49999999999998,0.088139637000002));
#153238=CARTESIAN_POINT('',(8.17684044,7.49999999999998,2.740922548));
#153239=CARTESIAN_POINT('Origin',(6.33602014,7.49999999999998,5.950498941));
#153240=CARTESIAN_POINT('',(8.309438723,7.49999999999998,2.307943698));
#153241=CARTESIAN_POINT('Origin',(2.22044604925031E-15,7.49999999999998,
2.22044604925031E-15));
#153242=CARTESIAN_POINT('Origin',(8.581583195,7.49999999999998,-1.382034268));
#153243=CARTESIAN_POINT('',(8.522442193,7.49999999999998,1.31960413));
#153244=CARTESIAN_POINT('Origin',(7.25052146,7.49999999999998,4.794113829));
#153245=CARTESIAN_POINT('',(8.579959389,7.49999999999998,0.870444068000003));
#153246=CARTESIAN_POINT('Origin',(2.22044604925031E-15,7.49999999999998,
2.22044604925031E-15));
#153247=CARTESIAN_POINT('Origin',(8.224580008,7.49999999999998,-2.812449563));
#153248=CARTESIAN_POINT('',(8.622868801,7.49999999999998,-0.139676895));
#153249=CARTESIAN_POINT('Origin',(7.956438479,7.49999999999998,3.499810792));
#153250=CARTESIAN_POINT('Origin',(2.22044604925031E-15,7.49999999999998,
2.22044604925031E-15));
#153251=CARTESIAN_POINT('Origin',(2.22044604925031E-15,17.5,2.22044604925031E-15));
#153252=CARTESIAN_POINT('',(0.978452338000002,2.49999999999998,-9.700779918));
#153253=CARTESIAN_POINT('',(0.675061572000001,7.49999999999998,-9.726602278));
#153254=CARTESIAN_POINT('Origin',(-3.834338166,2.49999999999998,-7.800733278));
#153255=CARTESIAN_POINT('',(-0.226413884999999,2.49999999999998,-8.621027361));
#153256=CARTESIAN_POINT('Origin',(3.834338166,2.49999999999998,-7.800733278));
#153257=CARTESIAN_POINT('',(0.226413885000002,2.49999999999998,-8.621027361));
#153258=CARTESIAN_POINT('Origin',(2.22044604925031E-15,2.49999999999998,
2.22044604925031E-15));
#153259=CARTESIAN_POINT('Origin',(-2.460854379,2.49999999999998,-8.336533127));
#153260=CARTESIAN_POINT('',(1.233803568,2.49999999999998,-8.535285863));
#153261=CARTESIAN_POINT('Origin',(5.097515025,2.49999999999998,-7.040520536));
#153262=CARTESIAN_POINT('',(1.680117823,2.49999999999998,-8.458757598));
#153263=CARTESIAN_POINT('Origin',(2.22044604925031E-15,2.49999999999998,
2.22044604925031E-15));
#153264=CARTESIAN_POINT('Origin',(-7.956438479,2.49999999999998,3.499810792));
#153265=CARTESIAN_POINT('',(-8.622868801,2.49999999999998,-0.139676895));
#153266=CARTESIAN_POINT('Origin',(-7.630970629,2.49999999999998,-4.161955804));
#153267=CARTESIAN_POINT('',(-8.603650246,2.49999999999998,-0.592096651999998));
#153268=CARTESIAN_POINT('Origin',(2.22044604925031E-15,2.49999999999998,
2.22044604925031E-15));
#153269=CARTESIAN_POINT('Origin',(-8.43346325,2.49999999999998,2.10482457));
#153270=CARTESIAN_POINT('',(-8.475231174,2.49999999999998,-1.594939671));
#153271=CARTESIAN_POINT('Origin',(-6.817832118,2.49999999999998,-5.391730155));
#153272=CARTESIAN_POINT('',(-8.379829749,2.49999999999998,-2.03760383));
#153273=CARTESIAN_POINT('Origin',(2.22044604925031E-15,2.49999999999998,
2.22044604925031E-15));
#153274=CARTESIAN_POINT('Origin',(-8.667872637,2.49999999999998,0.649286377));
#153275=CARTESIAN_POINT('',(-8.083776576,2.49999999999998,-3.004318937));
#153276=CARTESIAN_POINT('Origin',(-5.808556991,2.49999999999998,-6.466394246));
#153277=CARTESIAN_POINT('',(-7.914936808,2.49999999999998,-3.424492856));
#153278=CARTESIAN_POINT('Origin',(2.22044604925031E-15,2.49999999999998,
2.22044604925031E-15));
#153279=CARTESIAN_POINT('Origin',(-8.65292311,2.49999999999998,-0.824930601999998));
#153280=CARTESIAN_POINT('',(-7.459766444,2.49999999999998,-4.327269417));
#153281=CARTESIAN_POINT('Origin',(-4.632180254,2.49999999999998,-7.355031947));
#153282=CARTESIAN_POINT('',(-7.222345546,2.49999999999998,-4.712865457));
#153283=CARTESIAN_POINT('Origin',(2.22044604925031E-15,2.49999999999998,
2.22044604925031E-15));
#153284=CARTESIAN_POINT('Origin',(-5.097515025,2.49999999999998,-7.040520536));
#153285=CARTESIAN_POINT('',(-1.680117823,2.49999999999998,-8.458757598));
#153286=CARTESIAN_POINT('Origin',(2.460854379,2.49999999999998,-8.336533127));
#153287=CARTESIAN_POINT('',(-1.233803569,2.49999999999998,-8.535285862));
#153288=CARTESIAN_POINT('Origin',(2.22044604925031E-15,2.49999999999998,
2.22044604925031E-15));
#153289=CARTESIAN_POINT('Origin',(-6.214045658,2.49999999999998,-6.077764837));
#153290=CARTESIAN_POINT('',(-3.085487831,2.49999999999998,-8.05314478));
#153291=CARTESIAN_POINT('Origin',(1.016576292,2.49999999999998,-8.632506096));
#153292=CARTESIAN_POINT('',(-2.65852674,2.49999999999998,-8.20399973));
#153293=CARTESIAN_POINT('Origin',(2.22044604925031E-15,2.49999999999998,
2.22044604925031E-15));
#153294=CARTESIAN_POINT('Origin',(-7.151809512,2.49999999999998,-4.940162908));
#153295=CARTESIAN_POINT('',(-4.402093971,2.49999999999998,-7.415857649));
#153296=CARTESIAN_POINT('Origin',(-0.456946843999999,2.49999999999998,-8.680137582));
#153297=CARTESIAN_POINT('',(-4.006768937,2.49999999999998,-7.636699463));
#153298=CARTESIAN_POINT('Origin',(2.22044604925031E-15,2.49999999999998,
2.22044604925031E-15));
#153299=CARTESIAN_POINT('Origin',(-8.38904474,2.49999999999998,-2.275415831));
#153300=CARTESIAN_POINT('',(-6.621152413,2.49999999999998,-5.525732234));
#153301=CARTESIAN_POINT('Origin',(-3.322544125,2.49999999999998,-8.032078771));
#153302=CARTESIAN_POINT('',(-6.321980552,2.49999999999998,-5.8656575));
#153303=CARTESIAN_POINT('Origin',(2.22044604925031E-15,2.49999999999998,
2.22044604925031E-15));
#153304=CARTESIAN_POINT('Origin',(-7.883828827,2.49999999999998,-3.660441488));
#153305=CARTESIAN_POINT('',(-5.592059883,2.49999999999998,-6.565229795));
#153306=CARTESIAN_POINT('Origin',(-1.917324452,2.49999999999998,-8.478057313));
#153307=CARTESIAN_POINT('',(-5.239743688,2.49999999999998,-6.849705256));
#153308=CARTESIAN_POINT('Origin',(2.22044604925031E-15,2.49999999999998,
2.22044604925031E-15));
#153309=CARTESIAN_POINT('Origin',(3.158976522,2.49999999999998,8.09780564));
#153310=CARTESIAN_POINT('',(-0.505515968999999,2.49999999999998,8.60917125));
#153311=CARTESIAN_POINT('Origin',(-4.482073316,2.49999999999998,7.447456454));
#153312=CARTESIAN_POINT('',(-0.956712421999999,2.49999999999998,8.570768772));
#153313=CARTESIAN_POINT('Origin',(2.22044604925031E-15,2.49999999999998,
2.22044604925031E-15));
#153314=CARTESIAN_POINT('Origin',(1.745001724,2.49999999999998,8.515195702));
#153315=CARTESIAN_POINT('',(-1.953201585,2.49999999999998,8.399903545));
#153316=CARTESIAN_POINT('Origin',(-5.676229022,2.49999999999998,6.582857506));
#153317=CARTESIAN_POINT('',(-2.391417938,2.49999999999998,8.285800881));
#153318=CARTESIAN_POINT('Origin',(2.22044604925031E-15,2.49999999999998,
2.22044604925031E-15));
#153319=CARTESIAN_POINT('Origin',(-1.19142778,2.49999999999998,8.610115487));
#153320=CARTESIAN_POINT('',(-4.639971864,2.49999999999998,7.269390422));
#153321=CARTESIAN_POINT('Origin',(-7.545000119,2.49999999999998,4.315850098));
#153322=CARTESIAN_POINT('',(-5.015144041,2.49999999999998,7.015818288));
#153323=CARTESIAN_POINT('Origin',(2.22044604925031E-15,2.49999999999998,
2.22044604925031E-15));
#153324=CARTESIAN_POINT('Origin',(0.280826404000001,2.49999999999998,8.687619086));
#153325=CARTESIAN_POINT('',(-3.344697148,2.49999999999998,7.948985909));
#153326=CARTESIAN_POINT('Origin',(-6.707089953,2.49999999999998,5.528881732));
#153327=CARTESIAN_POINT('',(-3.757326714,2.49999999999998,7.762465586));
#153328=CARTESIAN_POINT('Origin',(2.22044604925031E-15,2.49999999999998,
2.22044604925031E-15));
#153329=CARTESIAN_POINT('Origin',(-7.25052146,2.49999999999998,4.794113829));
#153330=CARTESIAN_POINT('',(-8.522442193,2.49999999999998,1.31960413));
#153331=CARTESIAN_POINT('Origin',(-8.224580008,2.49999999999998,-2.812449563));
#153332=CARTESIAN_POINT('',(-8.579959389,2.49999999999998,0.870444068000003));
#153333=CARTESIAN_POINT('Origin',(2.22044604925031E-15,2.49999999999998,
2.22044604925031E-15));
#153334=CARTESIAN_POINT('Origin',(-6.33602014,2.49999999999998,5.950498941));
#153335=CARTESIAN_POINT('',(-8.17684044,2.49999999999998,2.740922548));
#153336=CARTESIAN_POINT('Origin',(-8.581583195,2.49999999999998,-1.382034268));
#153337=CARTESIAN_POINT('',(-8.309438723,2.49999999999998,2.307943698));
#153338=CARTESIAN_POINT('Origin',(2.22044604925031E-15,2.49999999999998,
2.22044604925031E-15));
#153339=CARTESIAN_POINT('Origin',(-5.239243055,2.49999999999998,6.935699032));
#153340=CARTESIAN_POINT('',(-7.596005875,2.49999999999998,4.083389615));
#153341=CARTESIAN_POINT('Origin',(-8.691709858,2.49999999999998,0.088139637000002));
#153342=CARTESIAN_POINT('',(-7.799870633,2.49999999999998,3.67904799));
#153343=CARTESIAN_POINT('Origin',(2.22044604925031E-15,2.49999999999998,
2.22044604925031E-15));
#153344=CARTESIAN_POINT('Origin',(-2.629406756,2.49999999999998,8.284914542));
#153345=CARTESIAN_POINT('',(-5.801763037,2.49999999999998,6.380667807));
#153346=CARTESIAN_POINT('Origin',(-8.165854367,2.49999999999998,2.978659314));
#153347=CARTESIAN_POINT('',(-6.128684805,2.49999999999998,6.067338672));
#153348=CARTESIAN_POINT('Origin',(2.22044604925031E-15,2.49999999999998,
2.22044604925031E-15));
#153349=CARTESIAN_POINT('Origin',(-3.991742488,2.49999999999998,7.721371689));
#153350=CARTESIAN_POINT('',(-6.796648051,2.49999999999998,5.308384996));
#153351=CARTESIAN_POINT('Origin',(-8.551791853,2.49999999999998,1.555777924));
#153352=CARTESIAN_POINT('',(-7.065914466,2.49999999999998,4.944312768));
#153353=CARTESIAN_POINT('Origin',(2.22044604925031E-15,2.49999999999998,
2.22044604925031E-15));
#153354=CARTESIAN_POINT('Origin',(8.224580008,2.49999999999998,-2.812449563));
#153355=CARTESIAN_POINT('',(8.579959389,2.49999999999998,0.870444068000003));
#153356=CARTESIAN_POINT('Origin',(7.25052146,2.49999999999998,4.794113829));
#153357=CARTESIAN_POINT('',(8.522442193,2.49999999999998,1.31960413));
#153358=CARTESIAN_POINT('Origin',(2.22044604925031E-15,2.49999999999998,
2.22044604925031E-15));
#153359=CARTESIAN_POINT('Origin',(8.581583195,2.49999999999998,-1.382034268));
#153360=CARTESIAN_POINT('',(8.309438723,2.49999999999998,2.307943698));
#153361=CARTESIAN_POINT('Origin',(6.33602014,2.49999999999998,5.950498941));
#153362=CARTESIAN_POINT('',(8.17684044,2.49999999999998,2.740922548));
#153363=CARTESIAN_POINT('Origin',(2.22044604925031E-15,2.49999999999998,
2.22044604925031E-15));
#153364=CARTESIAN_POINT('Origin',(8.551791853,2.49999999999998,1.555777924));
#153365=CARTESIAN_POINT('',(7.065914466,2.49999999999998,4.944312769));
#153366=CARTESIAN_POINT('Origin',(3.991742488,2.49999999999998,7.721371689));
#153367=CARTESIAN_POINT('',(6.796648051,2.49999999999998,5.308384996));
#153368=CARTESIAN_POINT('Origin',(2.22044604925031E-15,2.49999999999998,
2.22044604925031E-15));
#153369=CARTESIAN_POINT('Origin',(8.691709858,2.49999999999998,0.088139637000002));
#153370=CARTESIAN_POINT('',(7.799870633,2.49999999999998,3.679047989));
#153371=CARTESIAN_POINT('Origin',(5.239243055,2.49999999999998,6.935699032));
#153372=CARTESIAN_POINT('',(7.596005875,2.49999999999998,4.083389615));
#153373=CARTESIAN_POINT('Origin',(2.22044604925031E-15,2.49999999999998,
2.22044604925031E-15));
#153374=CARTESIAN_POINT('Origin',(4.482073316,2.49999999999998,7.447456454));
#153375=CARTESIAN_POINT('',(0.956712422000002,2.49999999999998,8.570768772));
#153376=CARTESIAN_POINT('Origin',(-3.158976522,2.49999999999998,8.09780564));
#153377=CARTESIAN_POINT('',(0.505515969000001,2.49999999999998,8.60917125));
#153378=CARTESIAN_POINT('Origin',(2.22044604925031E-15,2.49999999999998,
2.22044604925031E-15));
#153379=CARTESIAN_POINT('Origin',(5.676229022,2.49999999999998,6.582857506));
#153380=CARTESIAN_POINT('',(2.391417938,2.49999999999998,8.285800881));
#153381=CARTESIAN_POINT('Origin',(2.22044604925031E-15,2.49999999999998,
2.22044604925031E-15));
#153382=CARTESIAN_POINT('Origin',(6.707089953,2.49999999999998,5.528881732));
#153383=CARTESIAN_POINT('',(3.757326714,2.49999999999998,7.762465586));
#153384=CARTESIAN_POINT('Origin',(2.22044604925031E-15,2.49999999999998,
2.22044604925031E-15));
#153385=CARTESIAN_POINT('Origin',(8.165854367,2.49999999999998,2.978659314));
#153386=CARTESIAN_POINT('',(6.128684805,2.49999999999998,6.067338672));
#153387=CARTESIAN_POINT('Origin',(2.629406756,2.49999999999998,8.284914542));
#153388=CARTESIAN_POINT('',(5.801763037,2.49999999999998,6.380667807));
#153389=CARTESIAN_POINT('Origin',(2.22044604925031E-15,2.49999999999998,
2.22044604925031E-15));
#153390=CARTESIAN_POINT('Origin',(7.545000119,2.49999999999998,4.315850098));
#153391=CARTESIAN_POINT('',(5.015144041,2.49999999999998,7.015818288));
#153392=CARTESIAN_POINT('Origin',(1.19142778,2.49999999999998,8.610115487));
#153393=CARTESIAN_POINT('',(4.639971864,2.49999999999998,7.269390422));
#153394=CARTESIAN_POINT('Origin',(2.22044604925031E-15,2.49999999999998,
2.22044604925031E-15));
#153395=CARTESIAN_POINT('Origin',(1.917324452,2.49999999999998,-8.478057313));
#153396=CARTESIAN_POINT('',(5.239743687,2.49999999999998,-6.849705256));
#153397=CARTESIAN_POINT('Origin',(7.883828827,2.49999999999998,-3.660441488));
#153398=CARTESIAN_POINT('',(5.592059883,2.49999999999998,-6.565229795));
#153399=CARTESIAN_POINT('Origin',(2.22044604925031E-15,2.49999999999998,
2.22044604925031E-15));
#153400=CARTESIAN_POINT('Origin',(3.322544125,2.49999999999998,-8.032078771));
#153401=CARTESIAN_POINT('',(6.321980552,2.49999999999998,-5.8656575));
#153402=CARTESIAN_POINT('Origin',(8.38904474,2.49999999999998,-2.275415831));
#153403=CARTESIAN_POINT('',(6.621152413,2.49999999999998,-5.525732234));
#153404=CARTESIAN_POINT('Origin',(2.22044604925031E-15,2.49999999999998,
2.22044604925031E-15));
#153405=CARTESIAN_POINT('Origin',(7.151809512,2.49999999999998,-4.940162908));
#153406=CARTESIAN_POINT('',(4.402093972,2.49999999999998,-7.415857648));
#153407=CARTESIAN_POINT('Origin',(2.22044604925031E-15,2.49999999999998,
2.22044604925031E-15));
#153408=CARTESIAN_POINT('Origin',(6.214045658,2.49999999999998,-6.077764837));
#153409=CARTESIAN_POINT('',(3.085487831,2.49999999999998,-8.05314478));
#153410=CARTESIAN_POINT('Origin',(2.22044604925031E-15,2.49999999999998,
2.22044604925031E-15));
#153411=CARTESIAN_POINT('Origin',(4.632180254,2.49999999999998,-7.355031947));
#153412=CARTESIAN_POINT('',(7.222345546,2.49999999999998,-4.712865457));
#153413=CARTESIAN_POINT('Origin',(8.65292311,2.49999999999998,-0.824930601999998));
#153414=CARTESIAN_POINT('',(7.459766444,2.49999999999998,-4.327269416));
#153415=CARTESIAN_POINT('Origin',(2.22044604925031E-15,2.49999999999998,
2.22044604925031E-15));
#153416=CARTESIAN_POINT('Origin',(5.808556991,2.49999999999998,-6.466394246));
#153417=CARTESIAN_POINT('',(7.914936808,2.49999999999998,-3.424492856));
#153418=CARTESIAN_POINT('Origin',(8.667872637,2.49999999999998,0.649286377));
#153419=CARTESIAN_POINT('',(8.083776576,2.49999999999998,-3.004318937));
#153420=CARTESIAN_POINT('Origin',(2.22044604925031E-15,2.49999999999998,
2.22044604925031E-15));
#153421=CARTESIAN_POINT('Origin',(6.817832118,2.49999999999998,-5.391730155));
#153422=CARTESIAN_POINT('',(8.37982975,2.49999999999998,-2.03760383));
#153423=CARTESIAN_POINT('Origin',(8.43346325,2.49999999999998,2.10482457));
#153424=CARTESIAN_POINT('',(8.475231174,2.49999999999998,-1.594939671));
#153425=CARTESIAN_POINT('Origin',(2.22044604925031E-15,2.49999999999998,
2.22044604925031E-15));
#153426=CARTESIAN_POINT('Origin',(7.630970629,2.49999999999998,-4.161955804));
#153427=CARTESIAN_POINT('',(8.603650246,2.49999999999998,-0.592096652999998));
#153428=CARTESIAN_POINT('Origin',(7.956438479,2.49999999999998,3.499810792));
#153429=CARTESIAN_POINT('',(8.622868801,2.49999999999998,-0.139676895));
#153430=CARTESIAN_POINT('Origin',(2.22044604925031E-15,2.49999999999998,
2.22044604925031E-15));
#153431=CARTESIAN_POINT('Origin',(2.22044604925031E-15,7.70005079999998,
2.22044604925031E-15));
#153432=CARTESIAN_POINT('Origin',(2.22044604925031E-15,-1.30000000000002,
2.22044604925031E-15));
#153433=CARTESIAN_POINT('Origin',(2.22044604925031E-15,-1.30000000000002,
2.22044604925031E-15));
#153434=CARTESIAN_POINT('Origin',(2.22044604925031E-15,5.19999999999998,
2.22044604925031E-15));
#153435=CARTESIAN_POINT('Origin',(-5.077182071,4.99999999999998,-1.795054936));
#153436=CARTESIAN_POINT('',(-5.077182071,4.99999999999998,-1.795054936));
#153437=CARTESIAN_POINT('',(-5.07718207126124,2.69999999999998,-1.7950549352611));
#153438=CARTESIAN_POINT('',(-5.077182071,4.99999999999998,-1.795054936));
#153439=CARTESIAN_POINT('',(-5.077182071,2.69999999999998,-1.795054936));
#153440=CARTESIAN_POINT('',(-6.4,4.99999999999998,-2.262741699));
#153441=CARTESIAN_POINT('Origin',(-4.943848737,4.99999999999998,-2.172178552));
#153442=CARTESIAN_POINT('',(-4.57763771968452,4.99999999999998,-2.0112764371543));
#153443=CARTESIAN_POINT('',(-4.57763772,2.69999999999998,-2.011276437));
#153444=CARTESIAN_POINT('',(-4.57763772,4.99999999999998,-2.011276437));
#153445=CARTESIAN_POINT('Origin',(-4.943848737,2.69999999999998,-2.172178552));
#153446=CARTESIAN_POINT('Origin',(-4.943848737,4.99999999999998,-2.172178552));
#153447=CARTESIAN_POINT('Origin',(2.22044604925031E-15,4.99999999999998,
2.22044604925031E-15));
#153448=CARTESIAN_POINT('',(4.57763772,4.99999999999998,-2.011276437));
#153449=CARTESIAN_POINT('',(4.57763772,2.69999999999998,-2.011276437));
#153450=CARTESIAN_POINT('',(4.57763772,4.99999999999998,-2.011276437));
#153451=CARTESIAN_POINT('Origin',(2.22044604925031E-15,2.69999999999998,
2.22044604925031E-15));
#153452=CARTESIAN_POINT('Origin',(2.22044604925031E-15,4.99999999999998,
2.22044604925031E-15));
#153453=CARTESIAN_POINT('Origin',(4.943848737,4.99999999999998,-2.172178552));
#153454=CARTESIAN_POINT('',(5.07718207041197,4.99999999999998,-1.79505493577758));
#153455=CARTESIAN_POINT('',(5.07718207057322,2.69999999999998,-1.79505493573434));
#153456=CARTESIAN_POINT('',(5.077182071,4.99999999999998,-1.795054936));
#153457=CARTESIAN_POINT('Origin',(4.943848737,2.69999999999998,-2.172178552));
#153458=CARTESIAN_POINT('Origin',(4.943848737,4.99999999999998,-2.172178552));
#153459=CARTESIAN_POINT('Origin',(6.4,4.99999999999998,-2.2627417));
#153460=CARTESIAN_POINT('',(6.4,4.99999999999998,-2.2627417));
#153461=CARTESIAN_POINT('',(6.4,4.99999999999998,-2.2627417));
#153462=CARTESIAN_POINT('',(6.4,2.69999999999998,-2.2627417));
#153463=CARTESIAN_POINT('',(5.07718207,4.99999999999998,-1.795054936));
#153464=CARTESIAN_POINT('Origin',(6.266666667,4.99999999999998,-2.639865316));
#153465=CARTESIAN_POINT('',(6.63529411796585,4.99999999999998,-2.79515151131894));
#153466=CARTESIAN_POINT('',(6.635294118,4.99999999999998,-2.795151512));
#153467=CARTESIAN_POINT('Origin',(6.266666667,4.99999999999998,-2.639865316));
#153468=CARTESIAN_POINT('Origin',(2.22044604925031E-15,4.99999999999998,
2.22044604925031E-15));
#153469=CARTESIAN_POINT('Origin',(2.22044604925031E-15,2.69999999999998,
2.22044604925031E-15));
#153470=CARTESIAN_POINT('Origin',(2.22044604925031E-15,4.99999999999998,
2.22044604925031E-15));
#153471=CARTESIAN_POINT('Origin',(-6.266666667,4.99999999999998,-2.639865316));
#153472=CARTESIAN_POINT('Origin',(-4.943848737,4.99999999999998,2.172178552));
#153473=CARTESIAN_POINT('',(-5.077182071,4.99999999999998,1.795054936));
#153474=CARTESIAN_POINT('',(-5.077182071,2.69999999999998,1.795054935));
#153475=CARTESIAN_POINT('',(-5.077182071,4.99999999999998,1.795054936));
#153476=CARTESIAN_POINT('',(-4.57763772,2.69999999999998,2.011276437));
#153477=CARTESIAN_POINT('Origin',(-4.943848737,2.69999999999998,2.172178552));
#153478=CARTESIAN_POINT('',(-4.57763772,4.99999999999998,2.011276437));
#153479=CARTESIAN_POINT('',(-4.57763772,4.99999999999998,2.011276437));
#153480=CARTESIAN_POINT('Origin',(-4.943848737,4.99999999999998,2.172178552));
#153481=CARTESIAN_POINT('Origin',(-5.077182071,4.99999999999998,1.795054936));
#153482=CARTESIAN_POINT('',(-6.4,2.69999999999998,2.262741699));
#153483=CARTESIAN_POINT('',(-5.077182071,4.99999999999998,1.795054936));
#153484=CARTESIAN_POINT('Origin',(2.22044604925031E-15,4.99999999999998,
2.22044604925031E-15));
#153485=CARTESIAN_POINT('',(6.63529411796585,4.99999999999998,2.79515151131895));
#153486=CARTESIAN_POINT('',(6.635294118,4.99999999999998,2.795151512));
#153487=CARTESIAN_POINT('Origin',(2.22044604925031E-15,2.69999999999998,
2.22044604925031E-15));
#153488=CARTESIAN_POINT('Origin',(2.22044604925031E-15,4.99999999999998,
2.22044604925031E-15));
#153489=CARTESIAN_POINT('Origin',(6.266666667,4.99999999999998,2.639865316));
#153490=CARTESIAN_POINT('',(6.40000000007864,4.99999999999998,2.26274169944424));
#153491=CARTESIAN_POINT('',(6.4,4.99999999999998,2.262741699));
#153492=CARTESIAN_POINT('Origin',(6.266666667,4.99999999999998,2.639865316));
#153493=CARTESIAN_POINT('Origin',(6.4,4.99999999999998,2.2627417));
#153494=CARTESIAN_POINT('',(5.07718207037154,4.99999999999998,1.79505493622526));
#153495=CARTESIAN_POINT('',(5.077182071,2.69999999999998,1.795054935));
#153496=CARTESIAN_POINT('',(5.077182071,4.99999999999998,1.795054937));
#153497=CARTESIAN_POINT('',(5.07718207,2.69999999999998,1.795054936));
#153498=CARTESIAN_POINT('',(6.4,4.99999999999998,2.2627417));
#153499=CARTESIAN_POINT('Origin',(4.943848737,4.99999999999998,2.172178552));
#153500=CARTESIAN_POINT('',(4.57763771968453,4.99999999999998,2.0112764371543));
#153501=CARTESIAN_POINT('',(4.57763772,2.69999999999998,2.011276437));
#153502=CARTESIAN_POINT('',(4.57763772,4.99999999999998,2.011276437));
#153503=CARTESIAN_POINT('Origin',(4.943848737,2.69999999999998,2.172178552));
#153504=CARTESIAN_POINT('Origin',(4.943848737,4.99999999999998,2.172178552));
#153505=CARTESIAN_POINT('Origin',(2.22044604925031E-15,4.99999999999998,
2.22044604925031E-15));
#153506=CARTESIAN_POINT('Origin',(2.22044604925031E-15,2.69999999999998,
2.22044604925031E-15));
#153507=CARTESIAN_POINT('Origin',(2.22044604925031E-15,4.99999999999998,
2.22044604925031E-15));
#153508=CARTESIAN_POINT('Origin',(-4.943848737,4.99999999999998,2.172178552));
#153509=CARTESIAN_POINT('Origin',(-6.266666667,2.69999999999998,-2.639865316));
#153510=CARTESIAN_POINT('Origin',(-6.819607843,2.69999999999998,-2.872794609));
#153511=CARTESIAN_POINT('Origin',(-6.466666668,2.69999999999998,-2.074179889));
#153512=CARTESIAN_POINT('Origin',(-0.0666666669999971,2.69999999999998,
0.188561808000001));
#153513=CARTESIAN_POINT('Origin',(-5.143848737,2.69999999999998,-1.606493127));
#153514=CARTESIAN_POINT('Origin',(2.22044604925031E-15,2.69999999999998,
2.22044604925031E-15));
#153515=CARTESIAN_POINT('Origin',(-4.943848737,2.69999999999998,-2.172178552));
#153516=CARTESIAN_POINT('Origin',(-4.394532211,2.69999999999998,-1.93082538));
#153517=CARTESIAN_POINT('Origin',(2.22044604925031E-15,2.69999999999998,
2.22044604925031E-15));
#153518=CARTESIAN_POINT('Origin',(4.394532211,2.69999999999998,-1.93082538));
#153519=CARTESIAN_POINT('Origin',(0.0666666670000016,2.69999999999998,0.188561808000001));
#153520=CARTESIAN_POINT('Origin',(5.143848738,2.69999999999998,-1.606493127));
#153521=CARTESIAN_POINT('Origin',(4.943848737,2.69999999999998,-2.172178552));
#153522=CARTESIAN_POINT('Origin',(4.943848737,2.69999999999998,2.172178552));
#153523=CARTESIAN_POINT('Origin',(5.143848738,2.69999999999998,1.606493125));
#153524=CARTESIAN_POINT('Origin',(4.394532211,2.69999999999998,1.93082538));
#153525=CARTESIAN_POINT('Origin',(2.22044604925031E-15,2.69999999999998,
2.22044604925031E-15));
#153526=CARTESIAN_POINT('Origin',(-4.394532211,2.69999999999998,1.93082538));
#153527=CARTESIAN_POINT('Origin',(0.0666666670000016,2.69999999999998,-0.188561808000001));
#153528=CARTESIAN_POINT('Origin',(-4.943848737,2.69999999999998,2.172178552));
#153529=CARTESIAN_POINT('Origin',(-5.143848738,2.69999999999998,1.606493125));
#153530=CARTESIAN_POINT('Origin',(-0.0666666669999971,2.69999999999998,
-0.188561808000001));
#153531=CARTESIAN_POINT('Origin',(-6.466666667,2.69999999999998,2.074179891));
#153532=CARTESIAN_POINT('Origin',(2.22044604925031E-15,2.69999999999998,
2.22044604925031E-15));
#153533=CARTESIAN_POINT('Origin',(-6.819607843,2.69999999999998,2.87279461));
#153534=CARTESIAN_POINT('Origin',(-6.266666667,2.69999999999998,2.639865316));
#153535=CARTESIAN_POINT('Origin',(6.,4.49999999999998,2.22044604925031E-15));
#153536=CARTESIAN_POINT('Origin',(-6.,4.49999999999998,2.22044604925031E-15));
#459199=UNCERTAINTY_MEASURE_WITH_UNIT(LENGTH_MEASURE(0.01),#459243,
'DISTANCE_ACCURACY_VALUE',
'Maximum model space distance between geometric entities at asserted c
onnectivities');
#459216=UNCERTAINTY_MEASURE_WITH_UNIT(LENGTH_MEASURE(0.01),#459243,
'DISTANCE_ACCURACY_VALUE',
'Maximum model space distance between geometric entities at asserted c
onnectivities');
#459225=(
GEOMETRIC_REPRESENTATION_CONTEXT(3)
GLOBAL_UNCERTAINTY_ASSIGNED_CONTEXT((#459199))
GLOBAL_UNIT_ASSIGNED_CONTEXT((#459243,#459245,#459246))
REPRESENTATION_CONTEXT('','3D')
);
#459242=(
GEOMETRIC_REPRESENTATION_CONTEXT(3)
GLOBAL_UNCERTAINTY_ASSIGNED_CONTEXT((#459216))
GLOBAL_UNIT_ASSIGNED_CONTEXT((#459243,#459245,#459246))
REPRESENTATION_CONTEXT('','3D')
);
#459243=(
LENGTH_UNIT()
NAMED_UNIT(*)
SI_UNIT(.MILLI.,.METRE.)
);
#459245=(
NAMED_UNIT(*)
PLANE_ANGLE_UNIT()
SI_UNIT($,.RADIAN.)
);
#459246=(
NAMED_UNIT(*)
SI_UNIT($,.STERADIAN.)
SOLID_ANGLE_UNIT()
);
#459255=SHAPE_DEFINITION_REPRESENTATION(#459280,#459336);
#459280=PRODUCT_DEFINITION_SHAPE('',$,#459362);
#459336=SHAPE_REPRESENTATION('',(#97243),#459225);
#459353=PRODUCT_DEFINITION_CONTEXT('part definition',#459430,'design');
#459362=PRODUCT_DEFINITION('Filament Drive Gear','Filament Drive Gear',
#459387,#459353);
#459387=PRODUCT_DEFINITION_FORMATION('',$,#459440);
#459430=APPLICATION_CONTEXT(
'Core Data for Automotive Mechanical Design Process');
#459431=PRODUCT_CONTEXT('part definition',#459430,'mechanical');
#459440=PRODUCT('Filament Drive Gear','Filament Drive Gear',$,(#459431));
#459506=COLOUR_RGB('Light Blue',0.38,0.62,0.78);
#459507=FILL_AREA_STYLE_COLOUR('',#459506);
#459508=FILL_AREA_STYLE('',(#459507));
#459509=SURFACE_STYLE_FILL_AREA(#459508);
#459510=SURFACE_SIDE_STYLE('',(#459509));
#459511=SURFACE_STYLE_USAGE(.BOTH.,#459510);
#459512=PRESENTATION_STYLE_ASSIGNMENT((#459511));
ENDSEC;
END-ISO-10303-21;
